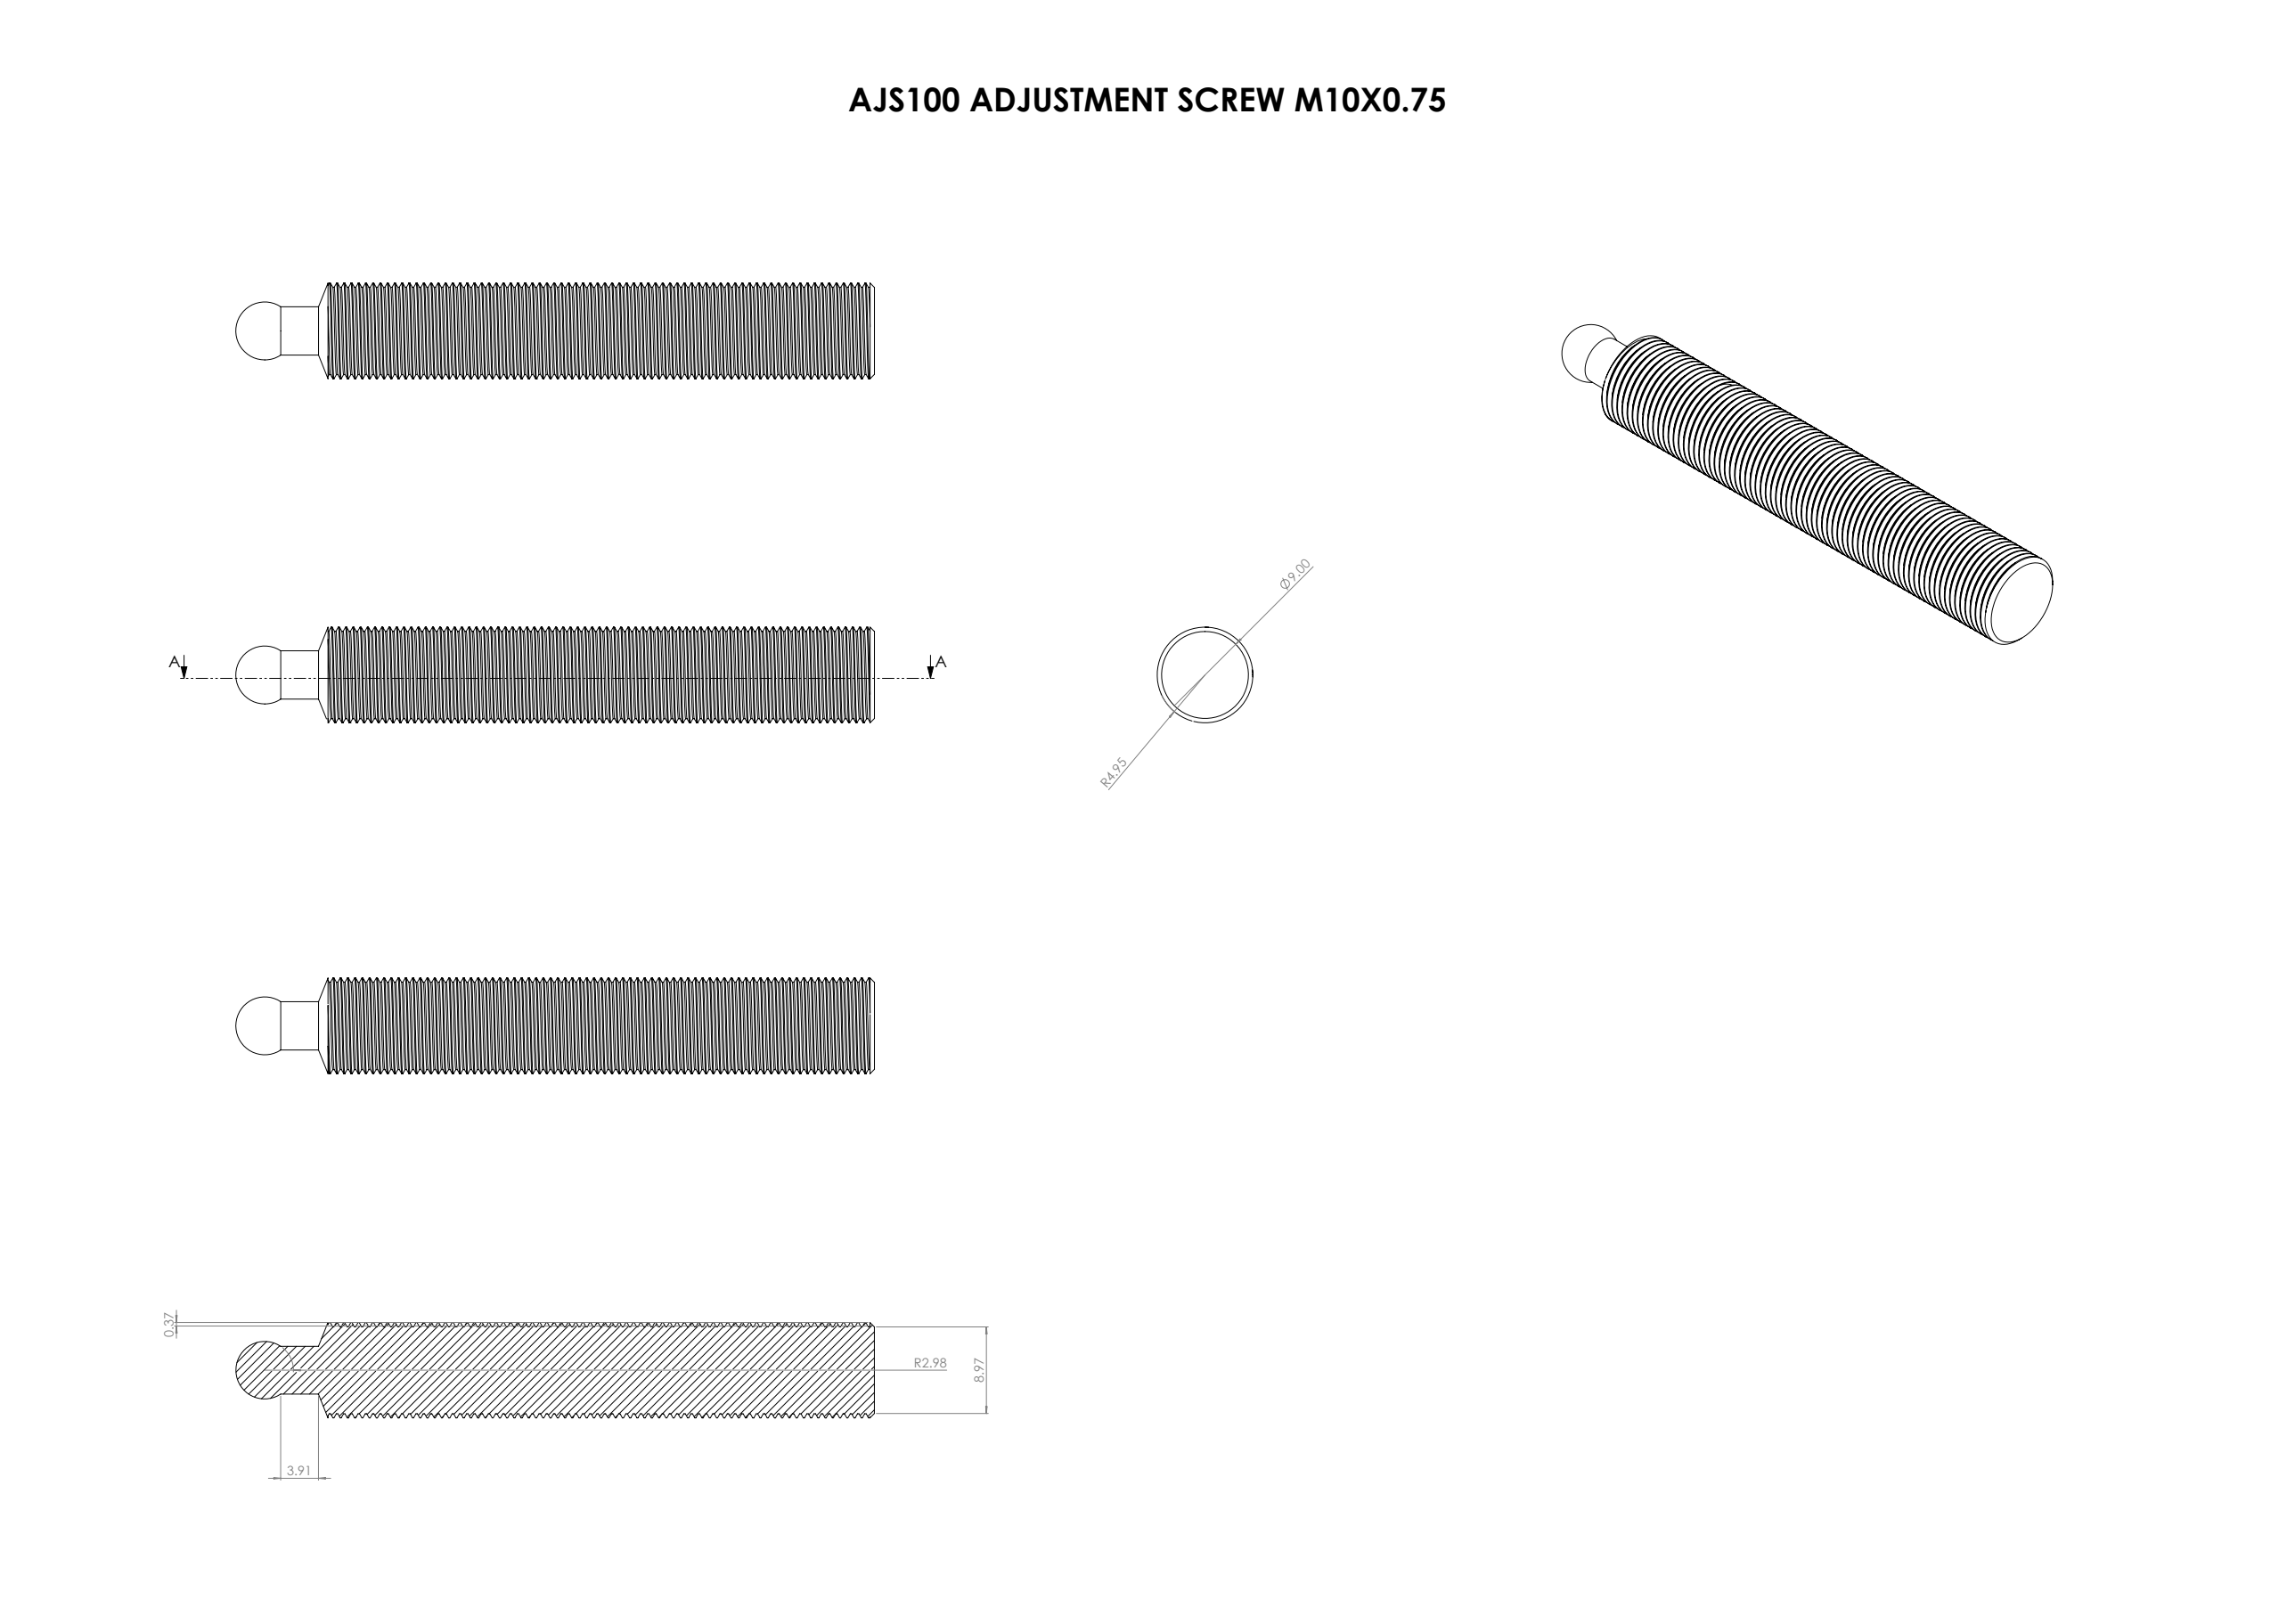
ISO-10303-21;
HEADER;
/* Generated by software containing ST-Developer
 * from STEP Tools, Inc. (www.steptools.com) 
 */

FILE_DESCRIPTION(
/* description */ (''),
/* implementation_level */ '2;1');

FILE_NAME(
/* name */ '05_AJS100_Adjustment_Screw_M10x0.75.step',
/* time_stamp */ '2026-10-21T01:56:51-07:00',
/* author */ (''),
/* organization */ (''),
/* preprocessor_version */ 'ST-DEVELOPER v20.2',
/* originating_system */ 'Autodesk Translation Framework v15.15.0.0',
/* authorisation */ '');

FILE_SCHEMA (('AUTOMOTIVE_DESIGN { 1 0 10303 214 3 1 1 }'));
ENDSEC;

DATA;
#10=MECHANICAL_DESIGN_GEOMETRIC_PRESENTATION_REPRESENTATION('',(#286),#82384);
#156=SPHERICAL_SURFACE('',#33152,3.00000000000001);
#248=SHAPE_REPRESENTATION_RELATIONSHIP('SRR','None',#82482,#267);
#267=ADVANCED_BREP_SHAPE_REPRESENTATION('',(#305),#82381);
#286=STYLED_ITEM('',(#82638),#305);
#305=MANIFOLD_SOLID_BREP('Body1',#30677);
#429=B_SPLINE_SURFACE_WITH_KNOTS('',3,3,((#76147,#76148,#76149,#76150,#76151,
#76152,#76153,#76154,#76155,#76156,#76157,#76158,#76159,#76160,#76161,#76162,
#76163,#76164,#76165,#76166,#76167,#76168,#76169,#76170,#76171,#76172,#76173,
#76174,#76175,#76176,#76177,#76178,#76179,#76180,#76181,#76182,#76183,#76184,
#76185,#76186,#76187,#76188,#76189,#76190,#76191,#76192,#76193,#76194,#76195,
#76196,#76197,#76198,#76199,#76200,#76201,#76202,#76203,#76204,#76205,#76206,
#76207,#76208,#76209,#76210,#76211,#76212,#76213,#76214,#76215,#76216,#76217,
#76218,#76219,#76220,#76221,#76222,#76223,#76224,#76225,#76226,#76227,#76228,
#76229,#76230,#76231,#76232,#76233,#76234,#76235,#76236,#76237,#76238,#76239,
#76240,#76241,#76242,#76243,#76244,#76245,#76246,#76247,#76248,#76249,#76250,
#76251,#76252,#76253,#76254,#76255,#76256,#76257,#76258,#76259,#76260,#76261,
#76262,#76263,#76264,#76265,#76266,#76267,#76268,#76269,#76270,#76271,#76272,
#76273,#76274,#76275,#76276,#76277,#76278,#76279,#76280,#76281,#76282,#76283,
#76284,#76285,#76286,#76287,#76288,#76289,#76290,#76291,#76292,#76293,#76294,
#76295,#76296,#76297,#76298,#76299,#76300,#76301,#76302,#76303,#76304,#76305,
#76306,#76307,#76308,#76309,#76310,#76311,#76312,#76313,#76314,#76315,#76316,
#76317,#76318,#76319,#76320,#76321,#76322,#76323,#76324,#76325,#76326,#76327,
#76328,#76329,#76330,#76331,#76332,#76333,#76334,#76335,#76336,#76337,#76338,
#76339,#76340,#76341,#76342,#76343,#76344,#76345,#76346,#76347,#76348,#76349,
#76350,#76351,#76352,#76353,#76354,#76355,#76356,#76357,#76358,#76359,#76360,
#76361,#76362,#76363,#76364,#76365,#76366,#76367,#76368,#76369,#76370,#76371,
#76372,#76373,#76374,#76375,#76376,#76377,#76378,#76379,#76380,#76381,#76382,
#76383,#76384,#76385,#76386,#76387,#76388,#76389,#76390,#76391,#76392,#76393,
#76394,#76395,#76396,#76397,#76398,#76399,#76400,#76401,#76402,#76403,#76404,
#76405,#76406,#76407,#76408,#76409,#76410,#76411,#76412,#76413,#76414,#76415,
#76416,#76417,#76418,#76419,#76420,#76421,#76422,#76423,#76424,#76425,#76426,
#76427,#76428,#76429,#76430,#76431,#76432,#76433,#76434,#76435,#76436,#76437,
#76438,#76439,#76440,#76441,#76442,#76443,#76444,#76445,#76446,#76447,#76448,
#76449,#76450,#76451,#76452,#76453,#76454,#76455,#76456,#76457,#76458,#76459,
#76460,#76461,#76462,#76463,#76464,#76465,#76466,#76467,#76468,#76469,#76470,
#76471,#76472,#76473,#76474,#76475,#76476,#76477,#76478,#76479,#76480,#76481,
#76482,#76483,#76484,#76485,#76486,#76487,#76488,#76489,#76490,#76491,#76492,
#76493,#76494,#76495,#76496,#76497,#76498,#76499,#76500,#76501,#76502,#76503,
#76504,#76505,#76506,#76507,#76508,#76509,#76510,#76511,#76512,#76513,#76514,
#76515,#76516,#76517,#76518,#76519,#76520,#76521,#76522,#76523,#76524,#76525,
#76526,#76527,#76528,#76529,#76530,#76531,#76532,#76533,#76534,#76535,#76536,
#76537,#76538,#76539,#76540,#76541,#76542,#76543,#76544,#76545,#76546,#76547,
#76548,#76549,#76550,#76551,#76552,#76553,#76554,#76555,#76556,#76557,#76558,
#76559,#76560,#76561,#76562,#76563,#76564,#76565,#76566,#76567,#76568,#76569,
#76570,#76571,#76572,#76573,#76574,#76575,#76576,#76577,#76578,#76579,#76580,
#76581,#76582,#76583,#76584,#76585,#76586,#76587,#76588,#76589,#76590,#76591,
#76592,#76593,#76594,#76595,#76596,#76597,#76598,#76599,#76600,#76601,#76602,
#76603,#76604,#76605,#76606,#76607,#76608,#76609,#76610,#76611,#76612,#76613,
#76614,#76615,#76616,#76617,#76618,#76619,#76620,#76621,#76622,#76623,#76624),
(#76625,#76626,#76627,#76628,#76629,#76630,#76631,#76632,#76633,#76634,
#76635,#76636,#76637,#76638,#76639,#76640,#76641,#76642,#76643,#76644,#76645,
#76646,#76647,#76648,#76649,#76650,#76651,#76652,#76653,#76654,#76655,#76656,
#76657,#76658,#76659,#76660,#76661,#76662,#76663,#76664,#76665,#76666,#76667,
#76668,#76669,#76670,#76671,#76672,#76673,#76674,#76675,#76676,#76677,#76678,
#76679,#76680,#76681,#76682,#76683,#76684,#76685,#76686,#76687,#76688,#76689,
#76690,#76691,#76692,#76693,#76694,#76695,#76696,#76697,#76698,#76699,#76700,
#76701,#76702,#76703,#76704,#76705,#76706,#76707,#76708,#76709,#76710,#76711,
#76712,#76713,#76714,#76715,#76716,#76717,#76718,#76719,#76720,#76721,#76722,
#76723,#76724,#76725,#76726,#76727,#76728,#76729,#76730,#76731,#76732,#76733,
#76734,#76735,#76736,#76737,#76738,#76739,#76740,#76741,#76742,#76743,#76744,
#76745,#76746,#76747,#76748,#76749,#76750,#76751,#76752,#76753,#76754,#76755,
#76756,#76757,#76758,#76759,#76760,#76761,#76762,#76763,#76764,#76765,#76766,
#76767,#76768,#76769,#76770,#76771,#76772,#76773,#76774,#76775,#76776,#76777,
#76778,#76779,#76780,#76781,#76782,#76783,#76784,#76785,#76786,#76787,#76788,
#76789,#76790,#76791,#76792,#76793,#76794,#76795,#76796,#76797,#76798,#76799,
#76800,#76801,#76802,#76803,#76804,#76805,#76806,#76807,#76808,#76809,#76810,
#76811,#76812,#76813,#76814,#76815,#76816,#76817,#76818,#76819,#76820,#76821,
#76822,#76823,#76824,#76825,#76826,#76827,#76828,#76829,#76830,#76831,#76832,
#76833,#76834,#76835,#76836,#76837,#76838,#76839,#76840,#76841,#76842,#76843,
#76844,#76845,#76846,#76847,#76848,#76849,#76850,#76851,#76852,#76853,#76854,
#76855,#76856,#76857,#76858,#76859,#76860,#76861,#76862,#76863,#76864,#76865,
#76866,#76867,#76868,#76869,#76870,#76871,#76872,#76873,#76874,#76875,#76876,
#76877,#76878,#76879,#76880,#76881,#76882,#76883,#76884,#76885,#76886,#76887,
#76888,#76889,#76890,#76891,#76892,#76893,#76894,#76895,#76896,#76897,#76898,
#76899,#76900,#76901,#76902,#76903,#76904,#76905,#76906,#76907,#76908,#76909,
#76910,#76911,#76912,#76913,#76914,#76915,#76916,#76917,#76918,#76919,#76920,
#76921,#76922,#76923,#76924,#76925,#76926,#76927,#76928,#76929,#76930,#76931,
#76932,#76933,#76934,#76935,#76936,#76937,#76938,#76939,#76940,#76941,#76942,
#76943,#76944,#76945,#76946,#76947,#76948,#76949,#76950,#76951,#76952,#76953,
#76954,#76955,#76956,#76957,#76958,#76959,#76960,#76961,#76962,#76963,#76964,
#76965,#76966,#76967,#76968,#76969,#76970,#76971,#76972,#76973,#76974,#76975,
#76976,#76977,#76978,#76979,#76980,#76981,#76982,#76983,#76984,#76985,#76986,
#76987,#76988,#76989,#76990,#76991,#76992,#76993,#76994,#76995,#76996,#76997,
#76998,#76999,#77000,#77001,#77002,#77003,#77004,#77005,#77006,#77007,#77008,
#77009,#77010,#77011,#77012,#77013,#77014,#77015,#77016,#77017,#77018,#77019,
#77020,#77021,#77022,#77023,#77024,#77025,#77026,#77027,#77028,#77029,#77030,
#77031,#77032,#77033,#77034,#77035,#77036,#77037,#77038,#77039,#77040,#77041,
#77042,#77043,#77044,#77045,#77046,#77047,#77048,#77049,#77050,#77051,#77052,
#77053,#77054,#77055,#77056,#77057,#77058,#77059,#77060,#77061,#77062,#77063,
#77064,#77065,#77066,#77067,#77068,#77069,#77070,#77071,#77072,#77073,#77074,
#77075,#77076,#77077,#77078,#77079,#77080,#77081,#77082,#77083,#77084,#77085,
#77086,#77087,#77088,#77089,#77090,#77091,#77092,#77093,#77094,#77095,#77096,
#77097,#77098,#77099,#77100,#77101,#77102),(#77103,#77104,#77105,#77106,
#77107,#77108,#77109,#77110,#77111,#77112,#77113,#77114,#77115,#77116,#77117,
#77118,#77119,#77120,#77121,#77122,#77123,#77124,#77125,#77126,#77127,#77128,
#77129,#77130,#77131,#77132,#77133,#77134,#77135,#77136,#77137,#77138,#77139,
#77140,#77141,#77142,#77143,#77144,#77145,#77146,#77147,#77148,#77149,#77150,
#77151,#77152,#77153,#77154,#77155,#77156,#77157,#77158,#77159,#77160,#77161,
#77162,#77163,#77164,#77165,#77166,#77167,#77168,#77169,#77170,#77171,#77172,
#77173,#77174,#77175,#77176,#77177,#77178,#77179,#77180,#77181,#77182,#77183,
#77184,#77185,#77186,#77187,#77188,#77189,#77190,#77191,#77192,#77193,#77194,
#77195,#77196,#77197,#77198,#77199,#77200,#77201,#77202,#77203,#77204,#77205,
#77206,#77207,#77208,#77209,#77210,#77211,#77212,#77213,#77214,#77215,#77216,
#77217,#77218,#77219,#77220,#77221,#77222,#77223,#77224,#77225,#77226,#77227,
#77228,#77229,#77230,#77231,#77232,#77233,#77234,#77235,#77236,#77237,#77238,
#77239,#77240,#77241,#77242,#77243,#77244,#77245,#77246,#77247,#77248,#77249,
#77250,#77251,#77252,#77253,#77254,#77255,#77256,#77257,#77258,#77259,#77260,
#77261,#77262,#77263,#77264,#77265,#77266,#77267,#77268,#77269,#77270,#77271,
#77272,#77273,#77274,#77275,#77276,#77277,#77278,#77279,#77280,#77281,#77282,
#77283,#77284,#77285,#77286,#77287,#77288,#77289,#77290,#77291,#77292,#77293,
#77294,#77295,#77296,#77297,#77298,#77299,#77300,#77301,#77302,#77303,#77304,
#77305,#77306,#77307,#77308,#77309,#77310,#77311,#77312,#77313,#77314,#77315,
#77316,#77317,#77318,#77319,#77320,#77321,#77322,#77323,#77324,#77325,#77326,
#77327,#77328,#77329,#77330,#77331,#77332,#77333,#77334,#77335,#77336,#77337,
#77338,#77339,#77340,#77341,#77342,#77343,#77344,#77345,#77346,#77347,#77348,
#77349,#77350,#77351,#77352,#77353,#77354,#77355,#77356,#77357,#77358,#77359,
#77360,#77361,#77362,#77363,#77364,#77365,#77366,#77367,#77368,#77369,#77370,
#77371,#77372,#77373,#77374,#77375,#77376,#77377,#77378,#77379,#77380,#77381,
#77382,#77383,#77384,#77385,#77386,#77387,#77388,#77389,#77390,#77391,#77392,
#77393,#77394,#77395,#77396,#77397,#77398,#77399,#77400,#77401,#77402,#77403,
#77404,#77405,#77406,#77407,#77408,#77409,#77410,#77411,#77412,#77413,#77414,
#77415,#77416,#77417,#77418,#77419,#77420,#77421,#77422,#77423,#77424,#77425,
#77426,#77427,#77428,#77429,#77430,#77431,#77432,#77433,#77434,#77435,#77436,
#77437,#77438,#77439,#77440,#77441,#77442,#77443,#77444,#77445,#77446,#77447,
#77448,#77449,#77450,#77451,#77452,#77453,#77454,#77455,#77456,#77457,#77458,
#77459,#77460,#77461,#77462,#77463,#77464,#77465,#77466,#77467,#77468,#77469,
#77470,#77471,#77472,#77473,#77474,#77475,#77476,#77477,#77478,#77479,#77480,
#77481,#77482,#77483,#77484,#77485,#77486,#77487,#77488,#77489,#77490,#77491,
#77492,#77493,#77494,#77495,#77496,#77497,#77498,#77499,#77500,#77501,#77502,
#77503,#77504,#77505,#77506,#77507,#77508,#77509,#77510,#77511,#77512,#77513,
#77514,#77515,#77516,#77517,#77518,#77519,#77520,#77521,#77522,#77523,#77524,
#77525,#77526,#77527,#77528,#77529,#77530,#77531,#77532,#77533,#77534,#77535,
#77536,#77537,#77538,#77539,#77540,#77541,#77542,#77543,#77544,#77545,#77546,
#77547,#77548,#77549,#77550,#77551,#77552,#77553,#77554,#77555,#77556,#77557,
#77558,#77559,#77560,#77561,#77562,#77563,#77564,#77565,#77566,#77567,#77568,
#77569,#77570,#77571,#77572,#77573,#77574,#77575,#77576,#77577,#77578,#77579,
#77580),(#77581,#77582,#77583,#77584,#77585,#77586,#77587,#77588,#77589,
#77590,#77591,#77592,#77593,#77594,#77595,#77596,#77597,#77598,#77599,#77600,
#77601,#77602,#77603,#77604,#77605,#77606,#77607,#77608,#77609,#77610,#77611,
#77612,#77613,#77614,#77615,#77616,#77617,#77618,#77619,#77620,#77621,#77622,
#77623,#77624,#77625,#77626,#77627,#77628,#77629,#77630,#77631,#77632,#77633,
#77634,#77635,#77636,#77637,#77638,#77639,#77640,#77641,#77642,#77643,#77644,
#77645,#77646,#77647,#77648,#77649,#77650,#77651,#77652,#77653,#77654,#77655,
#77656,#77657,#77658,#77659,#77660,#77661,#77662,#77663,#77664,#77665,#77666,
#77667,#77668,#77669,#77670,#77671,#77672,#77673,#77674,#77675,#77676,#77677,
#77678,#77679,#77680,#77681,#77682,#77683,#77684,#77685,#77686,#77687,#77688,
#77689,#77690,#77691,#77692,#77693,#77694,#77695,#77696,#77697,#77698,#77699,
#77700,#77701,#77702,#77703,#77704,#77705,#77706,#77707,#77708,#77709,#77710,
#77711,#77712,#77713,#77714,#77715,#77716,#77717,#77718,#77719,#77720,#77721,
#77722,#77723,#77724,#77725,#77726,#77727,#77728,#77729,#77730,#77731,#77732,
#77733,#77734,#77735,#77736,#77737,#77738,#77739,#77740,#77741,#77742,#77743,
#77744,#77745,#77746,#77747,#77748,#77749,#77750,#77751,#77752,#77753,#77754,
#77755,#77756,#77757,#77758,#77759,#77760,#77761,#77762,#77763,#77764,#77765,
#77766,#77767,#77768,#77769,#77770,#77771,#77772,#77773,#77774,#77775,#77776,
#77777,#77778,#77779,#77780,#77781,#77782,#77783,#77784,#77785,#77786,#77787,
#77788,#77789,#77790,#77791,#77792,#77793,#77794,#77795,#77796,#77797,#77798,
#77799,#77800,#77801,#77802,#77803,#77804,#77805,#77806,#77807,#77808,#77809,
#77810,#77811,#77812,#77813,#77814,#77815,#77816,#77817,#77818,#77819,#77820,
#77821,#77822,#77823,#77824,#77825,#77826,#77827,#77828,#77829,#77830,#77831,
#77832,#77833,#77834,#77835,#77836,#77837,#77838,#77839,#77840,#77841,#77842,
#77843,#77844,#77845,#77846,#77847,#77848,#77849,#77850,#77851,#77852,#77853,
#77854,#77855,#77856,#77857,#77858,#77859,#77860,#77861,#77862,#77863,#77864,
#77865,#77866,#77867,#77868,#77869,#77870,#77871,#77872,#77873,#77874,#77875,
#77876,#77877,#77878,#77879,#77880,#77881,#77882,#77883,#77884,#77885,#77886,
#77887,#77888,#77889,#77890,#77891,#77892,#77893,#77894,#77895,#77896,#77897,
#77898,#77899,#77900,#77901,#77902,#77903,#77904,#77905,#77906,#77907,#77908,
#77909,#77910,#77911,#77912,#77913,#77914,#77915,#77916,#77917,#77918,#77919,
#77920,#77921,#77922,#77923,#77924,#77925,#77926,#77927,#77928,#77929,#77930,
#77931,#77932,#77933,#77934,#77935,#77936,#77937,#77938,#77939,#77940,#77941,
#77942,#77943,#77944,#77945,#77946,#77947,#77948,#77949,#77950,#77951,#77952,
#77953,#77954,#77955,#77956,#77957,#77958,#77959,#77960,#77961,#77962,#77963,
#77964,#77965,#77966,#77967,#77968,#77969,#77970,#77971,#77972,#77973,#77974,
#77975,#77976,#77977,#77978,#77979,#77980,#77981,#77982,#77983,#77984,#77985,
#77986,#77987,#77988,#77989,#77990,#77991,#77992,#77993,#77994,#77995,#77996,
#77997,#77998,#77999,#78000,#78001,#78002,#78003,#78004,#78005,#78006,#78007,
#78008,#78009,#78010,#78011,#78012,#78013,#78014,#78015,#78016,#78017,#78018,
#78019,#78020,#78021,#78022,#78023,#78024,#78025,#78026,#78027,#78028,#78029,
#78030,#78031,#78032,#78033,#78034,#78035,#78036,#78037,#78038,#78039,#78040,
#78041,#78042,#78043,#78044,#78045,#78046,#78047,#78048,#78049,#78050,#78051,
#78052,#78053,#78054,#78055,#78056,#78057,#78058)),.UNSPECIFIED.,.F.,.F.,
 .F.,(4,4),(4,1,1,1,1,1,1,1,1,1,1,1,1,1,1,1,1,1,1,1,1,1,1,1,1,1,1,1,1,1,
1,1,1,1,1,1,1,1,1,1,1,1,1,1,1,1,1,1,1,1,1,1,1,1,1,1,1,1,1,1,1,1,1,1,1,1,
1,1,1,1,1,1,1,1,1,1,1,1,1,1,1,1,1,1,1,1,1,1,1,1,1,1,1,1,1,1,1,1,1,1,1,1,
1,1,1,1,1,1,1,1,1,1,1,1,1,1,1,1,1,1,1,1,1,1,1,1,1,1,1,1,1,1,1,1,1,1,1,1,
1,1,1,1,1,1,1,1,1,1,1,1,1,1,1,1,1,1,1,1,1,1,1,1,1,1,1,1,1,1,1,1,1,1,1,1,
1,1,1,1,1,1,1,1,1,1,1,1,1,1,1,1,1,1,1,1,1,1,1,1,1,1,1,1,1,1,1,1,1,1,1,1,
1,1,1,1,1,1,1,1,1,1,1,1,1,1,1,1,1,1,1,1,1,1,1,1,1,1,1,1,1,1,1,1,1,1,1,1,
1,1,1,1,1,1,1,1,1,1,1,1,1,1,1,1,1,1,1,1,1,1,1,1,1,1,1,1,1,1,1,1,1,1,1,1,
1,1,1,1,1,1,1,1,1,1,1,1,1,1,1,1,1,1,1,1,1,1,1,1,1,1,1,1,1,1,1,1,1,1,1,1,
1,1,1,1,1,1,1,1,1,1,1,1,1,1,1,1,1,1,1,1,1,1,1,1,1,1,1,1,1,1,1,1,1,1,1,1,
1,1,1,1,1,1,1,1,1,1,1,1,1,1,1,1,1,1,1,1,1,1,1,1,1,1,1,1,1,1,1,1,1,1,1,1,
1,1,1,1,1,1,1,1,1,1,1,1,1,1,1,1,1,1,1,1,1,1,1,1,1,1,1,1,1,1,1,1,1,1,1,1,
1,1,1,1,1,1,1,1,1,1,1,1,1,1,1,1,1,1,1,1,1,1,1,1,1,1,1,1,1,1,1,1,1,1,1,1,
1,1,1,1,1,1,1,1,1,1,1,1,1,4),(0.,0.0496809906637672),(8.29538555664048,
8.79496569366582,9.29454583069116,10.2937061047418,11.2928663787925,12.2920266528432,
13.2911869268939,14.2903472009446,15.2895074749953,16.288667749046,17.2878280230966,
18.2869882971473,19.286148571198,20.2853088452487,21.2844691192994,22.2836293933501,
23.2827896674008,24.2819499414514,25.2811102155021,26.2802704895528,27.2794307636035,
28.2785910376542,29.2777513117049,30.2769115857556,31.2760718598062,32.2752321338569,
33.2743924079076,34.2735526819583,35.272712956009,36.2718732300597,37.2710335041103,
38.270193778161,39.2693540522117,40.2685143262624,41.2676746003131,42.2668348743638,
43.2659951484145,44.2651554224651,45.2643156965158,46.2634759705665,47.2626362446172,
48.2617965186679,49.2609567927186,50.2601170667693,51.2592773408199,52.2584376148706,
53.2575978889213,54.256758162972,55.2559184370227,56.2550787110734,57.2542389851241,
58.2533992591747,59.2525595332254,60.2517198072761,61.2508800813268,62.2500403553775,
63.2492006294282,64.2483609034789,65.2475211775295,66.2466814515802,67.2458417256309,
68.2450019996816,69.2441622737323,70.243322547783,71.2424828218336,72.2416430958843,
73.240803369935,74.2399636439857,75.2391239180364,76.2382841920871,77.2374444661378,
78.2366047401885,79.2357650142391,80.2349252882898,81.2340855623405,82.2332458363912,
83.2324061104419,84.2315663844926,85.2307266585432,86.2298869325939,87.2290472066446,
88.2282074806953,89.227367754746,90.2265280287967,91.2256883028474,92.2248485768981,
93.2240088509487,94.2231691249994,95.2223293990501,96.2214896731008,97.2206499471515,
98.2198102212022,99.2189704952528,100.218130769304,101.217291043354,102.216451317405,
103.215611591456,104.214771865506,105.213932139557,106.213092413608,107.212252687658,
108.211412961709,109.21057323576,110.20973350981,111.208893783861,112.208054057912,
113.207214331962,114.206374606013,115.205534880064,116.204695154114,117.203855428165,
118.203015702216,119.202175976267,120.201336250317,121.200496524368,122.199656798419,
123.198817072469,124.19797734652,125.197137620571,126.196297894621,127.195458168672,
128.194618442723,129.193778716773,130.192938990824,131.192099264875,132.191259538925,
133.190419812976,134.189580087027,135.188740361078,136.187900635128,137.187060909179,
138.18622118323,139.18538145728,140.184541731331,141.183702005382,142.182862279432,
143.182022553483,144.181182827534,145.180343101584,146.179503375635,147.178663649686,
148.177823923736,149.176984197787,150.176144471838,151.175304745888,152.174465019939,
153.17362529399,154.172785568041,155.171945842091,156.171106116142,157.170266390193,
158.169426664243,159.168586938294,160.167747212345,161.166907486395,162.166067760446,
163.165228034497,164.164388308547,165.163548582598,166.162708856649,167.161869130699,
168.16102940475,169.160189678801,170.159349952851,171.158510226902,172.157670500953,
173.156830775004,174.155991049054,175.155151323105,176.154311597156,177.153471871206,
178.152632145257,179.151792419308,180.150952693358,181.150112967409,182.14927324146,
183.14843351551,184.147593789561,185.146754063612,186.145914337662,187.145074611713,
188.144234885764,189.143395159815,190.142555433865,191.141715707916,192.140875981967,
193.140036256017,194.139196530068,195.138356804119,196.137517078169,197.13667735222,
198.135837626271,199.134997900321,200.134158174372,201.133318448423,202.132478722473,
203.131638996524,204.130799270575,205.129959544625,206.129119818676,207.128280092727,
208.127440366778,209.126600640828,210.125760914879,211.12492118893,212.12408146298,
213.123241737031,214.122402011082,215.121562285132,216.120722559183,217.119882833234,
218.119043107284,219.118203381335,220.117363655386,221.116523929436,222.115684203487,
223.114844477538,224.114004751588,225.113165025639,226.11232529969,227.111485573741,
228.110645847791,229.109806121842,230.108966395893,231.108126669943,232.107286943994,
233.106447218045,234.105607492095,235.104767766146,236.103928040197,237.103088314247,
238.102248588298,239.101408862349,240.100569136399,241.09972941045,242.098889684501,
243.098049958552,244.097210232602,245.096370506653,246.095530780704,247.094691054754,
248.093851328805,249.093011602856,250.092171876906,251.091332150957,252.090492425008,
253.089652699058,254.088812973109,255.08797324716,256.08713352121,257.086293795261,
258.085454069312,259.084614343362,260.083774617413,261.082934891464,262.082095165515,
263.081255439565,264.080415713616,265.079575987667,266.078736261717,267.077896535768,
268.077056809819,269.076217083869,270.07537735792,271.074537631971,272.073697906021,
273.072858180072,274.072018454123,275.071178728173,276.070339002224,277.069499276275,
278.068659550326,279.067819824376,280.066980098427,281.066140372478,282.065300646528,
283.064460920579,284.06362119463,285.06278146868,286.061941742731,287.061102016782,
288.060262290832,289.059422564883,290.058582838934,291.057743112984,292.056903387035,
293.056063661086,294.055223935136,295.054384209187,296.053544483238,297.052704757289,
298.051865031339,299.05102530539,300.050185579441,301.049345853491,302.048506127542,
303.047666401593,304.046826675643,305.045986949694,306.045147223745,307.044307497795,
308.043467771846,309.042628045897,310.041788319947,311.040948593998,312.040108868049,
313.039269142099,314.03842941615,315.037589690201,316.036749964252,317.035910238302,
318.035070512353,319.034230786404,320.033391060454,321.032551334505,322.031711608556,
323.030871882606,324.030032156657,325.029192430708,326.028352704758,327.027512978809,
328.02667325286,329.025833526911,330.024993800961,331.024154075012,332.023314349063,
333.022474623113,334.021634897164,335.020795171215,336.019955445265,337.019115719316,
338.018275993367,339.017436267417,340.016596541468,341.015756815519,342.014917089569,
343.01407736362,344.013237637671,345.012397911721,346.011558185772,347.010718459823,
348.009878733874,349.009039007924,350.008199281975,351.007359556026,352.006519830076,
353.005680104127,354.004840378178,355.004000652228,356.003160926279,357.00232120033,
358.00148147438,359.000641748431,359.999802022482,360.998962296532,361.998122570583,
362.997282844634,363.996443118684,364.995603392735,365.994763666786,366.993923940837,
367.993084214887,368.992244488938,369.991404762989,370.990565037039,371.98972531109,
372.988885585141,373.988045859191,374.987206133242,375.986366407293,376.985526681343,
377.984686955394,378.983847229445,379.983007503495,380.982167777546,381.981328051597,
382.980488325648,383.979648599698,384.978808873749,385.9779691478,386.97712942185,
387.976289695901,388.975449969952,389.974610244002,390.973770518053,391.972930792104,
392.972091066154,393.971251340205,394.970411614256,395.969571888306,396.968732162357,
397.967892436408,398.967052710458,399.966212984509,400.96537325856,401.964533532611,
402.963693806661,403.962854080712,404.962014354763,405.961174628813,406.960334902864,
407.959495176915,408.958655450965,409.957815725016,410.956975999067,411.956136273117,
412.955296547168,413.954456821219,414.953617095269,415.95277736932,416.951937643371,
417.951097917421,418.950258191472,419.949418465523,420.948578739574,421.947739013624,
422.946899287675,423.946059561726,424.945219835776,425.944380109827,426.943540383878,
427.942700657928,428.941860931979,429.94102120603,430.94018148008,431.939341754131,
432.938502028182,433.937662302232,434.936822576283,435.935982850334,436.935143124384,
437.934303398435,438.933463672486,439.932623946537,440.931784220587,441.930944494638,
442.930104768689,443.929265042739,444.92842531679,445.927585590841,446.926745864891,
447.925906138942,448.925066412993,449.924226687043,450.923386961094,451.922547235145,
452.921707509195,453.920867783246,454.920028057297,455.919188331348,456.918348605398,
457.917508879449,458.9166691535,459.91582942755,460.914989701601,461.914149975652,
462.913310249702,463.912470523753,464.911630797804,465.910791071854,466.909951345905,
467.909111619956,468.908271894006,469.907432168057,470.906592442108,471.905752716158,
472.904912990209,473.90407326426,474.903233538311,475.902393812361,476.901554086412,
477.900714360463,478.899874634513,479.899034908564,480.398615045589,480.898195182615),
 .UNSPECIFIED.);
#430=B_SPLINE_SURFACE_WITH_KNOTS('',3,3,((#78316,#78317,#78318,#78319,#78320,
#78321,#78322,#78323,#78324,#78325,#78326,#78327,#78328,#78329,#78330,#78331,
#78332,#78333,#78334,#78335,#78336,#78337,#78338,#78339,#78340,#78341,#78342,
#78343,#78344,#78345,#78346,#78347,#78348,#78349,#78350,#78351,#78352,#78353,
#78354,#78355,#78356,#78357,#78358,#78359,#78360,#78361,#78362,#78363,#78364,
#78365,#78366,#78367,#78368,#78369,#78370,#78371,#78372,#78373,#78374,#78375,
#78376,#78377,#78378,#78379,#78380,#78381,#78382,#78383,#78384,#78385,#78386,
#78387,#78388,#78389,#78390,#78391,#78392,#78393,#78394,#78395,#78396,#78397,
#78398,#78399,#78400,#78401,#78402,#78403,#78404,#78405,#78406,#78407,#78408,
#78409,#78410,#78411,#78412,#78413,#78414,#78415,#78416,#78417,#78418,#78419,
#78420,#78421,#78422,#78423,#78424,#78425,#78426,#78427,#78428,#78429,#78430,
#78431,#78432,#78433,#78434,#78435,#78436,#78437,#78438,#78439,#78440,#78441,
#78442,#78443,#78444,#78445,#78446,#78447,#78448,#78449,#78450,#78451,#78452,
#78453,#78454,#78455,#78456,#78457,#78458,#78459,#78460,#78461,#78462,#78463,
#78464,#78465,#78466,#78467,#78468,#78469,#78470,#78471,#78472,#78473,#78474,
#78475,#78476,#78477,#78478,#78479,#78480,#78481,#78482,#78483,#78484,#78485,
#78486,#78487,#78488,#78489,#78490,#78491,#78492,#78493,#78494,#78495,#78496,
#78497,#78498,#78499,#78500,#78501,#78502,#78503,#78504,#78505,#78506,#78507,
#78508,#78509,#78510,#78511,#78512,#78513,#78514,#78515,#78516,#78517,#78518,
#78519,#78520,#78521,#78522,#78523,#78524,#78525,#78526,#78527,#78528,#78529,
#78530,#78531,#78532,#78533,#78534,#78535,#78536,#78537,#78538,#78539,#78540,
#78541,#78542,#78543,#78544,#78545,#78546,#78547,#78548,#78549,#78550,#78551,
#78552,#78553,#78554,#78555,#78556,#78557,#78558,#78559,#78560,#78561,#78562,
#78563,#78564,#78565,#78566,#78567,#78568,#78569,#78570,#78571,#78572,#78573,
#78574,#78575,#78576,#78577,#78578,#78579,#78580,#78581,#78582,#78583,#78584,
#78585,#78586,#78587,#78588,#78589,#78590,#78591,#78592,#78593,#78594,#78595,
#78596,#78597,#78598,#78599,#78600,#78601,#78602,#78603,#78604,#78605,#78606,
#78607,#78608,#78609,#78610,#78611,#78612,#78613,#78614,#78615,#78616,#78617,
#78618,#78619,#78620,#78621,#78622,#78623,#78624,#78625,#78626,#78627,#78628,
#78629,#78630,#78631,#78632,#78633,#78634,#78635,#78636,#78637,#78638,#78639,
#78640,#78641,#78642,#78643,#78644,#78645,#78646,#78647,#78648,#78649,#78650,
#78651,#78652,#78653,#78654,#78655,#78656,#78657,#78658,#78659,#78660,#78661,
#78662,#78663,#78664,#78665,#78666,#78667,#78668,#78669,#78670,#78671,#78672,
#78673,#78674,#78675,#78676,#78677,#78678,#78679,#78680,#78681,#78682,#78683,
#78684,#78685,#78686,#78687,#78688,#78689,#78690,#78691,#78692,#78693,#78694,
#78695,#78696,#78697,#78698,#78699,#78700,#78701,#78702,#78703,#78704,#78705,
#78706,#78707,#78708,#78709,#78710,#78711,#78712,#78713,#78714,#78715,#78716,
#78717,#78718,#78719,#78720,#78721,#78722,#78723,#78724,#78725,#78726,#78727,
#78728,#78729,#78730,#78731,#78732,#78733,#78734,#78735,#78736,#78737,#78738,
#78739,#78740,#78741,#78742,#78743,#78744,#78745,#78746,#78747,#78748,#78749,
#78750,#78751,#78752,#78753,#78754,#78755,#78756,#78757,#78758,#78759,#78760,
#78761,#78762,#78763,#78764,#78765,#78766,#78767,#78768,#78769,#78770,#78771,
#78772,#78773,#78774,#78775,#78776,#78777,#78778,#78779,#78780,#78781,#78782,
#78783,#78784,#78785,#78786,#78787,#78788,#78789,#78790,#78791,#78792,#78793),
(#78794,#78795,#78796,#78797,#78798,#78799,#78800,#78801,#78802,#78803,
#78804,#78805,#78806,#78807,#78808,#78809,#78810,#78811,#78812,#78813,#78814,
#78815,#78816,#78817,#78818,#78819,#78820,#78821,#78822,#78823,#78824,#78825,
#78826,#78827,#78828,#78829,#78830,#78831,#78832,#78833,#78834,#78835,#78836,
#78837,#78838,#78839,#78840,#78841,#78842,#78843,#78844,#78845,#78846,#78847,
#78848,#78849,#78850,#78851,#78852,#78853,#78854,#78855,#78856,#78857,#78858,
#78859,#78860,#78861,#78862,#78863,#78864,#78865,#78866,#78867,#78868,#78869,
#78870,#78871,#78872,#78873,#78874,#78875,#78876,#78877,#78878,#78879,#78880,
#78881,#78882,#78883,#78884,#78885,#78886,#78887,#78888,#78889,#78890,#78891,
#78892,#78893,#78894,#78895,#78896,#78897,#78898,#78899,#78900,#78901,#78902,
#78903,#78904,#78905,#78906,#78907,#78908,#78909,#78910,#78911,#78912,#78913,
#78914,#78915,#78916,#78917,#78918,#78919,#78920,#78921,#78922,#78923,#78924,
#78925,#78926,#78927,#78928,#78929,#78930,#78931,#78932,#78933,#78934,#78935,
#78936,#78937,#78938,#78939,#78940,#78941,#78942,#78943,#78944,#78945,#78946,
#78947,#78948,#78949,#78950,#78951,#78952,#78953,#78954,#78955,#78956,#78957,
#78958,#78959,#78960,#78961,#78962,#78963,#78964,#78965,#78966,#78967,#78968,
#78969,#78970,#78971,#78972,#78973,#78974,#78975,#78976,#78977,#78978,#78979,
#78980,#78981,#78982,#78983,#78984,#78985,#78986,#78987,#78988,#78989,#78990,
#78991,#78992,#78993,#78994,#78995,#78996,#78997,#78998,#78999,#79000,#79001,
#79002,#79003,#79004,#79005,#79006,#79007,#79008,#79009,#79010,#79011,#79012,
#79013,#79014,#79015,#79016,#79017,#79018,#79019,#79020,#79021,#79022,#79023,
#79024,#79025,#79026,#79027,#79028,#79029,#79030,#79031,#79032,#79033,#79034,
#79035,#79036,#79037,#79038,#79039,#79040,#79041,#79042,#79043,#79044,#79045,
#79046,#79047,#79048,#79049,#79050,#79051,#79052,#79053,#79054,#79055,#79056,
#79057,#79058,#79059,#79060,#79061,#79062,#79063,#79064,#79065,#79066,#79067,
#79068,#79069,#79070,#79071,#79072,#79073,#79074,#79075,#79076,#79077,#79078,
#79079,#79080,#79081,#79082,#79083,#79084,#79085,#79086,#79087,#79088,#79089,
#79090,#79091,#79092,#79093,#79094,#79095,#79096,#79097,#79098,#79099,#79100,
#79101,#79102,#79103,#79104,#79105,#79106,#79107,#79108,#79109,#79110,#79111,
#79112,#79113,#79114,#79115,#79116,#79117,#79118,#79119,#79120,#79121,#79122,
#79123,#79124,#79125,#79126,#79127,#79128,#79129,#79130,#79131,#79132,#79133,
#79134,#79135,#79136,#79137,#79138,#79139,#79140,#79141,#79142,#79143,#79144,
#79145,#79146,#79147,#79148,#79149,#79150,#79151,#79152,#79153,#79154,#79155,
#79156,#79157,#79158,#79159,#79160,#79161,#79162,#79163,#79164,#79165,#79166,
#79167,#79168,#79169,#79170,#79171,#79172,#79173,#79174,#79175,#79176,#79177,
#79178,#79179,#79180,#79181,#79182,#79183,#79184,#79185,#79186,#79187,#79188,
#79189,#79190,#79191,#79192,#79193,#79194,#79195,#79196,#79197,#79198,#79199,
#79200,#79201,#79202,#79203,#79204,#79205,#79206,#79207,#79208,#79209,#79210,
#79211,#79212,#79213,#79214,#79215,#79216,#79217,#79218,#79219,#79220,#79221,
#79222,#79223,#79224,#79225,#79226,#79227,#79228,#79229,#79230,#79231,#79232,
#79233,#79234,#79235,#79236,#79237,#79238,#79239,#79240,#79241,#79242,#79243,
#79244,#79245,#79246,#79247,#79248,#79249,#79250,#79251,#79252,#79253,#79254,
#79255,#79256,#79257,#79258,#79259,#79260,#79261,#79262,#79263,#79264,#79265,
#79266,#79267,#79268,#79269,#79270,#79271),(#79272,#79273,#79274,#79275,
#79276,#79277,#79278,#79279,#79280,#79281,#79282,#79283,#79284,#79285,#79286,
#79287,#79288,#79289,#79290,#79291,#79292,#79293,#79294,#79295,#79296,#79297,
#79298,#79299,#79300,#79301,#79302,#79303,#79304,#79305,#79306,#79307,#79308,
#79309,#79310,#79311,#79312,#79313,#79314,#79315,#79316,#79317,#79318,#79319,
#79320,#79321,#79322,#79323,#79324,#79325,#79326,#79327,#79328,#79329,#79330,
#79331,#79332,#79333,#79334,#79335,#79336,#79337,#79338,#79339,#79340,#79341,
#79342,#79343,#79344,#79345,#79346,#79347,#79348,#79349,#79350,#79351,#79352,
#79353,#79354,#79355,#79356,#79357,#79358,#79359,#79360,#79361,#79362,#79363,
#79364,#79365,#79366,#79367,#79368,#79369,#79370,#79371,#79372,#79373,#79374,
#79375,#79376,#79377,#79378,#79379,#79380,#79381,#79382,#79383,#79384,#79385,
#79386,#79387,#79388,#79389,#79390,#79391,#79392,#79393,#79394,#79395,#79396,
#79397,#79398,#79399,#79400,#79401,#79402,#79403,#79404,#79405,#79406,#79407,
#79408,#79409,#79410,#79411,#79412,#79413,#79414,#79415,#79416,#79417,#79418,
#79419,#79420,#79421,#79422,#79423,#79424,#79425,#79426,#79427,#79428,#79429,
#79430,#79431,#79432,#79433,#79434,#79435,#79436,#79437,#79438,#79439,#79440,
#79441,#79442,#79443,#79444,#79445,#79446,#79447,#79448,#79449,#79450,#79451,
#79452,#79453,#79454,#79455,#79456,#79457,#79458,#79459,#79460,#79461,#79462,
#79463,#79464,#79465,#79466,#79467,#79468,#79469,#79470,#79471,#79472,#79473,
#79474,#79475,#79476,#79477,#79478,#79479,#79480,#79481,#79482,#79483,#79484,
#79485,#79486,#79487,#79488,#79489,#79490,#79491,#79492,#79493,#79494,#79495,
#79496,#79497,#79498,#79499,#79500,#79501,#79502,#79503,#79504,#79505,#79506,
#79507,#79508,#79509,#79510,#79511,#79512,#79513,#79514,#79515,#79516,#79517,
#79518,#79519,#79520,#79521,#79522,#79523,#79524,#79525,#79526,#79527,#79528,
#79529,#79530,#79531,#79532,#79533,#79534,#79535,#79536,#79537,#79538,#79539,
#79540,#79541,#79542,#79543,#79544,#79545,#79546,#79547,#79548,#79549,#79550,
#79551,#79552,#79553,#79554,#79555,#79556,#79557,#79558,#79559,#79560,#79561,
#79562,#79563,#79564,#79565,#79566,#79567,#79568,#79569,#79570,#79571,#79572,
#79573,#79574,#79575,#79576,#79577,#79578,#79579,#79580,#79581,#79582,#79583,
#79584,#79585,#79586,#79587,#79588,#79589,#79590,#79591,#79592,#79593,#79594,
#79595,#79596,#79597,#79598,#79599,#79600,#79601,#79602,#79603,#79604,#79605,
#79606,#79607,#79608,#79609,#79610,#79611,#79612,#79613,#79614,#79615,#79616,
#79617,#79618,#79619,#79620,#79621,#79622,#79623,#79624,#79625,#79626,#79627,
#79628,#79629,#79630,#79631,#79632,#79633,#79634,#79635,#79636,#79637,#79638,
#79639,#79640,#79641,#79642,#79643,#79644,#79645,#79646,#79647,#79648,#79649,
#79650,#79651,#79652,#79653,#79654,#79655,#79656,#79657,#79658,#79659,#79660,
#79661,#79662,#79663,#79664,#79665,#79666,#79667,#79668,#79669,#79670,#79671,
#79672,#79673,#79674,#79675,#79676,#79677,#79678,#79679,#79680,#79681,#79682,
#79683,#79684,#79685,#79686,#79687,#79688,#79689,#79690,#79691,#79692,#79693,
#79694,#79695,#79696,#79697,#79698,#79699,#79700,#79701,#79702,#79703,#79704,
#79705,#79706,#79707,#79708,#79709,#79710,#79711,#79712,#79713,#79714,#79715,
#79716,#79717,#79718,#79719,#79720,#79721,#79722,#79723,#79724,#79725,#79726,
#79727,#79728,#79729,#79730,#79731,#79732,#79733,#79734,#79735,#79736,#79737,
#79738,#79739,#79740,#79741,#79742,#79743,#79744,#79745,#79746,#79747,#79748,
#79749),(#79750,#79751,#79752,#79753,#79754,#79755,#79756,#79757,#79758,
#79759,#79760,#79761,#79762,#79763,#79764,#79765,#79766,#79767,#79768,#79769,
#79770,#79771,#79772,#79773,#79774,#79775,#79776,#79777,#79778,#79779,#79780,
#79781,#79782,#79783,#79784,#79785,#79786,#79787,#79788,#79789,#79790,#79791,
#79792,#79793,#79794,#79795,#79796,#79797,#79798,#79799,#79800,#79801,#79802,
#79803,#79804,#79805,#79806,#79807,#79808,#79809,#79810,#79811,#79812,#79813,
#79814,#79815,#79816,#79817,#79818,#79819,#79820,#79821,#79822,#79823,#79824,
#79825,#79826,#79827,#79828,#79829,#79830,#79831,#79832,#79833,#79834,#79835,
#79836,#79837,#79838,#79839,#79840,#79841,#79842,#79843,#79844,#79845,#79846,
#79847,#79848,#79849,#79850,#79851,#79852,#79853,#79854,#79855,#79856,#79857,
#79858,#79859,#79860,#79861,#79862,#79863,#79864,#79865,#79866,#79867,#79868,
#79869,#79870,#79871,#79872,#79873,#79874,#79875,#79876,#79877,#79878,#79879,
#79880,#79881,#79882,#79883,#79884,#79885,#79886,#79887,#79888,#79889,#79890,
#79891,#79892,#79893,#79894,#79895,#79896,#79897,#79898,#79899,#79900,#79901,
#79902,#79903,#79904,#79905,#79906,#79907,#79908,#79909,#79910,#79911,#79912,
#79913,#79914,#79915,#79916,#79917,#79918,#79919,#79920,#79921,#79922,#79923,
#79924,#79925,#79926,#79927,#79928,#79929,#79930,#79931,#79932,#79933,#79934,
#79935,#79936,#79937,#79938,#79939,#79940,#79941,#79942,#79943,#79944,#79945,
#79946,#79947,#79948,#79949,#79950,#79951,#79952,#79953,#79954,#79955,#79956,
#79957,#79958,#79959,#79960,#79961,#79962,#79963,#79964,#79965,#79966,#79967,
#79968,#79969,#79970,#79971,#79972,#79973,#79974,#79975,#79976,#79977,#79978,
#79979,#79980,#79981,#79982,#79983,#79984,#79985,#79986,#79987,#79988,#79989,
#79990,#79991,#79992,#79993,#79994,#79995,#79996,#79997,#79998,#79999,#80000,
#80001,#80002,#80003,#80004,#80005,#80006,#80007,#80008,#80009,#80010,#80011,
#80012,#80013,#80014,#80015,#80016,#80017,#80018,#80019,#80020,#80021,#80022,
#80023,#80024,#80025,#80026,#80027,#80028,#80029,#80030,#80031,#80032,#80033,
#80034,#80035,#80036,#80037,#80038,#80039,#80040,#80041,#80042,#80043,#80044,
#80045,#80046,#80047,#80048,#80049,#80050,#80051,#80052,#80053,#80054,#80055,
#80056,#80057,#80058,#80059,#80060,#80061,#80062,#80063,#80064,#80065,#80066,
#80067,#80068,#80069,#80070,#80071,#80072,#80073,#80074,#80075,#80076,#80077,
#80078,#80079,#80080,#80081,#80082,#80083,#80084,#80085,#80086,#80087,#80088,
#80089,#80090,#80091,#80092,#80093,#80094,#80095,#80096,#80097,#80098,#80099,
#80100,#80101,#80102,#80103,#80104,#80105,#80106,#80107,#80108,#80109,#80110,
#80111,#80112,#80113,#80114,#80115,#80116,#80117,#80118,#80119,#80120,#80121,
#80122,#80123,#80124,#80125,#80126,#80127,#80128,#80129,#80130,#80131,#80132,
#80133,#80134,#80135,#80136,#80137,#80138,#80139,#80140,#80141,#80142,#80143,
#80144,#80145,#80146,#80147,#80148,#80149,#80150,#80151,#80152,#80153,#80154,
#80155,#80156,#80157,#80158,#80159,#80160,#80161,#80162,#80163,#80164,#80165,
#80166,#80167,#80168,#80169,#80170,#80171,#80172,#80173,#80174,#80175,#80176,
#80177,#80178,#80179,#80180,#80181,#80182,#80183,#80184,#80185,#80186,#80187,
#80188,#80189,#80190,#80191,#80192,#80193,#80194,#80195,#80196,#80197,#80198,
#80199,#80200,#80201,#80202,#80203,#80204,#80205,#80206,#80207,#80208,#80209,
#80210,#80211,#80212,#80213,#80214,#80215,#80216,#80217,#80218,#80219,#80220,
#80221,#80222,#80223,#80224,#80225,#80226,#80227)),.UNSPECIFIED.,.F.,.F.,
 .F.,(4,4),(4,1,1,1,1,1,1,1,1,1,1,1,1,1,1,1,1,1,1,1,1,1,1,1,1,1,1,1,1,1,
1,1,1,1,1,1,1,1,1,1,1,1,1,1,1,1,1,1,1,1,1,1,1,1,1,1,1,1,1,1,1,1,1,1,1,1,
1,1,1,1,1,1,1,1,1,1,1,1,1,1,1,1,1,1,1,1,1,1,1,1,1,1,1,1,1,1,1,1,1,1,1,1,
1,1,1,1,1,1,1,1,1,1,1,1,1,1,1,1,1,1,1,1,1,1,1,1,1,1,1,1,1,1,1,1,1,1,1,1,
1,1,1,1,1,1,1,1,1,1,1,1,1,1,1,1,1,1,1,1,1,1,1,1,1,1,1,1,1,1,1,1,1,1,1,1,
1,1,1,1,1,1,1,1,1,1,1,1,1,1,1,1,1,1,1,1,1,1,1,1,1,1,1,1,1,1,1,1,1,1,1,1,
1,1,1,1,1,1,1,1,1,1,1,1,1,1,1,1,1,1,1,1,1,1,1,1,1,1,1,1,1,1,1,1,1,1,1,1,
1,1,1,1,1,1,1,1,1,1,1,1,1,1,1,1,1,1,1,1,1,1,1,1,1,1,1,1,1,1,1,1,1,1,1,1,
1,1,1,1,1,1,1,1,1,1,1,1,1,1,1,1,1,1,1,1,1,1,1,1,1,1,1,1,1,1,1,1,1,1,1,1,
1,1,1,1,1,1,1,1,1,1,1,1,1,1,1,1,1,1,1,1,1,1,1,1,1,1,1,1,1,1,1,1,1,1,1,1,
1,1,1,1,1,1,1,1,1,1,1,1,1,1,1,1,1,1,1,1,1,1,1,1,1,1,1,1,1,1,1,1,1,1,1,1,
1,1,1,1,1,1,1,1,1,1,1,1,1,1,1,1,1,1,1,1,1,1,1,1,1,1,1,1,1,1,1,1,1,1,1,1,
1,1,1,1,1,1,1,1,1,1,1,1,1,1,1,1,1,1,1,1,1,1,1,1,1,1,1,1,1,1,1,1,1,1,1,1,
1,1,1,1,1,1,1,1,1,1,1,1,1,4),(0.,0.0496809906637672),(11.6147305479253,
12.1143106849507,12.613890821976,13.6130510960267,14.6122113700774,15.6113716441281,
16.6105319181787,17.6096921922294,18.6088524662801,19.6080127403308,20.6071730143815,
21.6063332884322,22.6054935624829,23.6046538365335,24.6038141105842,25.6029743846349,
26.6021346586856,27.6012949327363,28.600455206787,29.5996154808376,30.5987757548883,
31.597936028939,32.5970963029897,33.5962565770404,34.5954168510911,35.5945771251418,
36.5937373991924,37.5928976732431,38.5920579472938,39.5912182213445,40.5903784953952,
41.5895387694459,42.5886990434966,43.5878593175472,44.5870195915979,45.5861798656486,
46.5853401396993,47.58450041375,48.5836606878007,49.5828209618514,50.581981235902,
51.5811415099527,52.5803017840034,53.5794620580541,54.5786223321048,55.5777826061555,
56.5769428802061,57.5761031542568,58.5752634283075,59.5744237023582,60.5735839764089,
61.5727442504596,62.5719045245103,63.5710647985609,64.5702250726116,65.5693853466623,
66.568545620713,67.5677058947637,68.5668661688144,69.5660264428651,70.5651867169157,
71.5643469909664,72.5635072650171,73.5626675390678,74.5618278131185,75.5609880871692,
76.5601483612199,77.5593086352705,78.5584689093212,79.5576291833719,80.5567894574226,
81.5559497314733,82.555110005524,83.5542702795747,84.5534305536253,85.552590827676,
86.5517511017267,87.5509113757774,88.5500716498281,89.5492319238788,90.5483921979294,
91.5475524719801,92.5467127460308,93.5458730200815,94.5450332941322,95.5441935681829,
96.5433538422336,97.5425141162843,98.5416743903349,99.5408346643856,100.539994938436,
101.539155212487,102.538315486538,103.537475760588,104.536636034639,105.53579630869,
106.53495658274,107.534116856791,108.533277130842,109.532437404892,110.531597678943,
111.530757952994,112.529918227045,113.529078501095,114.528238775146,115.527399049197,
116.526559323247,117.525719597298,118.524879871349,119.524040145399,120.52320041945,
121.522360693501,122.521520967551,123.520681241602,124.519841515653,125.519001789703,
126.518162063754,127.517322337805,128.516482611855,129.515642885906,130.514803159957,
131.513963434008,132.513123708058,133.512283982109,134.51144425616,135.51060453021,
136.509764804261,137.508925078312,138.508085352362,139.507245626413,140.506405900464,
141.505566174514,142.504726448565,143.503886722616,144.503046996666,145.502207270717,
146.501367544768,147.500527818819,148.499688092869,149.49884836692,150.498008640971,
151.497168915021,152.496329189072,153.495489463123,154.494649737173,155.493810011224,
156.492970285275,157.492130559325,158.491290833376,159.490451107427,160.489611381477,
161.488771655528,162.487931929579,163.487092203629,164.48625247768,165.485412751731,
166.484573025782,167.483733299832,168.482893573883,169.482053847934,170.481214121984,
171.480374396035,172.479534670086,173.478694944136,174.477855218187,175.477015492238,
176.476175766288,177.475336040339,178.47449631439,179.47365658844,180.472816862491,
181.471977136542,182.471137410592,183.470297684643,184.469457958694,185.468618232745,
186.467778506795,187.466938780846,188.466099054897,189.465259328947,190.464419602998,
191.463579877049,192.462740151099,193.46190042515,194.461060699201,195.460220973251,
196.459381247302,197.458541521353,198.457701795403,199.456862069454,200.456022343505,
201.455182617555,202.454342891606,203.453503165657,204.452663439708,205.451823713758,
206.450983987809,207.45014426186,208.44930453591,209.448464809961,210.447625084012,
211.446785358062,212.445945632113,213.445105906164,214.444266180214,215.443426454265,
216.442586728316,217.441747002366,218.440907276417,219.440067550468,220.439227824519,
221.438388098569,222.43754837262,223.436708646671,224.435868920721,225.435029194772,
226.434189468823,227.433349742873,228.432510016924,229.431670290975,230.430830565025,
231.429990839076,232.429151113127,233.428311387177,234.427471661228,235.426631935279,
236.42579220933,237.42495248338,238.424112757431,239.423273031482,240.422433305532,
241.421593579583,242.420753853634,243.419914127684,244.419074401735,245.418234675786,
246.417394949836,247.416555223887,248.415715497938,249.414875771988,250.414036046039,
251.41319632009,252.41235659414,253.411516868191,254.410677142242,255.409837416293,
256.408997690343,257.408157964394,258.407318238445,259.406478512495,260.405638786546,
261.404799060597,262.403959334647,263.403119608698,264.402279882749,265.401440156799,
266.40060043085,267.399760704901,268.398920978951,269.398081253002,270.397241527053,
271.396401801103,272.395562075154,273.394722349205,274.393882623256,275.393042897306,
276.392203171357,277.391363445408,278.390523719458,279.389683993509,280.38884426756,
281.38800454161,282.387164815661,283.386325089712,284.385485363762,285.384645637813,
286.383805911864,287.382966185914,288.382126459965,289.381286734016,290.380447008066,
291.379607282117,292.378767556168,293.377927830219,294.377088104269,295.37624837832,
296.375408652371,297.374568926421,298.373729200472,299.372889474523,300.372049748573,
301.371210022624,302.370370296675,303.369530570725,304.368690844776,305.367851118827,
306.367011392877,307.366171666928,308.365331940979,309.364492215029,310.36365248908,
311.362812763131,312.361973037182,313.361133311232,314.360293585283,315.359453859334,
316.358614133384,317.357774407435,318.356934681486,319.356094955536,320.355255229587,
321.354415503638,322.353575777688,323.352736051739,324.35189632579,325.35105659984,
326.350216873891,327.349377147942,328.348537421993,329.347697696043,330.346857970094,
331.346018244145,332.345178518195,333.344338792246,334.343499066297,335.342659340347,
336.341819614398,337.340979888449,338.340140162499,339.33930043655,340.338460710601,
341.337620984651,342.336781258702,343.335941532753,344.335101806803,345.334262080854,
346.333422354905,347.332582628956,348.331742903006,349.330903177057,350.330063451108,
351.329223725158,352.328383999209,353.32754427326,354.32670454731,355.325864821361,
356.325025095412,357.324185369462,358.323345643513,359.322505917564,360.321666191614,
361.320826465665,362.319986739716,363.319147013766,364.318307287817,365.317467561868,
366.316627835919,367.315788109969,368.31494838402,369.314108658071,370.313268932121,
371.312429206172,372.311589480223,373.310749754273,374.309910028324,375.309070302375,
376.308230576425,377.307390850476,378.306551124527,379.305711398577,380.304871672628,
381.304031946679,382.303192220729,383.30235249478,384.301512768831,385.300673042882,
386.299833316932,387.298993590983,388.298153865034,389.297314139084,390.296474413135,
391.295634687186,392.294794961236,393.293955235287,394.293115509338,395.292275783388,
396.291436057439,397.29059633149,398.289756605541,399.288916879591,400.288077153642,
401.287237427693,402.286397701743,403.285557975794,404.284718249845,405.283878523895,
406.283038797946,407.282199071997,408.281359346047,409.280519620098,410.279679894149,
411.278840168199,412.27800044225,413.277160716301,414.276320990351,415.275481264402,
416.274641538453,417.273801812504,418.272962086554,419.272122360605,420.271282634656,
421.270442908706,422.269603182757,423.268763456808,424.267923730858,425.267084004909,
426.26624427896,427.26540455301,428.264564827061,429.263725101112,430.262885375162,
431.262045649213,432.261205923264,433.260366197314,434.259526471365,435.258686745416,
436.257847019467,437.257007293517,438.256167567568,439.255327841619,440.254488115669,
441.25364838972,442.252808663771,443.251968937821,444.251129211872,445.250289485923,
446.249449759973,447.248610034024,448.247770308075,449.246930582125,450.246090856176,
451.245251130227,452.244411404278,453.243571678328,454.242731952379,455.24189222643,
456.24105250048,457.240212774531,458.239373048582,459.238533322632,460.237693596683,
461.236853870734,462.236014144784,463.235174418835,464.234334692886,465.233494966936,
466.232655240987,467.231815515038,468.230975789088,469.230136063139,470.22929633719,
471.228456611241,472.227616885291,473.226777159342,474.225937433393,475.225097707443,
476.224257981494,477.223418255545,478.222578529595,479.221738803646,480.220899077697,
481.220059351747,482.219219625798,483.218379899849,483.717960036874,484.217540173899),
 .UNSPECIFIED.);
#850=CYLINDRICAL_SURFACE('',#32983,4.954);
#851=CYLINDRICAL_SURFACE('',#32985,4.954);
#852=CYLINDRICAL_SURFACE('',#32986,4.954);
#853=CYLINDRICAL_SURFACE('',#32987,4.954);
#854=CYLINDRICAL_SURFACE('',#32988,4.954);
#855=CYLINDRICAL_SURFACE('',#32989,4.954);
#856=CYLINDRICAL_SURFACE('',#32990,4.954);
#857=CYLINDRICAL_SURFACE('',#32991,4.954);
#858=CYLINDRICAL_SURFACE('',#32992,4.954);
#859=CYLINDRICAL_SURFACE('',#32993,4.954);
#860=CYLINDRICAL_SURFACE('',#32994,4.954);
#861=CYLINDRICAL_SURFACE('',#32995,4.954);
#862=CYLINDRICAL_SURFACE('',#32996,4.954);
#863=CYLINDRICAL_SURFACE('',#32997,4.954);
#864=CYLINDRICAL_SURFACE('',#32998,4.954);
#865=CYLINDRICAL_SURFACE('',#32999,4.954);
#866=CYLINDRICAL_SURFACE('',#33000,4.954);
#867=CYLINDRICAL_SURFACE('',#33001,4.954);
#868=CYLINDRICAL_SURFACE('',#33002,4.954);
#869=CYLINDRICAL_SURFACE('',#33003,4.954);
#870=CYLINDRICAL_SURFACE('',#33004,4.954);
#871=CYLINDRICAL_SURFACE('',#33005,4.954);
#872=CYLINDRICAL_SURFACE('',#33006,4.954);
#873=CYLINDRICAL_SURFACE('',#33007,4.954);
#874=CYLINDRICAL_SURFACE('',#33008,4.954);
#875=CYLINDRICAL_SURFACE('',#33009,4.954);
#876=CYLINDRICAL_SURFACE('',#33010,4.954);
#877=CYLINDRICAL_SURFACE('',#33011,4.954);
#878=CYLINDRICAL_SURFACE('',#33012,4.954);
#879=CYLINDRICAL_SURFACE('',#33013,4.954);
#880=CYLINDRICAL_SURFACE('',#33014,4.954);
#881=CYLINDRICAL_SURFACE('',#33015,4.954);
#882=CYLINDRICAL_SURFACE('',#33016,4.954);
#883=CYLINDRICAL_SURFACE('',#33017,4.954);
#884=CYLINDRICAL_SURFACE('',#33018,4.954);
#885=CYLINDRICAL_SURFACE('',#33019,4.954);
#886=CYLINDRICAL_SURFACE('',#33020,4.954);
#887=CYLINDRICAL_SURFACE('',#33021,4.954);
#888=CYLINDRICAL_SURFACE('',#33022,4.954);
#889=CYLINDRICAL_SURFACE('',#33023,4.954);
#890=CYLINDRICAL_SURFACE('',#33024,4.954);
#891=CYLINDRICAL_SURFACE('',#33025,4.954);
#892=CYLINDRICAL_SURFACE('',#33026,4.954);
#893=CYLINDRICAL_SURFACE('',#33027,4.954);
#894=CYLINDRICAL_SURFACE('',#33028,4.954);
#895=CYLINDRICAL_SURFACE('',#33029,4.954);
#896=CYLINDRICAL_SURFACE('',#33030,4.954);
#897=CYLINDRICAL_SURFACE('',#33031,4.954);
#898=CYLINDRICAL_SURFACE('',#33032,4.954);
#899=CYLINDRICAL_SURFACE('',#33033,4.954);
#900=CYLINDRICAL_SURFACE('',#33034,4.954);
#901=CYLINDRICAL_SURFACE('',#33035,4.954);
#902=CYLINDRICAL_SURFACE('',#33036,4.954);
#903=CYLINDRICAL_SURFACE('',#33037,4.954);
#904=CYLINDRICAL_SURFACE('',#33038,4.954);
#905=CYLINDRICAL_SURFACE('',#33039,4.954);
#906=CYLINDRICAL_SURFACE('',#33040,4.954);
#907=CYLINDRICAL_SURFACE('',#33041,4.954);
#908=CYLINDRICAL_SURFACE('',#33042,4.954);
#909=CYLINDRICAL_SURFACE('',#33043,4.954);
#910=CYLINDRICAL_SURFACE('',#33044,4.954);
#911=CYLINDRICAL_SURFACE('',#33045,4.954);
#912=CYLINDRICAL_SURFACE('',#33046,4.954);
#913=CYLINDRICAL_SURFACE('',#33047,4.954);
#914=CYLINDRICAL_SURFACE('',#33048,4.954);
#915=CYLINDRICAL_SURFACE('',#33049,4.954);
#916=CYLINDRICAL_SURFACE('',#33050,4.954);
#917=CYLINDRICAL_SURFACE('',#33051,4.954);
#918=CYLINDRICAL_SURFACE('',#33052,4.954);
#919=CYLINDRICAL_SURFACE('',#33053,4.954);
#920=CYLINDRICAL_SURFACE('',#33054,4.954);
#921=CYLINDRICAL_SURFACE('',#33055,4.954);
#922=CYLINDRICAL_SURFACE('',#33056,4.954);
#923=CYLINDRICAL_SURFACE('',#33057,4.954);
#924=CYLINDRICAL_SURFACE('',#33058,4.954);
#925=CYLINDRICAL_SURFACE('',#33059,4.52375);
#926=CYLINDRICAL_SURFACE('',#33061,4.52375);
#927=CYLINDRICAL_SURFACE('',#33062,4.52375);
#928=CYLINDRICAL_SURFACE('',#33063,4.52375);
#929=CYLINDRICAL_SURFACE('',#33064,4.52375);
#930=CYLINDRICAL_SURFACE('',#33065,4.52375);
#931=CYLINDRICAL_SURFACE('',#33066,4.52375);
#932=CYLINDRICAL_SURFACE('',#33067,4.52375);
#933=CYLINDRICAL_SURFACE('',#33068,4.52375);
#934=CYLINDRICAL_SURFACE('',#33069,4.52375);
#935=CYLINDRICAL_SURFACE('',#33070,4.52375);
#936=CYLINDRICAL_SURFACE('',#33071,4.52375);
#937=CYLINDRICAL_SURFACE('',#33072,4.52375);
#938=CYLINDRICAL_SURFACE('',#33073,4.52375);
#939=CYLINDRICAL_SURFACE('',#33074,4.52375);
#940=CYLINDRICAL_SURFACE('',#33075,4.52375);
#941=CYLINDRICAL_SURFACE('',#33076,4.52375);
#942=CYLINDRICAL_SURFACE('',#33077,4.52375);
#943=CYLINDRICAL_SURFACE('',#33078,4.52375);
#944=CYLINDRICAL_SURFACE('',#33079,4.52375);
#945=CYLINDRICAL_SURFACE('',#33080,4.52375);
#946=CYLINDRICAL_SURFACE('',#33081,4.52375);
#947=CYLINDRICAL_SURFACE('',#33082,4.52375);
#948=CYLINDRICAL_SURFACE('',#33083,4.52375);
#949=CYLINDRICAL_SURFACE('',#33084,4.52375);
#950=CYLINDRICAL_SURFACE('',#33085,4.52375);
#951=CYLINDRICAL_SURFACE('',#33086,4.52375);
#952=CYLINDRICAL_SURFACE('',#33087,4.52375);
#953=CYLINDRICAL_SURFACE('',#33088,4.52375);
#954=CYLINDRICAL_SURFACE('',#33089,4.52375);
#955=CYLINDRICAL_SURFACE('',#33090,4.52375);
#956=CYLINDRICAL_SURFACE('',#33091,4.52375);
#957=CYLINDRICAL_SURFACE('',#33092,4.52375);
#958=CYLINDRICAL_SURFACE('',#33093,4.52375);
#959=CYLINDRICAL_SURFACE('',#33094,4.52375);
#960=CYLINDRICAL_SURFACE('',#33095,4.52375);
#961=CYLINDRICAL_SURFACE('',#33096,4.52375);
#962=CYLINDRICAL_SURFACE('',#33097,4.52375);
#963=CYLINDRICAL_SURFACE('',#33098,4.52375);
#964=CYLINDRICAL_SURFACE('',#33099,4.52375);
#965=CYLINDRICAL_SURFACE('',#33100,4.52375);
#966=CYLINDRICAL_SURFACE('',#33101,4.52375);
#967=CYLINDRICAL_SURFACE('',#33102,4.52375);
#968=CYLINDRICAL_SURFACE('',#33103,4.52375);
#969=CYLINDRICAL_SURFACE('',#33104,4.52375);
#970=CYLINDRICAL_SURFACE('',#33105,4.52375);
#971=CYLINDRICAL_SURFACE('',#33106,4.52375);
#972=CYLINDRICAL_SURFACE('',#33107,4.52375);
#973=CYLINDRICAL_SURFACE('',#33108,4.52375);
#974=CYLINDRICAL_SURFACE('',#33109,4.52375);
#975=CYLINDRICAL_SURFACE('',#33110,4.52375);
#976=CYLINDRICAL_SURFACE('',#33111,4.52375);
#977=CYLINDRICAL_SURFACE('',#33112,4.52375);
#978=CYLINDRICAL_SURFACE('',#33113,4.52375);
#979=CYLINDRICAL_SURFACE('',#33114,4.52375);
#980=CYLINDRICAL_SURFACE('',#33115,4.52375);
#981=CYLINDRICAL_SURFACE('',#33116,4.52375);
#982=CYLINDRICAL_SURFACE('',#33117,4.52375);
#983=CYLINDRICAL_SURFACE('',#33118,4.52375);
#984=CYLINDRICAL_SURFACE('',#33119,4.52375);
#985=CYLINDRICAL_SURFACE('',#33120,4.52375);
#986=CYLINDRICAL_SURFACE('',#33121,4.52375);
#987=CYLINDRICAL_SURFACE('',#33122,4.52375);
#988=CYLINDRICAL_SURFACE('',#33123,4.52375);
#989=CYLINDRICAL_SURFACE('',#33124,4.52375);
#990=CYLINDRICAL_SURFACE('',#33125,4.52375);
#991=CYLINDRICAL_SURFACE('',#33126,4.52375);
#992=CYLINDRICAL_SURFACE('',#33127,4.52375);
#993=CYLINDRICAL_SURFACE('',#33128,4.52375);
#994=CYLINDRICAL_SURFACE('',#33129,4.52375);
#995=CYLINDRICAL_SURFACE('',#33130,4.52375);
#996=CYLINDRICAL_SURFACE('',#33131,4.52375);
#997=CYLINDRICAL_SURFACE('',#33132,4.52375);
#998=CYLINDRICAL_SURFACE('',#33133,4.52375);
#999=CYLINDRICAL_SURFACE('',#33134,4.52375);
#1000=CYLINDRICAL_SURFACE('',#33142,4.52375);
#1001=CYLINDRICAL_SURFACE('',#33143,2.5);
#1002=CYLINDRICAL_SURFACE('',#33147,4.954);
#1765=CIRCLE('',#32984,4.954);
#1766=CIRCLE('',#33060,4.52375);
#1767=CIRCLE('',#33136,4.954);
#1768=CIRCLE('',#33137,4.954);
#1769=CIRCLE('',#33139,4.954);
#1770=CIRCLE('',#33140,4.954);
#1771=CIRCLE('',#33141,4.52375);
#1772=CIRCLE('',#33144,2.5);
#1773=CIRCLE('',#33145,2.5);
#1774=CIRCLE('',#33148,4.954);
#1775=CIRCLE('',#33150,4.5);
#1776=CIRCLE('',#33153,3.00000000000001);
#2061=CONICAL_SURFACE('',#33146,3.75,1.19028994968253);
#2062=CONICAL_SURFACE('',#33149,4.75,0.78539816339745);
#2912=B_SPLINE_CURVE_WITH_KNOTS('',3,(#70397,#70398,#70399,#70400,#70401,
#70402,#70403,#70404,#70405,#70406),.UNSPECIFIED.,.F.,.F.,(4,3,3,4),(-4.09323272002468,
-3.99664109620274,-2.99748082215206,-2.08103247056466),.UNSPECIFIED.);
#2913=B_SPLINE_CURVE_WITH_KNOTS('',3,(#70409,#70410,#70411,#70412,#70413,
#70414,#70415,#70416,#70417,#70418),.UNSPECIFIED.,.F.,.F.,(4,3,3,4),(0.,
0.499580137025342,0.999160274050685,1.12939240413109),.UNSPECIFIED.);
#2914=B_SPLINE_CURVE_WITH_KNOTS('',3,(#70423,#70424,#70425,#70426,#70427,
#70428,#70429,#70430,#70431,#70432,#70433,#70434,#70435,#70436,#70437,#70438,
#70439,#70440,#70441,#70442,#70443,#70444),.UNSPECIFIED.,.F.,.F.,(4,3,3,
3,3,3,3,4),(-10.3764180272043,-9.99160274050685,-8.99244246645616,-7.99328219240548,
-6.9941219183548,-5.99496164430411,-4.99580137025343,-4.09323272002468),
 .UNSPECIFIED.);
#2915=B_SPLINE_CURVE_WITH_KNOTS('',3,(#70445,#70446,#70447,#70448,#70449,
#70450,#70451,#70452,#70453,#70454,#70455,#70456,#70457,#70458,#70459,#70460,
#70461,#70462,#70463,#70464,#70465,#70466),.UNSPECIFIED.,.F.,.F.,(4,3,3,
3,3,3,3,4),(1.12939240413109,1.99832054810137,2.99748082215204,3.99664109620273,
4.9958013702534,5.99496164430408,6.99412191835476,7.41257771131067),
 .UNSPECIFIED.);
#2916=B_SPLINE_CURVE_WITH_KNOTS('',3,(#70471,#70472,#70473,#70474,#70475,
#70476,#70477,#70478,#70479,#70480,#70481,#70482,#70483,#70484,#70485,#70486,
#70487,#70488,#70489,#70490,#70491,#70492),.UNSPECIFIED.,.F.,.F.,(4,3,3,
3,3,3,3,4),(-16.6596033343839,-15.986564384811,-14.9874041107603,-13.9882438367096,
-12.9890835626589,-11.9899232886082,-10.9907630145575,-10.3764180272043),
 .UNSPECIFIED.);
#2917=B_SPLINE_CURVE_WITH_KNOTS('',3,(#70493,#70494,#70495,#70496,#70497,
#70498,#70499,#70500,#70501,#70502,#70503,#70504,#70505,#70506,#70507,#70508,
#70509,#70510,#70511,#70512,#70513,#70514),.UNSPECIFIED.,.F.,.F.,(4,3,3,
3,3,3,3,4),(7.41257771131067,7.99328219240545,8.99244246645615,9.99160274050685,
10.9907630145575,11.9899232886082,12.9890835626589,13.6957630184903),
 .UNSPECIFIED.);
#2918=B_SPLINE_CURVE_WITH_KNOTS('',3,(#70519,#70520,#70521,#70522,#70523,
#70524,#70525,#70526,#70527,#70528,#70529,#70530,#70531,#70532,#70533,#70534,
#70535,#70536,#70537,#70538,#70539,#70540),.UNSPECIFIED.,.F.,.F.,(4,3,3,
3,3,3,3,4),(-22.9427886415634,-21.9815260291151,-20.9823657550644,-19.9832054810137,
-18.984045206963,-17.9848849329123,-16.9857246588616,-16.6596033343839),
 .UNSPECIFIED.);
#2919=B_SPLINE_CURVE_WITH_KNOTS('',3,(#70541,#70542,#70543,#70544,#70545,
#70546,#70547,#70548,#70549,#70550,#70551,#70552,#70553,#70554,#70555,#70556,
#70557,#70558,#70559,#70560,#70561,#70562),.UNSPECIFIED.,.F.,.F.,(4,3,3,
3,3,3,3,4),(13.6957630184903,13.9882438367096,14.9874041107603,15.986564384811,
16.9857246588617,17.9848849329123,18.984045206963,19.9789483256699),
 .UNSPECIFIED.);
#2920=B_SPLINE_CURVE_WITH_KNOTS('',3,(#70567,#70568,#70569,#70570,#70571,
#70572,#70573,#70574,#70575,#70576,#70577,#70578,#70579,#70580,#70581,#70582,
#70583,#70584,#70585,#70586,#70587,#70588,#70589,#70590,#70591),
 .UNSPECIFIED.,.F.,.F.,(4,3,3,3,3,3,3,3,4),(-29.225973948743,-28.9756479474699,
-27.9764876734192,-26.9773273993685,-25.9781671253178,-24.9790068512671,
-23.9798465772164,-22.9806863031658,-22.9427886415634),.UNSPECIFIED.);
#2921=B_SPLINE_CURVE_WITH_KNOTS('',3,(#70592,#70593,#70594,#70595,#70596,
#70597,#70598,#70599,#70600,#70601,#70602,#70603,#70604,#70605,#70606,#70607,
#70608,#70609,#70610,#70611,#70612,#70613,#70614,#70615,#70616),
 .UNSPECIFIED.,.F.,.F.,(4,3,3,3,3,3,3,3,4),(19.9789483256699,19.9832054810137,
20.9823657550644,21.9815260291151,22.9806863031658,23.9798465772165,24.9790068512671,
25.9781671253178,26.2621336328494),.UNSPECIFIED.);
#2922=B_SPLINE_CURVE_WITH_KNOTS('',3,(#70621,#70622,#70623,#70624,#70625,
#70626,#70627,#70628,#70629,#70630,#70631,#70632,#70633,#70634,#70635,#70636,
#70637,#70638,#70639,#70640,#70641,#70642),.UNSPECIFIED.,.F.,.F.,(4,3,3,
3,3,3,3,4),(-35.5091592559226,-34.970609591774,-33.9714493177233,-32.9722890436726,
-31.9731287696219,-30.9739684955712,-29.9748082215206,-29.225973948743),
 .UNSPECIFIED.);
#2923=B_SPLINE_CURVE_WITH_KNOTS('',3,(#70643,#70644,#70645,#70646,#70647,
#70648,#70649,#70650,#70651,#70652,#70653,#70654,#70655,#70656,#70657,#70658,
#70659,#70660,#70661,#70662,#70663,#70664),.UNSPECIFIED.,.F.,.F.,(4,3,3,
3,3,3,3,4),(26.2621336328494,26.9773273993685,27.9764876734192,28.9756479474699,
29.9748082215206,30.9739684955713,31.9731287696219,32.545318940029),
 .UNSPECIFIED.);
#2924=B_SPLINE_CURVE_WITH_KNOTS('',3,(#70669,#70670,#70671,#70672,#70673,
#70674,#70675,#70676,#70677,#70678,#70679,#70680,#70681,#70682,#70683,#70684,
#70685,#70686,#70687,#70688,#70689,#70690),.UNSPECIFIED.,.F.,.F.,(4,3,3,
3,3,3,3,4),(-41.7923445631022,-40.9655712360781,-39.9664109620274,-38.9672506879767,
-37.968090413926,-36.9689301398754,-35.9697698658247,-35.5091592559226),
 .UNSPECIFIED.);
#2925=B_SPLINE_CURVE_WITH_KNOTS('',3,(#70691,#70692,#70693,#70694,#70695,
#70696,#70697,#70698,#70699,#70700,#70701,#70702,#70703,#70704,#70705,#70706,
#70707,#70708,#70709,#70710,#70711,#70712),.UNSPECIFIED.,.F.,.F.,(4,3,3,
3,3,3,3,4),(32.545318940029,32.9722890436726,33.9714493177233,34.970609591774,
35.9697698658247,36.9689301398753,37.968090413926,38.8285042472086),
 .UNSPECIFIED.);
#2926=B_SPLINE_CURVE_WITH_KNOTS('',3,(#70717,#70718,#70719,#70720,#70721,
#70722,#70723,#70724,#70725,#70726,#70727,#70728,#70729,#70730,#70731,#70732,
#70733,#70734,#70735,#70736,#70737,#70738,#70739,#70740,#70741),
 .UNSPECIFIED.,.F.,.F.,(4,3,3,3,3,3,3,3,4),(-48.0755298702818,-47.9596931544329,
-46.9605328803822,-45.9613726063315,-44.9622123322808,-43.9630520582302,
-42.9638917841795,-41.9647315101288,-41.7923445631022),.UNSPECIFIED.);
#2927=B_SPLINE_CURVE_WITH_KNOTS('',3,(#70742,#70743,#70744,#70745,#70746,
#70747,#70748,#70749,#70750,#70751,#70752,#70753,#70754,#70755,#70756,#70757,
#70758,#70759,#70760,#70761,#70762,#70763,#70764,#70765,#70766),
 .UNSPECIFIED.,.F.,.F.,(4,3,3,3,3,3,3,3,4),(38.8285042472086,38.9672506879767,
39.9664109620274,40.9655712360781,41.9647315101288,42.9638917841795,43.9630520582302,
44.9622123322809,45.1116895543882),.UNSPECIFIED.);
#2928=B_SPLINE_CURVE_WITH_KNOTS('',3,(#70771,#70772,#70773,#70774,#70775,
#70776,#70777,#70778,#70779,#70780,#70781,#70782,#70783,#70784,#70785,#70786,
#70787,#70788,#70789,#70790,#70791,#70792),.UNSPECIFIED.,.F.,.F.,(4,3,3,
3,3,3,3,4),(-54.3587151774614,-53.954654798737,-52.9554945246863,-51.9563342506356,
-50.9571739765849,-49.9580137025343,-48.9588534284836,-48.0755298702818),
 .UNSPECIFIED.);
#2929=B_SPLINE_CURVE_WITH_KNOTS('',3,(#70793,#70794,#70795,#70796,#70797,
#70798,#70799,#70800,#70801,#70802,#70803,#70804,#70805,#70806,#70807,#70808,
#70809,#70810,#70811,#70812,#70813,#70814),.UNSPECIFIED.,.F.,.F.,(4,3,3,
3,3,3,3,4),(45.1116895543882,45.9613726063316,46.9605328803822,47.9596931544329,
48.9588534284836,49.9580137025343,50.9571739765849,51.3948748615678),
 .UNSPECIFIED.);
#2930=B_SPLINE_CURVE_WITH_KNOTS('',3,(#70819,#70820,#70821,#70822,#70823,
#70824,#70825,#70826,#70827,#70828,#70829,#70830,#70831,#70832,#70833,#70834,
#70835,#70836,#70837,#70838,#70839,#70840),.UNSPECIFIED.,.F.,.F.,(4,3,3,
3,3,3,3,4),(-60.641900484641,-59.9496164430411,-58.9504561689904,-57.9512958949397,
-56.9521356208891,-55.9529753468384,-54.9538150727877,-54.3587151774614),
 .UNSPECIFIED.);
#2931=B_SPLINE_CURVE_WITH_KNOTS('',3,(#70841,#70842,#70843,#70844,#70845,
#70846,#70847,#70848,#70849,#70850,#70851,#70852,#70853,#70854,#70855,#70856,
#70857,#70858,#70859,#70860,#70861,#70862),.UNSPECIFIED.,.F.,.F.,(4,3,3,
3,3,3,3,4),(51.3948748615678,51.9563342506356,52.9554945246863,53.954654798737,
54.9538150727877,55.9529753468384,56.9521356208891,57.6780601687474),
 .UNSPECIFIED.);
#2932=B_SPLINE_CURVE_WITH_KNOTS('',3,(#70867,#70868,#70869,#70870,#70871,
#70872,#70873,#70874,#70875,#70876,#70877,#70878,#70879,#70880,#70881,#70882,
#70883,#70884,#70885,#70886,#70887,#70888),.UNSPECIFIED.,.F.,.F.,(4,3,3,
3,3,3,3,4),(-66.9250857918206,-65.9445780873452,-64.9454178132945,-63.9462575392438,
-62.9470972651932,-61.9479369911425,-60.9487767170918,-60.641900484641),
 .UNSPECIFIED.);
#2933=B_SPLINE_CURVE_WITH_KNOTS('',3,(#70889,#70890,#70891,#70892,#70893,
#70894,#70895,#70896,#70897,#70898,#70899,#70900,#70901,#70902,#70903,#70904,
#70905,#70906,#70907,#70908,#70909,#70910,#70911,#70912,#70913),
 .UNSPECIFIED.,.F.,.F.,(4,3,3,3,3,3,3,3,4),(57.6780601687474,57.9512958949398,
58.9504561689905,59.9496164430411,60.9487767170918,61.9479369911425,62.9470972651932,
63.9462575392438,63.961245475927),.UNSPECIFIED.);
#2934=B_SPLINE_CURVE_WITH_KNOTS('',3,(#70918,#70919,#70920,#70921,#70922,
#70923,#70924,#70925,#70926,#70927,#70928,#70929,#70930,#70931,#70932,#70933,
#70934,#70935,#70936,#70937,#70938,#70939,#70940,#70941,#70942),
 .UNSPECIFIED.,.F.,.F.,(4,3,3,3,3,3,3,3,4),(-73.2082710990002,-72.9387000057,
-71.9395397316493,-70.9403794575987,-69.941219183548,-68.9420589094973,
-67.9428986354466,-66.9437383613959,-66.9250857918206),.UNSPECIFIED.);
#2935=B_SPLINE_CURVE_WITH_KNOTS('',3,(#70943,#70944,#70945,#70946,#70947,
#70948,#70949,#70950,#70951,#70952,#70953,#70954,#70955,#70956,#70957,#70958,
#70959,#70960,#70961,#70962,#70963,#70964),.UNSPECIFIED.,.F.,.F.,(4,3,3,
3,3,3,3,4),(63.961245475927,64.9454178132945,65.9445780873452,66.9437383613959,
67.9428986354466,68.9420589094973,69.941219183548,70.2444307831066),
 .UNSPECIFIED.);
#2936=B_SPLINE_CURVE_WITH_KNOTS('',3,(#70969,#70970,#70971,#70972,#70973,
#70974,#70975,#70976,#70977,#70978,#70979,#70980,#70981,#70982,#70983,#70984,
#70985,#70986,#70987,#70988,#70989,#70990),.UNSPECIFIED.,.F.,.F.,(4,3,3,
3,3,3,3,4),(-79.4914564061798,-78.9336616500041,-77.9345013759535,-76.9353411019028,
-75.9361808278521,-74.9370205538014,-73.9378602797507,-73.2082710990002),
 .UNSPECIFIED.);
#2937=B_SPLINE_CURVE_WITH_KNOTS('',3,(#70991,#70992,#70993,#70994,#70995,
#70996,#70997,#70998,#70999,#71000,#71001,#71002,#71003,#71004,#71005,#71006,
#71007,#71008,#71009,#71010,#71011,#71012),.UNSPECIFIED.,.F.,.F.,(4,3,3,
3,3,3,3,4),(70.2444307831066,70.9403794575987,71.9395397316494,72.9387000057001,
73.9378602797507,74.9370205538014,75.9361808278521,76.5276160902862),
 .UNSPECIFIED.);
#2938=B_SPLINE_CURVE_WITH_KNOTS('',3,(#71017,#71018,#71019,#71020,#71021,
#71022,#71023,#71024,#71025,#71026,#71027,#71028,#71029,#71030,#71031,#71032,
#71033,#71034,#71035,#71036,#71037,#71038),.UNSPECIFIED.,.F.,.F.,(4,3,3,
3,3,3,3,4),(-85.7746417133594,-84.9286232943083,-83.9294630202576,-82.9303027462069,
-81.9311424721562,-80.9319821981055,-79.9328219240548,-79.4914564061798),
 .UNSPECIFIED.);
#2939=B_SPLINE_CURVE_WITH_KNOTS('',3,(#71039,#71040,#71041,#71042,#71043,
#71044,#71045,#71046,#71047,#71048,#71049,#71050,#71051,#71052,#71053,#71054,
#71055,#71056,#71057,#71058,#71059,#71060),.UNSPECIFIED.,.F.,.F.,(4,3,3,
3,3,3,3,4),(76.5276160902862,76.9353411019028,77.9345013759535,78.9336616500042,
79.9328219240548,80.9319821981055,81.9311424721562,82.8108013974658),
 .UNSPECIFIED.);
#2940=B_SPLINE_CURVE_WITH_KNOTS('',3,(#71065,#71066,#71067,#71068,#71069,
#71070,#71071,#71072,#71073,#71074,#71075,#71076,#71077,#71078,#71079,#71080,
#71081,#71082,#71083,#71084,#71085,#71086,#71087,#71088,#71089),
 .UNSPECIFIED.,.F.,.F.,(4,3,3,3,3,3,3,3,4),(-92.057827020539,-91.922745212663,
-90.9235849386124,-89.9244246645617,-88.925264390511,-87.9261041164603,
-86.9269438424096,-85.9277835683589,-85.7746417133594),.UNSPECIFIED.);
#2941=B_SPLINE_CURVE_WITH_KNOTS('',3,(#71090,#71091,#71092,#71093,#71094,
#71095,#71096,#71097,#71098,#71099,#71100,#71101,#71102,#71103,#71104,#71105,
#71106,#71107,#71108,#71109,#71110,#71111,#71112,#71113,#71114),
 .UNSPECIFIED.,.F.,.F.,(4,3,3,3,3,3,3,3,4),(82.8108013974658,82.9303027462069,
83.9294630202576,84.9286232943083,85.9277835683589,86.9269438424096,87.9261041164603,
88.925264390511,89.0939867046454),.UNSPECIFIED.);
#2942=B_SPLINE_CURVE_WITH_KNOTS('',3,(#71119,#71120,#71121,#71122,#71123,
#71124,#71125,#71126,#71127,#71128,#71129,#71130,#71131,#71132,#71133,#71134,
#71135,#71136,#71137,#71138,#71139,#71140),.UNSPECIFIED.,.F.,.F.,(4,3,3,
3,3,3,3,4),(-98.3410123277185,-97.9177068569672,-96.9185465829165,-95.9193863088658,
-94.9202260348151,-93.9210657607644,-92.9219054867137,-92.057827020539),
 .UNSPECIFIED.);
#2943=B_SPLINE_CURVE_WITH_KNOTS('',3,(#71141,#71142,#71143,#71144,#71145,
#71146,#71147,#71148,#71149,#71150,#71151,#71152,#71153,#71154,#71155,#71156,
#71157,#71158,#71159,#71160,#71161,#71162),.UNSPECIFIED.,.F.,.F.,(4,3,3,
3,3,3,3,4),(89.0939867046454,89.9244246645617,90.9235849386124,91.922745212663,
92.9219054867137,93.9210657607644,94.9202260348151,95.377172011825),
 .UNSPECIFIED.);
#2944=B_SPLINE_CURVE_WITH_KNOTS('',3,(#71167,#71168,#71169,#71170,#71171,
#71172,#71173,#71174,#71175,#71176,#71177,#71178,#71179,#71180,#71181,#71182,
#71183,#71184,#71185,#71186,#71187,#71188),.UNSPECIFIED.,.F.,.F.,(4,3,3,
3,3,3,3,4),(-104.624197634898,-103.912668501271,-102.913508227221,-101.91434795317,
-100.915187679119,-99.9160274050685,-98.9168671310179,-98.3410123277185),
 .UNSPECIFIED.);
#2945=B_SPLINE_CURVE_WITH_KNOTS('',3,(#71189,#71190,#71191,#71192,#71193,
#71194,#71195,#71196,#71197,#71198,#71199,#71200,#71201,#71202,#71203,#71204,
#71205,#71206,#71207,#71208,#71209,#71210),.UNSPECIFIED.,.F.,.F.,(4,3,3,
3,3,3,3,4),(95.377172011825,95.9193863088658,96.9185465829165,97.9177068569672,
98.9168671310178,99.9160274050685,100.915187679119,101.660357319005),
 .UNSPECIFIED.);
#2946=B_SPLINE_CURVE_WITH_KNOTS('',3,(#71215,#71216,#71217,#71218,#71219,
#71220,#71221,#71222,#71223,#71224,#71225,#71226,#71227,#71228,#71229,#71230,
#71231,#71232,#71233,#71234,#71235,#71236),.UNSPECIFIED.,.F.,.F.,(4,3,3,
3,3,3,3,4),(-110.907382942078,-109.907630145575,-108.908469871525,-107.909309597474,
-106.910149323423,-105.910989049373,-104.911828775322,-104.624197634898),
 .UNSPECIFIED.);
#2947=B_SPLINE_CURVE_WITH_KNOTS('',3,(#71237,#71238,#71239,#71240,#71241,
#71242,#71243,#71244,#71245,#71246,#71247,#71248,#71249,#71250,#71251,#71252,
#71253,#71254,#71255,#71256,#71257,#71258,#71259,#71260,#71261),
 .UNSPECIFIED.,.F.,.F.,(4,3,3,3,3,3,3,3,4),(101.660357319005,101.91434795317,
102.913508227221,103.912668501271,104.911828775322,105.910989049373,106.910149323423,
107.909309597474,107.943542626184),.UNSPECIFIED.);
#2948=B_SPLINE_CURVE_WITH_KNOTS('',3,(#71266,#71267,#71268,#71269,#71270,
#71271,#71272,#71273,#71274,#71275,#71276,#71277,#71278,#71279,#71280,#71281,
#71282,#71283,#71284,#71285,#71286,#71287),.UNSPECIFIED.,.F.,.F.,(4,3,3,
3,3,3,3,4),(-117.190568249257,-116.90175206393,-115.902591789879,-114.903431515829,
-113.904271241778,-112.905110967727,-111.905950693677,-110.907382942078),
 .UNSPECIFIED.);
#2949=B_SPLINE_CURVE_WITH_KNOTS('',3,(#71288,#71289,#71290,#71291,#71292,
#71293,#71294,#71295,#71296,#71297,#71298,#71299,#71300,#71301,#71302,#71303,
#71304,#71305,#71306,#71307,#71308,#71309),.UNSPECIFIED.,.F.,.F.,(4,3,3,
3,3,3,3,4),(107.943542626184,108.908469871525,109.907630145575,110.906790419626,
111.905950693677,112.905110967727,113.904271241778,114.226727933364),
 .UNSPECIFIED.);
#2950=B_SPLINE_CURVE_WITH_KNOTS('',3,(#71314,#71315,#71316,#71317,#71318,
#71319,#71320,#71321,#71322,#71323,#71324,#71325,#71326,#71327,#71328,#71329,
#71330,#71331,#71332,#71333,#71334,#71335),.UNSPECIFIED.,.F.,.F.,(4,3,3,
3,3,3,3,4),(-123.473753556437,-122.896713708234,-121.897553434184,-120.898393160133,
-119.899232886082,-118.900072612032,-117.900912337981,-117.190568249257),
 .UNSPECIFIED.);
#2951=B_SPLINE_CURVE_WITH_KNOTS('',3,(#71336,#71337,#71338,#71339,#71340,
#71341,#71342,#71343,#71344,#71345,#71346,#71347,#71348,#71349,#71350,#71351,
#71352,#71353,#71354,#71355,#71356,#71357),.UNSPECIFIED.,.F.,.F.,(4,3,3,
3,3,3,3,4),(114.226727933364,114.903431515829,115.90259178988,116.90175206393,
117.900912337981,118.900072612032,119.899232886082,120.509913240543),
 .UNSPECIFIED.);
#2952=B_SPLINE_CURVE_WITH_KNOTS('',3,(#71362,#71363,#71364,#71365,#71366,
#71367,#71368,#71369,#71370,#71371,#71372,#71373,#71374,#71375,#71376,#71377,
#71378,#71379,#71380,#71381,#71382,#71383),.UNSPECIFIED.,.F.,.F.,(4,3,3,
3,3,3,3,4),(-129.756938863617,-128.891675352538,-127.892515078488,-126.893354804437,
-125.894194530386,-124.895034256336,-123.895873982285,-123.473753556437),
 .UNSPECIFIED.);
#2953=B_SPLINE_CURVE_WITH_KNOTS('',3,(#71384,#71385,#71386,#71387,#71388,
#71389,#71390,#71391,#71392,#71393,#71394,#71395,#71396,#71397,#71398,#71399,
#71400,#71401,#71402,#71403,#71404,#71405),.UNSPECIFIED.,.F.,.F.,(4,3,3,
3,3,3,3,4),(120.509913240543,120.898393160133,121.897553434184,122.896713708234,
123.895873982285,124.895034256336,125.894194530386,126.793098547723),
 .UNSPECIFIED.);
#2954=B_SPLINE_CURVE_WITH_KNOTS('',3,(#71410,#71411,#71412,#71413,#71414,
#71415,#71416,#71417,#71418,#71419,#71420,#71421,#71422,#71423,#71424,#71425,
#71426,#71427,#71428,#71429,#71430,#71431,#71432,#71433,#71434),
 .UNSPECIFIED.,.F.,.F.,(4,3,3,3,3,3,3,3,4),(-136.040124170796,-135.885797270893,
-134.886636996842,-133.887476722792,-132.888316448741,-131.88915617469,
-130.88999590064,-129.890835626589,-129.756938863617),.UNSPECIFIED.);
#2955=B_SPLINE_CURVE_WITH_KNOTS('',3,(#71435,#71436,#71437,#71438,#71439,
#71440,#71441,#71442,#71443,#71444,#71445,#71446,#71447,#71448,#71449,#71450,
#71451,#71452,#71453,#71454,#71455,#71456,#71457,#71458,#71459),
 .UNSPECIFIED.,.F.,.F.,(4,3,3,3,3,3,3,3,4),(126.793098547723,126.893354804437,
127.892515078488,128.891675352538,129.890835626589,130.88999590064,131.88915617469,
132.888316448741,133.076283854902),.UNSPECIFIED.);
#2956=B_SPLINE_CURVE_WITH_KNOTS('',3,(#71464,#71465,#71466,#71467,#71468,
#71469,#71470,#71471,#71472,#71473,#71474,#71475,#71476,#71477,#71478,#71479,
#71480,#71481,#71482,#71483,#71484,#71485),.UNSPECIFIED.,.F.,.F.,(4,3,3,
3,3,3,3,4),(-142.323309477976,-141.880758915197,-140.881598641147,-139.882438367096,
-138.883278093045,-137.884117818995,-136.884957544944,-136.040124170796),
 .UNSPECIFIED.);
#2957=B_SPLINE_CURVE_WITH_KNOTS('',3,(#71486,#71487,#71488,#71489,#71490,
#71491,#71492,#71493,#71494,#71495,#71496,#71497,#71498,#71499,#71500,#71501,
#71502,#71503,#71504,#71505,#71506,#71507),.UNSPECIFIED.,.F.,.F.,(4,3,3,
3,3,3,3,4),(133.076283854902,133.887476722792,134.886636996843,135.885797270893,
136.884957544944,137.884117818995,138.883278093045,139.359469162082),
 .UNSPECIFIED.);
#2958=B_SPLINE_CURVE_WITH_KNOTS('',3,(#71512,#71513,#71514,#71515,#71516,
#71517,#71518,#71519,#71520,#71521,#71522,#71523,#71524,#71525,#71526,#71527,
#71528,#71529,#71530,#71531,#71532,#71533),.UNSPECIFIED.,.F.,.F.,(4,3,3,
3,3,3,3,4),(-148.606494785155,-147.875720559501,-146.876560285451,-145.8774000114,
-144.878239737349,-143.879079463299,-142.879919189248,-142.323309477976),
 .UNSPECIFIED.);
#2959=B_SPLINE_CURVE_WITH_KNOTS('',3,(#71534,#71535,#71536,#71537,#71538,
#71539,#71540,#71541,#71542,#71543,#71544,#71545,#71546,#71547,#71548,#71549,
#71550,#71551,#71552,#71553,#71554,#71555),.UNSPECIFIED.,.F.,.F.,(4,3,3,
3,3,3,3,4),(139.359469162082,139.882438367096,140.881598641147,141.880758915197,
142.879919189248,143.879079463299,144.878239737349,145.642654469262),
 .UNSPECIFIED.);
#2960=B_SPLINE_CURVE_WITH_KNOTS('',3,(#71560,#71561,#71562,#71563,#71564,
#71565,#71566,#71567,#71568,#71569,#71570,#71571,#71572,#71573,#71574,#71575,
#71576,#71577,#71578,#71579,#71580,#71581,#71582,#71583,#71584),
 .UNSPECIFIED.,.F.,.F.,(4,3,3,3,3,3,3,3,4),(-154.889680092335,-154.869842477856,
-153.870682203806,-152.871521929755,-151.872361655704,-150.873201381653,
-149.874041107603,-148.874880833552,-148.606494785155),.UNSPECIFIED.);
#2961=B_SPLINE_CURVE_WITH_KNOTS('',3,(#71585,#71586,#71587,#71588,#71589,
#71590,#71591,#71592,#71593,#71594,#71595,#71596,#71597,#71598,#71599,#71600,
#71601,#71602,#71603,#71604,#71605,#71606,#71607,#71608,#71609),
 .UNSPECIFIED.,.F.,.F.,(4,3,3,3,3,3,3,3,4),(145.642654469262,145.8774000114,
146.876560285451,147.875720559501,148.874880833552,149.874041107603,150.873201381653,
151.872361655704,151.925839776441),.UNSPECIFIED.);
#2962=B_SPLINE_CURVE_WITH_KNOTS('',3,(#71614,#71615,#71616,#71617,#71618,
#71619,#71620,#71621,#71622,#71623,#71624,#71625,#71626,#71627,#71628,#71629,
#71630,#71631,#71632,#71633,#71634,#71635),.UNSPECIFIED.,.F.,.F.,(4,3,3,
3,3,3,3,4),(-161.172865399514,-160.86480412216,-159.86564384811,-158.866483574059,
-157.867323300008,-156.868163025958,-155.869002751907,-154.889680092335),
 .UNSPECIFIED.);
#2963=B_SPLINE_CURVE_WITH_KNOTS('',3,(#71636,#71637,#71638,#71639,#71640,
#71641,#71642,#71643,#71644,#71645,#71646,#71647,#71648,#71649,#71650,#71651,
#71652,#71653,#71654,#71655,#71656,#71657),.UNSPECIFIED.,.F.,.F.,(4,3,3,
3,3,3,3,4),(151.925839776441,152.871521929755,153.870682203806,154.869842477856,
155.869002751907,156.868163025958,157.867323300008,158.209025083621),
 .UNSPECIFIED.);
#2964=B_SPLINE_CURVE_WITH_KNOTS('',3,(#71662,#71663,#71664,#71665,#71666,
#71667,#71668,#71669,#71670,#71671,#71672,#71673,#71674,#71675,#71676,#71677,
#71678,#71679,#71680,#71681,#71682,#71683),.UNSPECIFIED.,.F.,.F.,(4,3,3,
3,3,3,3,4),(-167.456050706694,-166.859765766464,-165.860605492414,-164.861445218363,
-163.862284944312,-162.863124670262,-161.863964396211,-161.172865399514),
 .UNSPECIFIED.);
#2965=B_SPLINE_CURVE_WITH_KNOTS('',3,(#71684,#71685,#71686,#71687,#71688,
#71689,#71690,#71691,#71692,#71693,#71694,#71695,#71696,#71697,#71698,#71699,
#71700,#71701,#71702,#71703,#71704,#71705),.UNSPECIFIED.,.F.,.F.,(4,3,3,
3,3,3,3,4),(158.209025083621,158.866483574059,159.86564384811,160.86480412216,
161.863964396211,162.863124670262,163.862284944312,164.4922103908),
 .UNSPECIFIED.);
#2966=B_SPLINE_CURVE_WITH_KNOTS('',3,(#71710,#71711,#71712,#71713,#71714,
#71715,#71716,#71717,#71718,#71719,#71720,#71721,#71722,#71723,#71724,#71725,
#71726,#71727,#71728,#71729,#71730,#71731),.UNSPECIFIED.,.F.,.F.,(4,3,3,
3,3,3,3,4),(-173.739236013873,-172.854727410769,-171.855567136718,-170.856406862667,
-169.857246588616,-168.858086314566,-167.858926040515,-167.456050706694),
 .UNSPECIFIED.);
#2967=B_SPLINE_CURVE_WITH_KNOTS('',3,(#71732,#71733,#71734,#71735,#71736,
#71737,#71738,#71739,#71740,#71741,#71742,#71743,#71744,#71745,#71746,#71747,
#71748,#71749,#71750,#71751,#71752,#71753),.UNSPECIFIED.,.F.,.F.,(4,3,3,
3,3,3,3,4),(164.4922103908,164.861445218363,165.860605492414,166.859765766465,
167.858926040515,168.858086314566,169.857246588617,170.77539569798),
 .UNSPECIFIED.);
#2968=B_SPLINE_CURVE_WITH_KNOTS('',3,(#71758,#71759,#71760,#71761,#71762,
#71763,#71764,#71765,#71766,#71767,#71768,#71769,#71770,#71771,#71772,#71773,
#71774,#71775,#71776,#71777,#71778,#71779,#71780,#71781,#71782),
 .UNSPECIFIED.,.F.,.F.,(4,3,3,3,3,3,3,3,4),(-180.022421321053,-179.848849329123,
-178.849689055073,-177.850528781022,-176.851368506971,-175.852208232921,
-174.85304795887,-173.853887684819,-173.739236013873),.UNSPECIFIED.);
#2969=B_SPLINE_CURVE_WITH_KNOTS('',3,(#71783,#71784,#71785,#71786,#71787,
#71788,#71789,#71790,#71791,#71792,#71793,#71794,#71795,#71796,#71797,#71798,
#71799,#71800,#71801,#71802,#71803,#71804,#71805,#71806,#71807),
 .UNSPECIFIED.,.F.,.F.,(4,3,3,3,3,3,3,3,4),(170.77539569798,170.856406862667,
171.855567136718,172.854727410769,173.853887684819,174.85304795887,175.852208232921,
176.851368506971,177.058581005159),.UNSPECIFIED.);
#2970=B_SPLINE_CURVE_WITH_KNOTS('',3,(#71812,#71813,#71814,#71815,#71816,
#71817,#71818,#71819,#71820,#71821,#71822,#71823,#71824,#71825,#71826,#71827,
#71828,#71829,#71830,#71831,#71832,#71833),.UNSPECIFIED.,.F.,.F.,(4,3,3,
3,3,3,3,4),(-186.305606628233,-185.843810973427,-184.844650699377,-183.845490425326,
-182.846330151275,-181.847169877225,-180.848009603174,-180.022421321053),
 .UNSPECIFIED.);
#2971=B_SPLINE_CURVE_WITH_KNOTS('',3,(#71834,#71835,#71836,#71837,#71838,
#71839,#71840,#71841,#71842,#71843,#71844,#71845,#71846,#71847,#71848,#71849,
#71850,#71851,#71852,#71853,#71854,#71855),.UNSPECIFIED.,.F.,.F.,(4,3,3,
3,3,3,3,4),(177.058581005159,177.850528781022,178.849689055073,179.848849329123,
180.848009603174,181.847169877225,182.846330151275,183.341766312339),
 .UNSPECIFIED.);
#2972=B_SPLINE_CURVE_WITH_KNOTS('',3,(#71860,#71861,#71862,#71863,#71864,
#71865,#71866,#71867,#71868,#71869,#71870,#71871,#71872,#71873,#71874,#71875,
#71876,#71877,#71878,#71879,#71880,#71881),.UNSPECIFIED.,.F.,.F.,(4,3,3,
3,3,3,3,4),(-192.588791935412,-191.838772617732,-190.839612343681,-189.84045206963,
-188.841291795579,-187.842131521529,-186.842971247478,-186.305606628233),
 .UNSPECIFIED.);
#2973=B_SPLINE_CURVE_WITH_KNOTS('',3,(#71882,#71883,#71884,#71885,#71886,
#71887,#71888,#71889,#71890,#71891,#71892,#71893,#71894,#71895,#71896,#71897,
#71898,#71899,#71900,#71901,#71902,#71903),.UNSPECIFIED.,.F.,.F.,(4,3,3,
3,3,3,3,4),(183.341766312339,183.845490425326,184.844650699377,185.843810973427,
186.842971247478,187.842131521529,188.84129179558,189.624951619519),
 .UNSPECIFIED.);
#2974=B_SPLINE_CURVE_WITH_KNOTS('',3,(#71908,#71909,#71910,#71911,#71912,
#71913,#71914,#71915,#71916,#71917,#71918,#71919,#71920,#71921,#71922,#71923,
#71924,#71925,#71926,#71927,#71928,#71929,#71930,#71931,#71932),
 .UNSPECIFIED.,.F.,.F.,(4,3,3,3,3,3,3,3,4),(-198.871977242592,-198.832894536086,
-197.833734262036,-196.834573987985,-195.835413713934,-194.836253439884,
-193.837093165833,-192.837932891782,-192.588791935412),.UNSPECIFIED.);
#2975=B_SPLINE_CURVE_WITH_KNOTS('',3,(#71933,#71934,#71935,#71936,#71937,
#71938,#71939,#71940,#71941,#71942,#71943,#71944,#71945,#71946,#71947,#71948,
#71949,#71950,#71951,#71952,#71953,#71954,#71955,#71956,#71957),
 .UNSPECIFIED.,.F.,.F.,(4,3,3,3,3,3,3,3,4),(189.624951619519,189.84045206963,
190.839612343681,191.838772617732,192.837932891782,193.837093165833,194.836253439884,
195.835413713934,195.908136926698),.UNSPECIFIED.);
#2976=B_SPLINE_CURVE_WITH_KNOTS('',3,(#71962,#71963,#71964,#71965,#71966,
#71967,#71968,#71969,#71970,#71971,#71972,#71973,#71974,#71975,#71976,#71977,
#71978,#71979,#71980,#71981,#71982,#71983),.UNSPECIFIED.,.F.,.F.,(4,3,3,
3,3,3,3,4),(-205.155162549771,-204.82785618039,-203.82869590634,-202.829535632289,
-201.830375358238,-200.831215084188,-199.832054810137,-198.871977242592),
 .UNSPECIFIED.);
#2977=B_SPLINE_CURVE_WITH_KNOTS('',3,(#71984,#71985,#71986,#71987,#71988,
#71989,#71990,#71991,#71992,#71993,#71994,#71995,#71996,#71997,#71998,#71999,
#72000,#72001,#72002,#72003,#72004,#72005),.UNSPECIFIED.,.F.,.F.,(4,3,3,
3,3,3,3,4),(195.908136926698,196.834573987985,197.833734262036,198.832894536086,
199.832054810137,200.831215084188,201.830375358238,202.191322233878),
 .UNSPECIFIED.);
#2978=B_SPLINE_CURVE_WITH_KNOTS('',3,(#72010,#72011,#72012,#72013,#72014,
#72015,#72016,#72017,#72018,#72019,#72020,#72021,#72022,#72023,#72024,#72025,
#72026,#72027,#72028,#72029,#72030,#72031),.UNSPECIFIED.,.F.,.F.,(4,3,3,
3,3,3,3,4),(-211.438347856951,-210.822817824695,-209.823657550644,-208.824497276593,
-207.825337002543,-206.826176728492,-205.827016454441,-205.155162549771),
 .UNSPECIFIED.);
#2979=B_SPLINE_CURVE_WITH_KNOTS('',3,(#72032,#72033,#72034,#72035,#72036,
#72037,#72038,#72039,#72040,#72041,#72042,#72043,#72044,#72045,#72046,#72047,
#72048,#72049,#72050,#72051,#72052,#72053),.UNSPECIFIED.,.F.,.F.,(4,3,3,
3,3,3,3,4),(202.191322233878,202.829535632289,203.82869590634,204.82785618039,
205.827016454441,206.826176728492,207.825337002543,208.474507541057),
 .UNSPECIFIED.);
#2980=B_SPLINE_CURVE_WITH_KNOTS('',3,(#72058,#72059,#72060,#72061,#72062,
#72063,#72064,#72065,#72066,#72067,#72068,#72069,#72070,#72071,#72072,#72073,
#72074,#72075,#72076,#72077,#72078,#72079),.UNSPECIFIED.,.F.,.F.,(4,3,3,
3,3,3,3,4),(-217.72153316413,-216.817779468999,-215.818619194948,-214.819458920897,
-213.820298646847,-212.821138372796,-211.821978098745,-211.438347856951),
 .UNSPECIFIED.);
#2981=B_SPLINE_CURVE_WITH_KNOTS('',3,(#72080,#72081,#72082,#72083,#72084,
#72085,#72086,#72087,#72088,#72089,#72090,#72091,#72092,#72093,#72094,#72095,
#72096,#72097,#72098,#72099,#72100,#72101),.UNSPECIFIED.,.F.,.F.,(4,3,3,
3,3,3,3,4),(208.474507541057,208.824497276593,209.823657550644,210.822817824695,
211.821978098745,212.821138372796,213.820298646847,214.757692848237),
 .UNSPECIFIED.);
#2982=B_SPLINE_CURVE_WITH_KNOTS('',3,(#72106,#72107,#72108,#72109,#72110,
#72111,#72112,#72113,#72114,#72115,#72116,#72117,#72118,#72119,#72120,#72121,
#72122,#72123,#72124,#72125,#72126,#72127,#72128,#72129,#72130),
 .UNSPECIFIED.,.F.,.F.,(4,3,3,3,3,3,3,3,4),(-224.00471847131,-223.811901387354,
-222.812741113303,-221.813580839252,-220.814420565201,-219.815260291151,
-218.8161000171,-217.816939743049,-217.72153316413),.UNSPECIFIED.);
#2983=B_SPLINE_CURVE_WITH_KNOTS('',3,(#72131,#72132,#72133,#72134,#72135,
#72136,#72137,#72138,#72139,#72140,#72141,#72142,#72143,#72144,#72145,#72146,
#72147,#72148,#72149,#72150,#72151,#72152,#72153,#72154,#72155),
 .UNSPECIFIED.,.F.,.F.,(4,3,3,3,3,3,3,3,4),(214.757692848237,214.819458920897,
215.818619194948,216.817779468999,217.816939743049,218.8161000171,219.815260291151,
220.814420565201,221.040878155416),.UNSPECIFIED.);
#2984=B_SPLINE_CURVE_WITH_KNOTS('',3,(#72160,#72161,#72162,#72163,#72164,
#72165,#72166,#72167,#72168,#72169,#72170,#72171,#72172,#72173,#72174,#72175,
#72176,#72177,#72178,#72179,#72180,#72181),.UNSPECIFIED.,.F.,.F.,(4,3,3,
3,3,3,3,4),(-230.287903778489,-229.806863031658,-228.807702757607,-227.808542483556,
-226.809382209506,-225.810221935455,-224.811061661404,-224.00471847131),
 .UNSPECIFIED.);
#2985=B_SPLINE_CURVE_WITH_KNOTS('',3,(#72182,#72183,#72184,#72185,#72186,
#72187,#72188,#72189,#72190,#72191,#72192,#72193,#72194,#72195,#72196,#72197,
#72198,#72199,#72200,#72201,#72202,#72203),.UNSPECIFIED.,.F.,.F.,(4,3,3,
3,3,3,3,4),(221.040878155416,221.813580839252,222.812741113303,223.811901387354,
224.811061661404,225.810221935455,226.809382209506,227.324063462596),
 .UNSPECIFIED.);
#2986=B_SPLINE_CURVE_WITH_KNOTS('',3,(#72208,#72209,#72210,#72211,#72212,
#72213,#72214,#72215,#72216,#72217,#72218,#72219,#72220,#72221,#72222,#72223,
#72224,#72225,#72226,#72227,#72228,#72229),.UNSPECIFIED.,.F.,.F.,(4,3,3,
3,3,3,3,4),(-236.571089085669,-235.801824675962,-234.802664401911,-233.80350412786,
-232.80434385381,-231.805183579759,-230.806023305708,-230.287903778489),
 .UNSPECIFIED.);
#2987=B_SPLINE_CURVE_WITH_KNOTS('',3,(#72230,#72231,#72232,#72233,#72234,
#72235,#72236,#72237,#72238,#72239,#72240,#72241,#72242,#72243,#72244,#72245,
#72246,#72247,#72248,#72249,#72250,#72251),.UNSPECIFIED.,.F.,.F.,(4,3,3,
3,3,3,3,4),(227.324063462596,227.808542483556,228.807702757607,229.806863031658,
230.806023305708,231.805183579759,232.80434385381,233.607248769776),
 .UNSPECIFIED.);
#2988=B_SPLINE_CURVE_WITH_KNOTS('',3,(#72256,#72257,#72258,#72259,#72260,
#72261,#72262,#72263,#72264,#72265,#72266,#72267,#72268,#72269,#72270,#72271,
#72272,#72273,#72274,#72275,#72276,#72277,#72278,#72279,#72280),
 .UNSPECIFIED.,.F.,.F.,(4,3,3,3,3,3,3,3,4),(-242.854274392849,-242.795946594317,
-241.796786320266,-240.797626046215,-239.798465772164,-238.799305498114,
-237.800145224063,-236.800984950012,-236.571089085669),.UNSPECIFIED.);
#2989=B_SPLINE_CURVE_WITH_KNOTS('',3,(#72281,#72282,#72283,#72284,#72285,
#72286,#72287,#72288,#72289,#72290,#72291,#72292,#72293,#72294,#72295,#72296,
#72297,#72298,#72299,#72300,#72301,#72302,#72303,#72304,#72305),
 .UNSPECIFIED.,.F.,.F.,(4,3,3,3,3,3,3,3,4),(233.607248769776,233.80350412786,
234.802664401911,235.801824675962,236.800984950012,237.800145224063,238.799305498114,
239.798465772164,239.890434076955),.UNSPECIFIED.);
#2990=B_SPLINE_CURVE_WITH_KNOTS('',3,(#72310,#72311,#72312,#72313,#72314,
#72315,#72316,#72317,#72318,#72319,#72320,#72321,#72322,#72323,#72324,#72325,
#72326,#72327,#72328,#72329,#72330,#72331),.UNSPECIFIED.,.F.,.F.,(4,3,3,
3,3,3,3,4),(-249.137459700028,-248.790908238621,-247.79174796457,-246.792587690519,
-245.793427416469,-244.794267142418,-243.795106868367,-242.854274392849),
 .UNSPECIFIED.);
#2991=B_SPLINE_CURVE_WITH_KNOTS('',3,(#72332,#72333,#72334,#72335,#72336,
#72337,#72338,#72339,#72340,#72341,#72342,#72343,#72344,#72345,#72346,#72347,
#72348,#72349,#72350,#72351,#72352,#72353),.UNSPECIFIED.,.F.,.F.,(4,3,3,
3,3,3,3,4),(239.890434076955,240.797626046215,241.796786320266,242.795946594317,
243.795106868367,244.794267142418,245.793427416469,246.173619384135),
 .UNSPECIFIED.);
#2992=B_SPLINE_CURVE_WITH_KNOTS('',3,(#72358,#72359,#72360,#72361,#72362,
#72363,#72364,#72365,#72366,#72367,#72368,#72369,#72370,#72371,#72372,#72373,
#72374,#72375,#72376,#72377,#72378,#72379),.UNSPECIFIED.,.F.,.F.,(4,3,3,
3,3,3,3,4),(-255.420645007208,-254.785869882925,-253.786709608874,-252.787549334823,
-251.788389060773,-250.789228786722,-249.790068512671,-249.137459700028),
 .UNSPECIFIED.);
#2993=B_SPLINE_CURVE_WITH_KNOTS('',3,(#72380,#72381,#72382,#72383,#72384,
#72385,#72386,#72387,#72388,#72389,#72390,#72391,#72392,#72393,#72394,#72395,
#72396,#72397,#72398,#72399,#72400,#72401),.UNSPECIFIED.,.F.,.F.,(4,3,3,
3,3,3,3,4),(246.173619384135,246.792587690519,247.79174796457,248.790908238621,
249.790068512671,250.789228786722,251.788389060773,252.456804691314),
 .UNSPECIFIED.);
#2994=B_SPLINE_CURVE_WITH_KNOTS('',3,(#72406,#72407,#72408,#72409,#72410,
#72411,#72412,#72413,#72414,#72415,#72416,#72417,#72418,#72419,#72420,#72421,
#72422,#72423,#72424,#72425,#72426,#72427),.UNSPECIFIED.,.F.,.F.,(4,3,3,
3,3,3,3,4),(-261.703830314387,-260.780831527229,-259.781671253178,-258.782510979127,
-257.783350705077,-256.784190431026,-255.785030156975,-255.420645007208),
 .UNSPECIFIED.);
#2995=B_SPLINE_CURVE_WITH_KNOTS('',3,(#72428,#72429,#72430,#72431,#72432,
#72433,#72434,#72435,#72436,#72437,#72438,#72439,#72440,#72441,#72442,#72443,
#72444,#72445,#72446,#72447,#72448,#72449),.UNSPECIFIED.,.F.,.F.,(4,3,3,
3,3,3,3,4),(252.456804691314,252.787549334823,253.786709608874,254.785869882925,
255.785030156975,256.784190431026,257.783350705077,258.739989998494),
 .UNSPECIFIED.);
#2996=B_SPLINE_CURVE_WITH_KNOTS('',3,(#72454,#72455,#72456,#72457,#72458,
#72459,#72460,#72461,#72462,#72463,#72464,#72465,#72466,#72467,#72468,#72469,
#72470,#72471,#72472,#72473,#72474,#72475,#72476,#72477,#72478),
 .UNSPECIFIED.,.F.,.F.,(4,3,3,3,3,3,3,3,4),(-267.987015621567,-267.774953445584,
-266.775793171533,-265.776632897482,-264.777472623432,-263.778312349381,
-262.77915207533,-261.77999180128,-261.703830314387),.UNSPECIFIED.);
#2997=B_SPLINE_CURVE_WITH_KNOTS('',3,(#72479,#72480,#72481,#72482,#72483,
#72484,#72485,#72486,#72487,#72488,#72489,#72490,#72491,#72492,#72493,#72494,
#72495,#72496,#72497,#72498,#72499,#72500,#72501,#72502,#72503),
 .UNSPECIFIED.,.F.,.F.,(4,3,3,3,3,3,3,3,4),(258.739989998494,258.782510979128,
259.781671253178,260.780831527229,261.77999180128,262.77915207533,263.778312349381,
264.777472623432,265.023175305673),.UNSPECIFIED.);
#2998=B_SPLINE_CURVE_WITH_KNOTS('',3,(#72508,#72509,#72510,#72511,#72512,
#72513,#72514,#72515,#72516,#72517,#72518,#72519,#72520,#72521,#72522,#72523,
#72524,#72525,#72526,#72527,#72528,#72529),.UNSPECIFIED.,.F.,.F.,(4,3,3,
3,3,3,3,4),(-274.270200928747,-273.769915089888,-272.770754815837,-271.771594541786,
-270.772434267736,-269.773273993685,-268.774113719634,-267.987015621567),
 .UNSPECIFIED.);
#2999=B_SPLINE_CURVE_WITH_KNOTS('',3,(#72530,#72531,#72532,#72533,#72534,
#72535,#72536,#72537,#72538,#72539,#72540,#72541,#72542,#72543,#72544,#72545,
#72546,#72547,#72548,#72549,#72550,#72551),.UNSPECIFIED.,.F.,.F.,(4,3,3,
3,3,3,3,4),(265.023175305673,265.776632897482,266.775793171533,267.774953445584,
268.774113719634,269.773273993685,270.772434267736,271.306360612853),
 .UNSPECIFIED.);
#3000=B_SPLINE_CURVE_WITH_KNOTS('',3,(#72556,#72557,#72558,#72559,#72560,
#72561,#72562,#72563,#72564,#72565,#72566,#72567,#72568,#72569,#72570,#72571,
#72572,#72573,#72574,#72575,#72576,#72577),.UNSPECIFIED.,.F.,.F.,(4,3,3,
3,3,3,3,4),(-280.553386235926,-279.764876734192,-278.765716460141,-277.76655618609,
-276.76739591204,-275.768235637989,-274.769075363938,-274.270200928747),
 .UNSPECIFIED.);
#3001=B_SPLINE_CURVE_WITH_KNOTS('',3,(#72578,#72579,#72580,#72581,#72582,
#72583,#72584,#72585,#72586,#72587,#72588,#72589,#72590,#72591,#72592,#72593,
#72594,#72595,#72596,#72597,#72598,#72599),.UNSPECIFIED.,.F.,.F.,(4,3,3,
3,3,3,3,4),(271.306360612853,271.771594541786,272.770754815837,273.769915089888,
274.769075363938,275.768235637989,276.76739591204,277.589545920032),
 .UNSPECIFIED.);
#3002=B_SPLINE_CURVE_WITH_KNOTS('',3,(#72604,#72605,#72606,#72607,#72608,
#72609,#72610,#72611,#72612,#72613,#72614,#72615,#72616,#72617,#72618,#72619,
#72620,#72621,#72622,#72623,#72624,#72625,#72626,#72627,#72628),
 .UNSPECIFIED.,.F.,.F.,(4,3,3,3,3,3,3,3,4),(-286.836571543106,-286.758998652547,
-285.759838378496,-284.760678104445,-283.761517830395,-282.762357556344,
-281.763197282293,-280.764037008243,-280.553386235926),.UNSPECIFIED.);
#3003=B_SPLINE_CURVE_WITH_KNOTS('',3,(#72629,#72630,#72631,#72632,#72633,
#72634,#72635,#72636,#72637,#72638,#72639,#72640,#72641,#72642,#72643,#72644,
#72645,#72646,#72647,#72648,#72649,#72650,#72651,#72652,#72653),
 .UNSPECIFIED.,.F.,.F.,(4,3,3,3,3,3,3,3,4),(277.589545920032,277.766556186091,
278.765716460141,279.764876734192,280.764037008243,281.763197282293,282.762357556344,
283.761517830395,283.872731227212),.UNSPECIFIED.);
#3004=B_SPLINE_CURVE_WITH_KNOTS('',3,(#72658,#72659,#72660,#72661,#72662,
#72663,#72664,#72665,#72666,#72667,#72668,#72669,#72670,#72671,#72672,#72673,
#72674,#72675,#72676,#72677,#72678,#72679),.UNSPECIFIED.,.F.,.F.,(4,3,3,
3,3,3,3,4),(-293.119756850285,-292.753960296851,-291.7548000228,-290.755639748749,
-289.756479474699,-288.757319200648,-287.758158926597,-286.836571543106),
 .UNSPECIFIED.);
#3005=B_SPLINE_CURVE_WITH_KNOTS('',3,(#72680,#72681,#72682,#72683,#72684,
#72685,#72686,#72687,#72688,#72689,#72690,#72691,#72692,#72693,#72694,#72695,
#72696,#72697,#72698,#72699,#72700,#72701),.UNSPECIFIED.,.F.,.F.,(4,3,3,
3,3,3,3,4),(283.872731227212,284.760678104445,285.759838378496,286.758998652547,
287.758158926597,288.757319200648,289.756479474699,290.155916534392),
 .UNSPECIFIED.);
#3006=B_SPLINE_CURVE_WITH_KNOTS('',3,(#72706,#72707,#72708,#72709,#72710,
#72711,#72712,#72713,#72714,#72715,#72716,#72717,#72718,#72719,#72720,#72721,
#72722,#72723,#72724,#72725,#72726,#72727),.UNSPECIFIED.,.F.,.F.,(4,3,3,
3,3,3,3,4),(-299.402942157465,-298.748921941155,-297.749761667104,-296.750601393054,
-295.751441119003,-294.752280844952,-293.753120570902,-293.119756850285),
 .UNSPECIFIED.);
#3007=B_SPLINE_CURVE_WITH_KNOTS('',3,(#72728,#72729,#72730,#72731,#72732,
#72733,#72734,#72735,#72736,#72737,#72738,#72739,#72740,#72741,#72742,#72743,
#72744,#72745,#72746,#72747,#72748,#72749),.UNSPECIFIED.,.F.,.F.,(4,3,3,
3,3,3,3,4),(290.155916534392,290.755639748749,291.7548000228,292.753960296851,
293.753120570902,294.752280844952,295.751441119003,296.439101841571),
 .UNSPECIFIED.);
#3008=B_SPLINE_CURVE_WITH_KNOTS('',3,(#72754,#72755,#72756,#72757,#72758,
#72759,#72760,#72761,#72762,#72763,#72764,#72765,#72766,#72767,#72768,#72769,
#72770,#72771,#72772,#72773,#72774,#72775),.UNSPECIFIED.,.F.,.F.,(4,3,3,
3,3,3,3,4),(-305.686127464644,-304.743883585459,-303.744723311408,-302.745563037358,
-301.746402763307,-300.747242489256,-299.748082215206,-299.402942157465),
 .UNSPECIFIED.);
#3009=B_SPLINE_CURVE_WITH_KNOTS('',3,(#72776,#72777,#72778,#72779,#72780,
#72781,#72782,#72783,#72784,#72785,#72786,#72787,#72788,#72789,#72790,#72791,
#72792,#72793,#72794,#72795,#72796,#72797),.UNSPECIFIED.,.F.,.F.,(4,3,3,
3,3,3,3,4),(296.439101841571,296.750601393054,297.749761667104,298.748921941155,
299.748082215206,300.747242489256,301.746402763307,302.722287148751),
 .UNSPECIFIED.);
#3010=B_SPLINE_CURVE_WITH_KNOTS('',3,(#72802,#72803,#72804,#72805,#72806,
#72807,#72808,#72809,#72810,#72811,#72812,#72813,#72814,#72815,#72816,#72817,
#72818,#72819,#72820,#72821,#72822,#72823,#72824,#72825,#72826),
 .UNSPECIFIED.,.F.,.F.,(4,3,3,3,3,3,3,3,4),(-311.969312771824,-311.738005503814,
-310.738845229763,-309.739684955712,-308.740524681662,-307.741364407611,
-306.74220413356,-305.74304385951,-305.686127464644),.UNSPECIFIED.);
#3011=B_SPLINE_CURVE_WITH_KNOTS('',3,(#72827,#72828,#72829,#72830,#72831,
#72832,#72833,#72834,#72835,#72836,#72837,#72838,#72839,#72840,#72841,#72842,
#72843,#72844,#72845,#72846,#72847,#72848,#72849,#72850,#72851),
 .UNSPECIFIED.,.F.,.F.,(4,3,3,3,3,3,3,3,4),(302.722287148751,302.745563037358,
303.744723311408,304.743883585459,305.74304385951,306.74220413356,307.741364407611,
308.740524681662,309.00547245593),.UNSPECIFIED.);
#3012=B_SPLINE_CURVE_WITH_KNOTS('',3,(#72856,#72857,#72858,#72859,#72860,
#72861,#72862,#72863,#72864,#72865,#72866,#72867,#72868,#72869,#72870,#72871,
#72872,#72873,#72874,#72875,#72876,#72877),.UNSPECIFIED.,.F.,.F.,(4,3,3,
3,3,3,3,4),(-318.252498079003,-317.732967148118,-316.733806874067,-315.734646600017,
-314.735486325966,-313.736326051915,-312.737165777864,-311.969312771824),
 .UNSPECIFIED.);
#3013=B_SPLINE_CURVE_WITH_KNOTS('',3,(#72878,#72879,#72880,#72881,#72882,
#72883,#72884,#72885,#72886,#72887,#72888,#72889,#72890,#72891,#72892,#72893,
#72894,#72895,#72896,#72897,#72898,#72899),.UNSPECIFIED.,.F.,.F.,(4,3,3,
3,3,3,3,4),(309.00547245593,309.739684955712,310.738845229763,311.738005503814,
312.737165777865,313.736326051915,314.735486325966,315.28865776311),
 .UNSPECIFIED.);
#3014=B_SPLINE_CURVE_WITH_KNOTS('',3,(#72904,#72905,#72906,#72907,#72908,
#72909,#72910,#72911,#72912,#72913,#72914,#72915,#72916,#72917,#72918,#72919,
#72920,#72921,#72922,#72923,#72924,#72925),.UNSPECIFIED.,.F.,.F.,(4,3,3,
3,3,3,3,4),(-324.535683386183,-323.727928792422,-322.728768518371,-321.729608244321,
-320.73044797027,-319.731287696219,-318.732127422169,-318.252498079003),
 .UNSPECIFIED.);
#3015=B_SPLINE_CURVE_WITH_KNOTS('',3,(#72926,#72927,#72928,#72929,#72930,
#72931,#72932,#72933,#72934,#72935,#72936,#72937,#72938,#72939,#72940,#72941,
#72942,#72943,#72944,#72945,#72946,#72947),.UNSPECIFIED.,.F.,.F.,(4,3,3,
3,3,3,3,4),(315.28865776311,315.734646600017,316.733806874067,317.732967148118,
318.732127422169,319.731287696219,320.73044797027,321.571843070289),
 .UNSPECIFIED.);
#3016=B_SPLINE_CURVE_WITH_KNOTS('',3,(#72952,#72953,#72954,#72955,#72956,
#72957,#72958,#72959,#72960,#72961,#72962,#72963,#72964,#72965,#72966,#72967,
#72968,#72969,#72970,#72971,#72972,#72973,#72974,#72975,#72976),
 .UNSPECIFIED.,.F.,.F.,(4,3,3,3,3,3,3,3,4),(-330.818868693363,-330.722050710777,
-329.722890436726,-328.723730162676,-327.724569888625,-326.725409614574,
-325.726249340523,-324.727089066473,-324.535683386183),.UNSPECIFIED.);
#3017=B_SPLINE_CURVE_WITH_KNOTS('',3,(#72977,#72978,#72979,#72980,#72981,
#72982,#72983,#72984,#72985,#72986,#72987,#72988,#72989,#72990,#72991,#72992,
#72993,#72994,#72995,#72996,#72997,#72998,#72999,#73000,#73001),
 .UNSPECIFIED.,.F.,.F.,(4,3,3,3,3,3,3,3,4),(321.571843070289,321.729608244321,
322.728768518371,323.727928792422,324.727089066473,325.726249340523,326.725409614574,
327.724569888625,327.855028377469),.UNSPECIFIED.);
#3018=B_SPLINE_CURVE_WITH_KNOTS('',3,(#73006,#73007,#73008,#73009,#73010,
#73011,#73012,#73013,#73014,#73015,#73016,#73017,#73018,#73019,#73020,#73021,
#73022,#73023,#73024,#73025,#73026,#73027),.UNSPECIFIED.,.F.,.F.,(4,3,3,
3,3,3,3,4),(-337.102054000542,-336.717012355081,-335.71785208103,-334.71869180698,
-333.719531532929,-332.720371258878,-331.721210984828,-330.818868693363),
 .UNSPECIFIED.);
#3019=B_SPLINE_CURVE_WITH_KNOTS('',3,(#73028,#73029,#73030,#73031,#73032,
#73033,#73034,#73035,#73036,#73037,#73038,#73039,#73040,#73041,#73042,#73043,
#73044,#73045,#73046,#73047,#73048,#73049),.UNSPECIFIED.,.F.,.F.,(4,3,3,
3,3,3,3,4),(327.855028377469,328.723730162675,329.722890436726,330.722050710777,
331.721210984828,332.720371258878,333.719531532929,334.138213684649),
 .UNSPECIFIED.);
#3020=B_SPLINE_CURVE_WITH_KNOTS('',3,(#73054,#73055,#73056,#73057,#73058,
#73059,#73060,#73061,#73062,#73063,#73064,#73065,#73066,#73067,#73068,#73069,
#73070,#73071,#73072,#73073,#73074,#73075),.UNSPECIFIED.,.F.,.F.,(4,3,3,
3,3,3,3,4),(-343.385239307722,-342.711973999385,-341.712813725334,-340.713653451284,
-339.714493177233,-338.715332903182,-337.716172629132,-337.102054000542),
 .UNSPECIFIED.);
#3021=B_SPLINE_CURVE_WITH_KNOTS('',3,(#73076,#73077,#73078,#73079,#73080,
#73081,#73082,#73083,#73084,#73085,#73086,#73087,#73088,#73089,#73090,#73091,
#73092,#73093,#73094,#73095,#73096,#73097),.UNSPECIFIED.,.F.,.F.,(4,3,3,
3,3,3,3,4),(334.138213684649,334.71869180698,335.71785208103,336.717012355081,
337.716172629132,338.715332903182,339.714493177233,340.421398991828),
 .UNSPECIFIED.);
#3022=B_SPLINE_CURVE_WITH_KNOTS('',3,(#73102,#73103,#73104,#73105,#73106,
#73107,#73108,#73109,#73110,#73111,#73112,#73113,#73114,#73115,#73116,#73117,
#73118,#73119,#73120,#73121,#73122,#73123),.UNSPECIFIED.,.F.,.F.,(4,3,3,
3,3,3,3,4),(-349.668424614901,-348.706935643689,-347.707775369639,-346.708615095588,
-345.709454821537,-344.710294547486,-343.711134273436,-343.385239307722),
 .UNSPECIFIED.);
#3023=B_SPLINE_CURVE_WITH_KNOTS('',3,(#73124,#73125,#73126,#73127,#73128,
#73129,#73130,#73131,#73132,#73133,#73134,#73135,#73136,#73137,#73138,#73139,
#73140,#73141,#73142,#73143,#73144,#73145),.UNSPECIFIED.,.F.,.F.,(4,3,3,
3,3,3,3,4),(340.421398991828,340.713653451284,341.712813725334,342.711973999385,
343.711134273436,344.710294547487,345.709454821537,346.704584299008),
 .UNSPECIFIED.);
#3024=B_SPLINE_CURVE_WITH_KNOTS('',3,(#73150,#73151,#73152,#73153,#73154,
#73155,#73156,#73157,#73158,#73159,#73160,#73161,#73162,#73163,#73164,#73165,
#73166,#73167,#73168,#73169,#73170,#73171,#73172,#73173,#73174),
 .UNSPECIFIED.,.F.,.F.,(4,3,3,3,3,3,3,3,4),(-355.951609922081,-355.701057562044,
-354.701897287993,-353.702737013943,-352.703576739892,-351.704416465841,
-350.705256191791,-349.70609591774,-349.668424614901),.UNSPECIFIED.);
#3025=B_SPLINE_CURVE_WITH_KNOTS('',3,(#73175,#73176,#73177,#73178,#73179,
#73180,#73181,#73182,#73183,#73184,#73185,#73186,#73187,#73188,#73189,#73190,
#73191,#73192,#73193,#73194,#73195,#73196,#73197,#73198,#73199),
 .UNSPECIFIED.,.F.,.F.,(4,3,3,3,3,3,3,3,4),(346.704584299008,346.708615095588,
347.707775369639,348.706935643689,349.70609591774,350.705256191791,351.704416465841,
352.703576739892,352.987769606187),.UNSPECIFIED.);
#3026=B_SPLINE_CURVE_WITH_KNOTS('',3,(#73204,#73205,#73206,#73207,#73208,
#73209,#73210,#73211,#73212,#73213,#73214,#73215,#73216,#73217,#73218,#73219,
#73220,#73221,#73222,#73223,#73224,#73225),.UNSPECIFIED.,.F.,.F.,(4,3,3,
3,3,3,3,4),(-362.23479522926,-361.696019206348,-360.696858932297,-359.697698658247,
-358.698538384196,-357.699378110145,-356.700217836095,-355.951609922081),
 .UNSPECIFIED.);
#3027=B_SPLINE_CURVE_WITH_KNOTS('',3,(#73226,#73227,#73228,#73229,#73230,
#73231,#73232,#73233,#73234,#73235,#73236,#73237,#73238,#73239,#73240,#73241,
#73242,#73243,#73244,#73245,#73246,#73247),.UNSPECIFIED.,.F.,.F.,(4,3,3,
3,3,3,3,4),(352.987769606187,353.702737013943,354.701897287993,355.701057562044,
356.700217836095,357.699378110145,358.698538384196,359.270954913367),
 .UNSPECIFIED.);
#3028=B_SPLINE_CURVE_WITH_KNOTS('',3,(#73252,#73253,#73254,#73255,#73256,
#73257,#73258,#73259,#73260,#73261,#73262,#73263,#73264,#73265,#73266,#73267,
#73268,#73269,#73270,#73271,#73272,#73273),.UNSPECIFIED.,.F.,.F.,(4,3,3,
3,3,3,3,4),(-368.51798053644,-367.690980850652,-366.691820576602,-365.692660302551,
-364.6935000285,-363.694339754449,-362.695179480399,-362.23479522926),
 .UNSPECIFIED.);
#3029=B_SPLINE_CURVE_WITH_KNOTS('',3,(#73274,#73275,#73276,#73277,#73278,
#73279,#73280,#73281,#73282,#73283,#73284,#73285,#73286,#73287,#73288,#73289,
#73290,#73291,#73292,#73293,#73294,#73295),.UNSPECIFIED.,.F.,.F.,(4,3,3,
3,3,3,3,4),(359.270954913367,359.697698658247,360.696858932297,361.696019206348,
362.695179480399,363.69433975445,364.6935000285,365.554140220546),
 .UNSPECIFIED.);
#3030=B_SPLINE_CURVE_WITH_KNOTS('',3,(#73300,#73301,#73302,#73303,#73304,
#73305,#73306,#73307,#73308,#73309,#73310,#73311,#73312,#73313,#73314,#73315,
#73316,#73317,#73318,#73319,#73320,#73321,#73322,#73323,#73324),
 .UNSPECIFIED.,.F.,.F.,(4,3,3,3,3,3,3,3,4),(-374.80116584362,-374.685102769007,
-373.685942494956,-372.686782220906,-371.687621946855,-370.688461672804,
-369.689301398754,-368.690141124703,-368.51798053644),.UNSPECIFIED.);
#3031=B_SPLINE_CURVE_WITH_KNOTS('',3,(#73325,#73326,#73327,#73328,#73329,
#73330,#73331,#73332,#73333,#73334,#73335,#73336,#73337,#73338,#73339,#73340,
#73341,#73342,#73343,#73344,#73345,#73346,#73347,#73348,#73349),
 .UNSPECIFIED.,.F.,.F.,(4,3,3,3,3,3,3,3,4),(365.554140220546,365.692660302551,
366.691820576602,367.690980850652,368.690141124703,369.689301398754,370.688461672804,
371.687621946855,371.837325527726),.UNSPECIFIED.);
#3032=B_SPLINE_CURVE_WITH_KNOTS('',3,(#73354,#73355,#73356,#73357,#73358,
#73359,#73360,#73361,#73362,#73363,#73364,#73365,#73366,#73367,#73368,#73369,
#73370,#73371,#73372,#73373,#73374,#73375),.UNSPECIFIED.,.F.,.F.,(4,3,3,
3,3,3,3,4),(-381.084351150799,-380.680064413311,-379.68090413926,-378.68174386521,
-377.682583591159,-376.683423317108,-375.684263043058,-374.80116584362),
 .UNSPECIFIED.);
#3033=B_SPLINE_CURVE_WITH_KNOTS('',3,(#73376,#73377,#73378,#73379,#73380,
#73381,#73382,#73383,#73384,#73385,#73386,#73387,#73388,#73389,#73390,#73391,
#73392,#73393,#73394,#73395,#73396,#73397),.UNSPECIFIED.,.F.,.F.,(4,3,3,
3,3,3,3,4),(371.837325527726,372.686782220906,373.685942494956,374.685102769007,
375.684263043058,376.683423317108,377.682583591159,378.120510834905),
 .UNSPECIFIED.);
#3034=B_SPLINE_CURVE_WITH_KNOTS('',3,(#73402,#73403,#73404,#73405,#73406,
#73407,#73408,#73409,#73410,#73411,#73412,#73413,#73414,#73415,#73416,#73417,
#73418,#73419,#73420,#73421,#73422,#73423),.UNSPECIFIED.,.F.,.F.,(4,3,3,
3,3,3,3,4),(-387.367536457979,-386.675026057615,-385.675865783564,-384.676705509514,
-383.677545235463,-382.678384961412,-381.679224687362,-381.084351150799),
 .UNSPECIFIED.);
#3035=B_SPLINE_CURVE_WITH_KNOTS('',3,(#73424,#73425,#73426,#73427,#73428,
#73429,#73430,#73431,#73432,#73433,#73434,#73435,#73436,#73437,#73438,#73439,
#73440,#73441,#73442,#73443,#73444,#73445),.UNSPECIFIED.,.F.,.F.,(4,3,3,
3,3,3,3,4),(378.120510834905,378.68174386521,379.68090413926,380.680064413311,
381.679224687362,382.678384961412,383.677545235463,384.403696142085),
 .UNSPECIFIED.);
#3036=B_SPLINE_CURVE_WITH_KNOTS('',3,(#73450,#73451,#73452,#73453,#73454,
#73455,#73456,#73457,#73458,#73459,#73460,#73461,#73462,#73463,#73464,#73465,
#73466,#73467,#73468,#73469,#73470,#73471),.UNSPECIFIED.,.F.,.F.,(4,3,3,
3,3,3,3,4),(-393.650721765158,-392.669987701919,-391.670827427869,-390.671667153818,
-389.672506879767,-388.673346605717,-387.674186331666,-387.367536457979),
 .UNSPECIFIED.);
#3037=B_SPLINE_CURVE_WITH_KNOTS('',3,(#73472,#73473,#73474,#73475,#73476,
#73477,#73478,#73479,#73480,#73481,#73482,#73483,#73484,#73485,#73486,#73487,
#73488,#73489,#73490,#73491,#73492,#73493,#73494,#73495,#73496),
 .UNSPECIFIED.,.F.,.F.,(4,3,3,3,3,3,3,3,4),(384.403696142085,384.676705509514,
385.675865783564,386.675026057615,387.674186331666,388.673346605717,389.672506879767,
390.671667153818,390.686881449265),.UNSPECIFIED.);
#3038=B_SPLINE_CURVE_WITH_KNOTS('',3,(#73501,#73502,#73503,#73504,#73505,
#73506,#73507,#73508,#73509,#73510,#73511,#73512,#73513,#73514,#73515,#73516,
#73517,#73518,#73519,#73520,#73521,#73522,#73523,#73524,#73525),
 .UNSPECIFIED.,.F.,.F.,(4,3,3,3,3,3,3,3,4),(-399.933907072338,-399.664109620274,
-398.664949346223,-397.665789072173,-396.666628798122,-395.667468524071,
-394.668308250021,-393.66914797597,-393.650721765158),.UNSPECIFIED.);
#3039=B_SPLINE_CURVE_WITH_KNOTS('',3,(#73526,#73527,#73528,#73529,#73530,
#73531,#73532,#73533,#73534,#73535,#73536,#73537,#73538,#73539,#73540,#73541,
#73542,#73543,#73544,#73545,#73546,#73547),.UNSPECIFIED.,.F.,.F.,(4,3,3,
3,3,3,3,4),(390.686881449265,391.670827427869,392.669987701919,393.66914797597,
394.668308250021,395.667468524071,396.666628798122,396.970066756444),
 .UNSPECIFIED.);
#3040=B_SPLINE_CURVE_WITH_KNOTS('',3,(#73552,#73553,#73554,#73555,#73556,
#73557,#73558,#73559,#73560,#73561,#73562,#73563,#73564,#73565,#73566,#73567,
#73568,#73569,#73570,#73571,#73572,#73573),.UNSPECIFIED.,.F.,.F.,(4,3,3,
3,3,3,3,4),(-406.217092379517,-405.659071264578,-404.659910990528,-403.660750716477,
-402.661590442426,-401.662430168375,-400.663269894325,-399.933907072338),
 .UNSPECIFIED.);
#3041=B_SPLINE_CURVE_WITH_KNOTS('',3,(#73574,#73575,#73576,#73577,#73578,
#73579,#73580,#73581,#73582,#73583,#73584,#73585,#73586,#73587,#73588,#73589,
#73590,#73591,#73592,#73593,#73594,#73595),.UNSPECIFIED.,.F.,.F.,(4,3,3,
3,3,3,3,4),(396.970066756444,397.665789072173,398.664949346223,399.664109620274,
400.663269894325,401.662430168376,402.661590442426,403.253252063624),
 .UNSPECIFIED.);
#3042=B_SPLINE_CURVE_WITH_KNOTS('',3,(#73600,#73601,#73602,#73603,#73604,
#73605,#73606,#73607,#73608,#73609,#73610,#73611,#73612,#73613,#73614,#73615,
#73616,#73617,#73618,#73619,#73620,#73621),.UNSPECIFIED.,.F.,.F.,(4,3,3,
3,3,3,3,4),(-412.500277686697,-411.654032908882,-410.654872634832,-409.655712360781,
-408.65655208673,-407.65739181268,-406.658231538629,-406.217092379517),
 .UNSPECIFIED.);
#3043=B_SPLINE_CURVE_WITH_KNOTS('',3,(#73622,#73623,#73624,#73625,#73626,
#73627,#73628,#73629,#73630,#73631,#73632,#73633,#73634,#73635,#73636,#73637,
#73638,#73639,#73640,#73641,#73642,#73643),.UNSPECIFIED.,.F.,.F.,(4,3,3,
3,3,3,3,4),(403.253252063624,403.660750716477,404.659910990528,405.659071264578,
406.658231538629,407.65739181268,408.65655208673,409.536437370803),
 .UNSPECIFIED.);
#3044=B_SPLINE_CURVE_WITH_KNOTS('',3,(#73648,#73649,#73650,#73651,#73652,
#73653,#73654,#73655,#73656,#73657,#73658,#73659,#73660,#73661,#73662,#73663,
#73664,#73665,#73666,#73667,#73668,#73669,#73670,#73671,#73672),
 .UNSPECIFIED.,.F.,.F.,(4,3,3,3,3,3,3,3,4),(-418.783462993876,-418.648154827237,
-417.648994553186,-416.649834279136,-415.650674005085,-414.651513731034,
-413.652353456984,-412.653193182933,-412.500277686697),.UNSPECIFIED.);
#3045=B_SPLINE_CURVE_WITH_KNOTS('',3,(#73673,#73674,#73675,#73676,#73677,
#73678,#73679,#73680,#73681,#73682,#73683,#73684,#73685,#73686,#73687,#73688,
#73689,#73690,#73691,#73692,#73693,#73694,#73695,#73696,#73697),
 .UNSPECIFIED.,.F.,.F.,(4,3,3,3,3,3,3,3,4),(409.536437370803,409.655712360781,
410.654872634832,411.654032908882,412.653193182933,413.652353456984,414.651513731034,
415.650674005085,415.819622677983),.UNSPECIFIED.);
#3046=B_SPLINE_CURVE_WITH_KNOTS('',3,(#73702,#73703,#73704,#73705,#73706,
#73707,#73708,#73709,#73710,#73711,#73712,#73713,#73714,#73715,#73716,#73717,
#73718,#73719,#73720,#73721,#73722,#73723),.UNSPECIFIED.,.F.,.F.,(4,3,3,
3,3,3,3,4),(-425.066648301056,-424.643116471541,-423.643956197491,-422.64479592344,
-421.645635649389,-420.646475375338,-419.647315101288,-418.783462993876),
 .UNSPECIFIED.);
#3047=B_SPLINE_CURVE_WITH_KNOTS('',3,(#73724,#73725,#73726,#73727,#73728,
#73729,#73730,#73731,#73732,#73733,#73734,#73735,#73736,#73737,#73738,#73739,
#73740,#73741,#73742,#73743,#73744,#73745),.UNSPECIFIED.,.F.,.F.,(4,3,3,
3,3,3,3,4),(415.819622677983,416.649834279136,417.648994553187,418.648154827237,
419.647315101288,420.646475375339,421.645635649389,422.102807985162),
 .UNSPECIFIED.);
#3048=B_SPLINE_CURVE_WITH_KNOTS('',3,(#73750,#73751,#73752,#73753,#73754,
#73755,#73756,#73757,#73758,#73759,#73760,#73761,#73762,#73763,#73764,#73765,
#73766,#73767,#73768,#73769,#73770,#73771),.UNSPECIFIED.,.F.,.F.,(4,3,3,
3,3,3,3,4),(-431.349833608236,-430.638078115845,-429.638917841795,-428.639757567744,
-427.640597293693,-426.641437019643,-425.642276745592,-425.066648301056),
 .UNSPECIFIED.);
#3049=B_SPLINE_CURVE_WITH_KNOTS('',3,(#73772,#73773,#73774,#73775,#73776,
#73777,#73778,#73779,#73780,#73781,#73782,#73783,#73784,#73785,#73786,#73787,
#73788,#73789,#73790,#73791,#73792,#73793),.UNSPECIFIED.,.F.,.F.,(4,3,3,
3,3,3,3,4),(422.102807985162,422.64479592344,423.643956197491,424.643116471541,
425.642276745592,426.641437019643,427.640597293693,428.385993292342),
 .UNSPECIFIED.);
#3050=B_SPLINE_CURVE_WITH_KNOTS('',3,(#73798,#73799,#73800,#73801,#73802,
#73803,#73804,#73805,#73806,#73807,#73808,#73809,#73810,#73811,#73812,#73813,
#73814,#73815,#73816,#73817,#73818,#73819),.UNSPECIFIED.,.F.,.F.,(4,3,3,
3,3,3,3,4),(-437.633018915415,-436.633039760149,-435.633879486099,-434.634719212048,
-433.635558937997,-432.636398663947,-431.637238389896,-431.349833608236),
 .UNSPECIFIED.);
#3051=B_SPLINE_CURVE_WITH_KNOTS('',3,(#73820,#73821,#73822,#73823,#73824,
#73825,#73826,#73827,#73828,#73829,#73830,#73831,#73832,#73833,#73834,#73835,
#73836,#73837,#73838,#73839,#73840,#73841,#73842,#73843,#73844),
 .UNSPECIFIED.,.F.,.F.,(4,3,3,3,3,3,3,3,4),(428.385993292342,428.639757567744,
429.638917841795,430.638078115845,431.637238389896,432.636398663947,433.635558937997,
434.634719212048,434.669178599522),.UNSPECIFIED.);
#3052=B_SPLINE_CURVE_WITH_KNOTS('',3,(#73849,#73850,#73851,#73852,#73853,
#73854,#73855,#73856,#73857,#73858,#73859,#73860,#73861,#73862,#73863,#73864,
#73865,#73866,#73867,#73868,#73869,#73870),.UNSPECIFIED.,.F.,.F.,(4,3,3,
3,3,3,3,4),(-443.916204222595,-443.627161678504,-442.628001404454,-441.628841130403,
-440.629680856352,-439.630520582302,-438.631360308251,-437.633018915415),
 .UNSPECIFIED.);
#3053=B_SPLINE_CURVE_WITH_KNOTS('',3,(#73871,#73872,#73873,#73874,#73875,
#73876,#73877,#73878,#73879,#73880,#73881,#73882,#73883,#73884,#73885,#73886,
#73887,#73888,#73889,#73890,#73891,#73892),.UNSPECIFIED.,.F.,.F.,(4,3,3,
3,3,3,3,4),(434.669178599522,435.633879486099,436.633039760149,437.6322000342,
438.631360308251,439.630520582302,440.629680856352,440.952363906701),
 .UNSPECIFIED.);
#3054=B_SPLINE_CURVE_WITH_KNOTS('',3,(#73897,#73898,#73899,#73900,#73901,
#73902,#73903,#73904,#73905,#73906,#73907,#73908,#73909,#73910,#73911,#73912,
#73913,#73914,#73915,#73916,#73917,#73918),.UNSPECIFIED.,.F.,.F.,(4,3,3,
3,3,3,3,4),(-450.199389529774,-449.622123322808,-448.622963048758,-447.623802774707,
-446.624642500656,-445.625482226606,-444.626321952555,-443.916204222595),
 .UNSPECIFIED.);
#3055=B_SPLINE_CURVE_WITH_KNOTS('',3,(#73919,#73920,#73921,#73922,#73923,
#73924,#73925,#73926,#73927,#73928,#73929,#73930,#73931,#73932,#73933,#73934,
#73935,#73936,#73937,#73938,#73939,#73940),.UNSPECIFIED.,.F.,.F.,(4,3,3,
3,3,3,3,4),(440.952363906701,441.628841130403,442.628001404454,443.627161678504,
444.626321952555,445.625482226606,446.624642500656,447.235549213881),
 .UNSPECIFIED.);
#3056=B_SPLINE_CURVE_WITH_KNOTS('',3,(#73945,#73946,#73947,#73948,#73949,
#73950,#73951,#73952,#73953,#73954,#73955,#73956,#73957,#73958,#73959,#73960,
#73961,#73962,#73963,#73964,#73965,#73966),.UNSPECIFIED.,.F.,.F.,(4,3,3,
3,3,3,3,4),(-456.482574836954,-455.617084967113,-454.617924693062,-453.618764419011,
-452.61960414496,-451.62044387091,-450.621283596859,-450.199389529774),
 .UNSPECIFIED.);
#3057=B_SPLINE_CURVE_WITH_KNOTS('',3,(#73967,#73968,#73969,#73970,#73971,
#73972,#73973,#73974,#73975,#73976,#73977,#73978,#73979,#73980,#73981,#73982,
#73983,#73984,#73985,#73986,#73987,#73988),.UNSPECIFIED.,.F.,.F.,(4,3,3,
3,3,3,3,4),(447.235549213881,447.623802774707,448.622963048758,449.622123322808,
450.621283596859,451.62044387091,452.61960414496,453.51873452106),
 .UNSPECIFIED.);
#3058=B_SPLINE_CURVE_WITH_KNOTS('',3,(#73993,#73994,#73995,#73996,#73997,
#73998,#73999,#74000,#74001,#74002,#74003,#74004,#74005,#74006,#74007,#74008,
#74009,#74010,#74011,#74012,#74013,#74014,#74015,#74016,#74017),
 .UNSPECIFIED.,.F.,.F.,(4,3,3,3,3,3,3,3,4),(-462.765760144133,-462.611206885467,
-461.612046611417,-460.612886337366,-459.613726063315,-458.614565789265,
-457.615405515214,-456.616245241163,-456.482574836954),.UNSPECIFIED.);
#3059=B_SPLINE_CURVE_WITH_KNOTS('',3,(#74018,#74019,#74020,#74021,#74022,
#74023,#74024,#74025,#74026,#74027,#74028,#74029,#74030,#74031,#74032,#74033,
#74034,#74035,#74036,#74037,#74038,#74039,#74040,#74041,#74042),
 .UNSPECIFIED.,.F.,.F.,(4,3,3,3,3,3,3,3,4),(453.51873452106,453.618764419011,
454.617924693062,455.617084967112,456.616245241163,457.615405515214,458.614565789265,
459.613726063315,459.80191982824),.UNSPECIFIED.);
#3060=B_SPLINE_CURVE_WITH_KNOTS('',3,(#74047,#74048,#74049,#74050,#74051,
#74052,#74053,#74054,#74055,#74056,#74057,#74058,#74059,#74060,#74061,#74062,
#74063,#74064,#74065,#74066,#74067,#74068),.UNSPECIFIED.,.F.,.F.,(4,3,3,
3,3,3,3,4),(-469.048945451313,-468.606168529771,-467.607008255721,-466.60784798167,
-465.608687707619,-464.609527433569,-463.610367159518,-462.765760144133),
 .UNSPECIFIED.);
#3061=B_SPLINE_CURVE_WITH_KNOTS('',3,(#74069,#74070,#74071,#74072,#74073,
#74074,#74075,#74076,#74077,#74078,#74079,#74080,#74081,#74082,#74083,#74084,
#74085,#74086,#74087,#74088,#74089,#74090),.UNSPECIFIED.,.F.,.F.,(4,3,3,
3,3,3,3,4),(459.80191982824,460.612886337366,461.612046611417,462.611206885467,
463.610367159518,464.609527433569,465.608687707619,466.085105135419),
 .UNSPECIFIED.);
#3062=B_SPLINE_CURVE_WITH_KNOTS('',3,(#74096,#74097,#74098,#74099,#74100),
 .UNSPECIFIED.,.F.,.F.,(4,1,4),(480.663675999238,481.220059351747,482.136507703335),
 .UNSPECIFIED.);
#3063=B_SPLINE_CURVE_WITH_KNOTS('',3,(#74103,#74104,#74105,#74106),
 .UNSPECIFIED.,.F.,.F.,(4,4),(480.663675999238,480.898195182615),
 .UNSPECIFIED.);
#3064=B_SPLINE_CURVE_WITH_KNOTS('',3,(#74111,#74112,#74113,#74114,#74115,
#74116,#74117,#74118,#74119,#74120),.UNSPECIFIED.,.F.,.F.,(4,1,1,1,1,1,
1,4),(474.380490692059,475.225097707443,476.224257981494,477.223418255545,
478.222578529595,479.221738803646,480.220899077697,480.663675999238),
 .UNSPECIFIED.);
#3065=B_SPLINE_CURVE_WITH_KNOTS('',3,(#74121,#74122,#74123,#74124,#74125,
#74126,#74127,#74128,#74129,#74130,#74131),.UNSPECIFIED.,.F.,.F.,(4,1,1,
1,1,1,1,1,4),(474.380490692059,474.903233538311,475.902393812361,476.901554086412,
477.900714360463,478.899874634513,479.899034908564,480.398615045589,480.663675999238),
 .UNSPECIFIED.);
#3066=B_SPLINE_CURVE_WITH_KNOTS('',3,(#74136,#74137,#74138,#74139,#74140,
#74141,#74142,#74143,#74144,#74145,#74146),.UNSPECIFIED.,.F.,.F.,(4,1,1,
1,1,1,1,1,4),(468.097305384879,468.230975789088,469.230136063139,470.22929633719,
471.228456611241,472.227616885291,473.226777159342,474.225937433393,474.380490692059),
 .UNSPECIFIED.);
#3067=B_SPLINE_CURVE_WITH_KNOTS('',3,(#74147,#74148,#74149,#74150,#74151,
#74152,#74153,#74154,#74155,#74156),.UNSPECIFIED.,.F.,.F.,(4,1,1,1,1,1,
1,4),(468.097305384879,468.908271894006,469.907432168057,470.906592442108,
471.905752716158,472.904912990209,473.90407326426,474.380490692059),
 .UNSPECIFIED.);
#3068=B_SPLINE_CURVE_WITH_KNOTS('',3,(#74161,#74162,#74163,#74164,#74165,
#74166,#74167,#74168,#74169,#74170),.UNSPECIFIED.,.F.,.F.,(4,1,1,1,1,1,
1,4),(461.814120077699,462.236014144784,463.235174418835,464.234334692886,
465.233494966936,466.232655240987,467.231815515038,468.097305384879),
 .UNSPECIFIED.);
#3069=B_SPLINE_CURVE_WITH_KNOTS('',3,(#74171,#74172,#74173,#74174,#74175,
#74176,#74177,#74178,#74179,#74180,#74181),.UNSPECIFIED.,.F.,.F.,(4,1,1,
1,1,1,1,1,4),(461.8141200777,461.914149975652,462.913310249702,463.912470523753,
464.911630797804,465.910791071854,466.909951345905,467.909111619956,468.097305384879),
 .UNSPECIFIED.);
#3070=B_SPLINE_CURVE_WITH_KNOTS('',3,(#74186,#74187,#74188,#74189,#74190,
#74191,#74192,#74193,#74194,#74195),.UNSPECIFIED.,.F.,.F.,(4,1,1,1,1,1,
1,4),(455.53093477052,456.24105250048,457.240212774531,458.239373048582,
459.238533322632,460.237693596683,461.236853870734,461.814120077699),
 .UNSPECIFIED.);
#3071=B_SPLINE_CURVE_WITH_KNOTS('',3,(#74196,#74197,#74198,#74199,#74200,
#74201,#74202,#74203,#74204,#74205),.UNSPECIFIED.,.F.,.F.,(4,1,1,1,1,1,
1,4),(455.53093477052,455.919188331348,456.918348605398,457.917508879449,
458.9166691535,459.91582942755,460.914989701601,461.8141200777),
 .UNSPECIFIED.);
#3072=B_SPLINE_CURVE_WITH_KNOTS('',3,(#74210,#74211,#74212,#74213,#74214,
#74215,#74216,#74217,#74218,#74219),.UNSPECIFIED.,.F.,.F.,(4,1,1,1,1,1,
1,4),(449.24774946334,450.246090856176,451.245251130227,452.244411404278,
453.243571678328,454.242731952379,455.24189222643,455.53093477052),
 .UNSPECIFIED.);
#3073=B_SPLINE_CURVE_WITH_KNOTS('',3,(#74220,#74221,#74222,#74223,#74224,
#74225,#74226,#74227,#74228,#74229),.UNSPECIFIED.,.F.,.F.,(4,1,1,1,1,1,
1,4),(449.24774946334,449.924226687043,450.923386961094,451.922547235145,
452.921707509195,453.920867783246,454.920028057297,455.53093477052),
 .UNSPECIFIED.);
#3074=B_SPLINE_CURVE_WITH_KNOTS('',3,(#74234,#74235,#74236,#74237,#74238,
#74239,#74240,#74241,#74242,#74243,#74244),.UNSPECIFIED.,.F.,.F.,(4,1,1,
1,1,1,1,1,4),(442.964564156161,443.251968937821,444.251129211872,445.250289485923,
446.249449759973,447.248610034024,448.247770308075,449.246930582125,449.24774946334),
 .UNSPECIFIED.);
#3075=B_SPLINE_CURVE_WITH_KNOTS('',3,(#74245,#74246,#74247,#74248,#74249,
#74250,#74251,#74252,#74253,#74254),.UNSPECIFIED.,.F.,.F.,(4,1,1,1,1,1,
1,4),(442.964564156161,443.929265042739,444.92842531679,445.927585590841,
446.926745864891,447.925906138942,448.925066412993,449.24774946334),
 .UNSPECIFIED.);
#3076=B_SPLINE_CURVE_WITH_KNOTS('',3,(#74259,#74260,#74261,#74262,#74263,
#74264,#74265,#74266,#74267,#74268),.UNSPECIFIED.,.F.,.F.,(4,1,1,1,1,1,
1,4),(436.681378848981,437.257007293517,438.256167567568,439.255327841619,
440.254488115669,441.25364838972,442.252808663771,442.964564156161),
 .UNSPECIFIED.);
#3077=B_SPLINE_CURVE_WITH_KNOTS('',3,(#74269,#74270,#74271,#74272,#74273,
#74274,#74275,#74276,#74277,#74278,#74279),.UNSPECIFIED.,.F.,.F.,(4,1,1,
1,1,1,1,1,4),(436.681378848981,436.935143124384,437.934303398435,438.933463672486,
439.932623946537,440.931784220587,441.930944494638,442.930104768689,442.964564156161),
 .UNSPECIFIED.);
#3078=B_SPLINE_CURVE_WITH_KNOTS('',3,(#74284,#74285,#74286,#74287,#74288,
#74289,#74290,#74291,#74292,#74293),.UNSPECIFIED.,.F.,.F.,(4,1,1,1,1,1,
1,4),(430.398193541802,431.262045649213,432.261205923264,433.260366197314,
434.259526471365,435.258686745416,436.257847019467,436.681378848981),
 .UNSPECIFIED.);
#3079=B_SPLINE_CURVE_WITH_KNOTS('',3,(#74294,#74295,#74296,#74297,#74298,
#74299,#74300,#74301,#74302,#74303),.UNSPECIFIED.,.F.,.F.,(4,1,1,1,1,1,
1,4),(430.398193541802,430.94018148008,431.939341754131,432.938502028182,
433.937662302232,434.936822576283,435.935982850334,436.681378848981),
 .UNSPECIFIED.);
#3080=B_SPLINE_CURVE_WITH_KNOTS('',3,(#74308,#74309,#74310,#74311,#74312,
#74313,#74314,#74315,#74316,#74317,#74318),.UNSPECIFIED.,.F.,.F.,(4,1,1,
1,1,1,1,1,4),(424.115008234622,424.267923730858,425.267084004909,426.26624427896,
427.26540455301,428.264564827061,429.263725101112,430.262885375162,430.398193541802),
 .UNSPECIFIED.);
#3081=B_SPLINE_CURVE_WITH_KNOTS('',3,(#74319,#74320,#74321,#74322,#74323,
#74324,#74325,#74326,#74327,#74328),.UNSPECIFIED.,.F.,.F.,(4,1,1,1,1,1,
1,4),(424.115008234622,424.945219835776,425.944380109827,426.943540383878,
427.942700657928,428.941860931979,429.94102120603,430.398193541802),
 .UNSPECIFIED.);
#3082=B_SPLINE_CURVE_WITH_KNOTS('',3,(#74333,#74334,#74335,#74336,#74337,
#74338,#74339,#74340,#74341,#74342),.UNSPECIFIED.,.F.,.F.,(4,1,1,1,1,1,
1,4),(417.831822927443,418.272962086554,419.272122360605,420.271282634656,
421.270442908706,422.269603182757,423.268763456808,424.115008234622),
 .UNSPECIFIED.);
#3083=B_SPLINE_CURVE_WITH_KNOTS('',3,(#74343,#74344,#74345,#74346,#74347,
#74348,#74349,#74350,#74351,#74352,#74353),.UNSPECIFIED.,.F.,.F.,(4,1,1,
1,1,1,1,1,4),(417.831822927443,417.951097917421,418.950258191472,419.949418465523,
420.948578739574,421.947739013624,422.946899287675,423.946059561726,424.115008234622),
 .UNSPECIFIED.);
#3084=B_SPLINE_CURVE_WITH_KNOTS('',3,(#74358,#74359,#74360,#74361,#74362,
#74363,#74364,#74365,#74366,#74367),.UNSPECIFIED.,.F.,.F.,(4,1,1,1,1,1,
1,4),(411.548637620263,412.27800044225,413.277160716301,414.276320990351,
415.275481264402,416.274641538453,417.273801812504,417.831822927443),
 .UNSPECIFIED.);
#3085=B_SPLINE_CURVE_WITH_KNOTS('',3,(#74368,#74369,#74370,#74371,#74372,
#74373,#74374,#74375,#74376,#74377),.UNSPECIFIED.,.F.,.F.,(4,1,1,1,1,1,
1,4),(411.548637620263,411.956136273117,412.955296547168,413.954456821219,
414.953617095269,415.95277736932,416.951937643371,417.831822927443),
 .UNSPECIFIED.);
#3086=B_SPLINE_CURVE_WITH_KNOTS('',3,(#74382,#74383,#74384,#74385,#74386,
#74387,#74388,#74389,#74390,#74391,#74392),.UNSPECIFIED.,.F.,.F.,(4,1,1,
1,1,1,1,1,4),(405.265452313083,405.283878523895,406.283038797946,407.282199071997,
408.281359346047,409.280519620098,410.279679894149,411.278840168199,411.548637620263),
 .UNSPECIFIED.);
#3087=B_SPLINE_CURVE_WITH_KNOTS('',3,(#74393,#74394,#74395,#74396,#74397,
#74398,#74399,#74400,#74401,#74402),.UNSPECIFIED.,.F.,.F.,(4,1,1,1,1,1,
1,4),(405.265452313083,405.961174628813,406.960334902864,407.959495176915,
408.958655450965,409.957815725016,410.956975999067,411.548637620263),
 .UNSPECIFIED.);
#3088=B_SPLINE_CURVE_WITH_KNOTS('',3,(#74407,#74408,#74409,#74410,#74411,
#74412,#74413,#74414,#74415,#74416),.UNSPECIFIED.,.F.,.F.,(4,1,1,1,1,1,
1,4),(398.982267005904,399.288916879591,400.288077153642,401.287237427693,
402.286397701743,403.285557975794,404.284718249845,405.265452313083),
 .UNSPECIFIED.);
#3089=B_SPLINE_CURVE_WITH_KNOTS('',3,(#74417,#74418,#74419,#74420,#74421,
#74422,#74423,#74424,#74425,#74426),.UNSPECIFIED.,.F.,.F.,(4,1,1,1,1,1,
1,4),(398.982267005904,399.966212984509,400.96537325856,401.964533532611,
402.963693806661,403.962854080712,404.962014354763,405.265452313083),
 .UNSPECIFIED.);
#3090=B_SPLINE_CURVE_WITH_KNOTS('',3,(#74431,#74432,#74433,#74434,#74435,
#74436,#74437,#74438,#74439,#74440),.UNSPECIFIED.,.F.,.F.,(4,1,1,1,1,1,
1,4),(392.699081698724,393.293955235287,394.293115509338,395.292275783388,
396.291436057439,397.29059633149,398.289756605541,398.982267005904),
 .UNSPECIFIED.);
#3091=B_SPLINE_CURVE_WITH_KNOTS('',3,(#74441,#74442,#74443,#74444,#74445,
#74446,#74447,#74448,#74449,#74450,#74451),.UNSPECIFIED.,.F.,.F.,(4,1,1,
1,1,1,1,1,4),(392.699081698724,392.972091066154,393.971251340205,394.970411614256,
395.969571888306,396.968732162357,397.967892436408,398.967052710458,398.982267005904),
 .UNSPECIFIED.);
#3092=B_SPLINE_CURVE_WITH_KNOTS('',3,(#74456,#74457,#74458,#74459,#74460,
#74461,#74462,#74463,#74464,#74465),.UNSPECIFIED.,.F.,.F.,(4,1,1,1,1,1,
1,4),(386.415896391545,387.298993590983,388.298153865034,389.297314139084,
390.296474413135,391.295634687186,392.294794961236,392.699081698724),
 .UNSPECIFIED.);
#3093=B_SPLINE_CURVE_WITH_KNOTS('',3,(#74466,#74467,#74468,#74469,#74470,
#74471,#74472,#74473,#74474,#74475),.UNSPECIFIED.,.F.,.F.,(4,1,1,1,1,1,
1,4),(386.415896391545,386.97712942185,387.976289695901,388.975449969952,
389.974610244002,390.973770518053,391.972930792104,392.699081698724),
 .UNSPECIFIED.);
#3094=B_SPLINE_CURVE_WITH_KNOTS('',3,(#74480,#74481,#74482,#74483,#74484,
#74485,#74486,#74487,#74488,#74489,#74490),.UNSPECIFIED.,.F.,.F.,(4,1,1,
1,1,1,1,1,4),(380.132711084365,380.304871672628,381.304031946679,382.303192220729,
383.30235249478,384.301512768831,385.300673042882,386.299833316932,386.415896391545),
 .UNSPECIFIED.);
#3095=B_SPLINE_CURVE_WITH_KNOTS('',3,(#74491,#74492,#74493,#74494,#74495,
#74496,#74497,#74498,#74499,#74500),.UNSPECIFIED.,.F.,.F.,(4,1,1,1,1,1,
1,4),(380.132711084365,380.982167777546,381.981328051597,382.980488325648,
383.979648599698,384.978808873749,385.9779691478,386.415896391545),
 .UNSPECIFIED.);
#3096=B_SPLINE_CURVE_WITH_KNOTS('',3,(#74505,#74506,#74507,#74508,#74509,
#74510,#74511,#74512,#74513,#74514),.UNSPECIFIED.,.F.,.F.,(4,1,1,1,1,1,
1,4),(373.849525777186,374.309910028324,375.309070302375,376.308230576425,
377.307390850476,378.306551124527,379.305711398577,380.132711084365),
 .UNSPECIFIED.);
#3097=B_SPLINE_CURVE_WITH_KNOTS('',3,(#74515,#74516,#74517,#74518,#74519,
#74520,#74521,#74522,#74523,#74524,#74525),.UNSPECIFIED.,.F.,.F.,(4,1,1,
1,1,1,1,1,4),(373.849525777186,373.988045859191,374.987206133242,375.986366407293,
376.985526681343,377.984686955394,378.983847229445,379.983007503495,380.132711084365),
 .UNSPECIFIED.);
#3098=B_SPLINE_CURVE_WITH_KNOTS('',3,(#74530,#74531,#74532,#74533,#74534,
#74535,#74536,#74537,#74538,#74539),.UNSPECIFIED.,.F.,.F.,(4,1,1,1,1,1,
1,4),(367.566340470006,368.31494838402,369.314108658071,370.313268932121,
371.312429206172,372.311589480223,373.310749754273,373.849525777186),
 .UNSPECIFIED.);
#3099=B_SPLINE_CURVE_WITH_KNOTS('',3,(#74540,#74541,#74542,#74543,#74544,
#74545,#74546,#74547,#74548,#74549),.UNSPECIFIED.,.F.,.F.,(4,1,1,1,1,1,
1,4),(367.566340470006,367.993084214887,368.992244488938,369.991404762989,
370.990565037039,371.98972531109,372.988885585141,373.849525777186),
 .UNSPECIFIED.);
#3100=B_SPLINE_CURVE_WITH_KNOTS('',3,(#74554,#74555,#74556,#74557,#74558,
#74559,#74560,#74561,#74562,#74563,#74564),.UNSPECIFIED.,.F.,.F.,(4,1,1,
1,1,1,1,1,4),(361.283155162826,361.320826465665,362.319986739716,363.319147013766,
364.318307287817,365.317467561868,366.316627835919,367.315788109969,367.566340470006),
 .UNSPECIFIED.);
#3101=B_SPLINE_CURVE_WITH_KNOTS('',3,(#74565,#74566,#74567,#74568,#74569,
#74570,#74571,#74572,#74573,#74574),.UNSPECIFIED.,.F.,.F.,(4,1,1,1,1,1,
1,4),(361.283155162827,361.998122570583,362.997282844634,363.996443118684,
364.995603392735,365.994763666786,366.993923940837,367.566340470006),
 .UNSPECIFIED.);
#3102=B_SPLINE_CURVE_WITH_KNOTS('',3,(#74579,#74580,#74581,#74582,#74583,
#74584,#74585,#74586,#74587,#74588),.UNSPECIFIED.,.F.,.F.,(4,1,1,1,1,1,
1,4),(354.999969855647,355.325864821361,356.325025095412,357.324185369462,
358.323345643513,359.322505917564,360.321666191614,361.283155162826),
 .UNSPECIFIED.);
#3103=B_SPLINE_CURVE_WITH_KNOTS('',3,(#74589,#74590,#74591,#74592,#74593,
#74594,#74595,#74596,#74597,#74598,#74599),.UNSPECIFIED.,.F.,.F.,(4,1,1,
1,1,1,1,1,4),(354.999969855647,355.004000652228,356.003160926279,357.00232120033,
358.00148147438,359.000641748431,359.999802022482,360.998962296532,361.283155162827),
 .UNSPECIFIED.);
#3104=B_SPLINE_CURVE_WITH_KNOTS('',3,(#74604,#74605,#74606,#74607,#74608,
#74609,#74610,#74611,#74612,#74613),.UNSPECIFIED.,.F.,.F.,(4,1,1,1,1,1,
1,4),(348.716784548467,349.330903177057,350.330063451108,351.329223725158,
352.328383999209,353.32754427326,354.32670454731,354.999969855647),
 .UNSPECIFIED.);
#3105=B_SPLINE_CURVE_WITH_KNOTS('',3,(#74614,#74615,#74616,#74617,#74618,
#74619,#74620,#74621,#74622,#74623),.UNSPECIFIED.,.F.,.F.,(4,1,1,1,1,1,
1,4),(348.716784548468,349.009039007924,350.008199281975,351.007359556026,
352.006519830076,353.005680104127,354.004840378178,354.999969855647),
 .UNSPECIFIED.);
#3106=B_SPLINE_CURVE_WITH_KNOTS('',3,(#74628,#74629,#74630,#74631,#74632,
#74633,#74634,#74635,#74636,#74637),.UNSPECIFIED.,.F.,.F.,(4,1,1,1,1,1,
1,4),(342.433599241288,343.335941532753,344.335101806803,345.334262080854,
346.333422354905,347.332582628956,348.331742903006,348.716784548467),
 .UNSPECIFIED.);
#3107=B_SPLINE_CURVE_WITH_KNOTS('',3,(#74638,#74639,#74640,#74641,#74642,
#74643,#74644,#74645,#74646,#74647),.UNSPECIFIED.,.F.,.F.,(4,1,1,1,1,1,
1,4),(342.433599241288,343.01407736362,344.013237637671,345.012397911721,
346.011558185772,347.010718459823,348.009878733874,348.716784548468),
 .UNSPECIFIED.);
#3108=B_SPLINE_CURVE_WITH_KNOTS('',3,(#74652,#74653,#74654,#74655,#74656,
#74657,#74658,#74659,#74660,#74661,#74662),.UNSPECIFIED.,.F.,.F.,(4,1,1,
1,1,1,1,1,4),(336.150413934108,336.341819614398,337.340979888449,338.340140162499,
339.33930043655,340.338460710601,341.337620984651,342.336781258702,342.433599241288),
 .UNSPECIFIED.);
#3109=B_SPLINE_CURVE_WITH_KNOTS('',3,(#74663,#74664,#74665,#74666,#74667,
#74668,#74669,#74670,#74671,#74672),.UNSPECIFIED.,.F.,.F.,(4,1,1,1,1,1,
1,4),(336.150413934108,337.019115719316,338.018275993367,339.017436267417,
340.016596541468,341.015756815519,342.014917089569,342.433599241288),
 .UNSPECIFIED.);
#3110=B_SPLINE_CURVE_WITH_KNOTS('',3,(#74677,#74678,#74679,#74680,#74681,
#74682,#74683,#74684,#74685,#74686),.UNSPECIFIED.,.F.,.F.,(4,1,1,1,1,1,
1,4),(329.867228626929,330.346857970094,331.346018244145,332.345178518195,
333.344338792246,334.343499066297,335.342659340347,336.150413934108),
 .UNSPECIFIED.);
#3111=B_SPLINE_CURVE_WITH_KNOTS('',3,(#74687,#74688,#74689,#74690,#74691,
#74692,#74693,#74694,#74695,#74696,#74697),.UNSPECIFIED.,.F.,.F.,(4,1,1,
1,1,1,1,1,4),(329.867228626929,330.024993800961,331.024154075012,332.023314349063,
333.022474623113,334.021634897164,335.020795171215,336.019955445265,336.150413934108),
 .UNSPECIFIED.);
#3112=B_SPLINE_CURVE_WITH_KNOTS('',3,(#74702,#74703,#74704,#74705,#74706,
#74707,#74708,#74709,#74710,#74711),.UNSPECIFIED.,.F.,.F.,(4,1,1,1,1,1,
1,4),(323.584043319749,324.35189632579,325.35105659984,326.350216873891,
327.349377147942,328.348537421993,329.347697696043,329.867228626929),
 .UNSPECIFIED.);
#3113=B_SPLINE_CURVE_WITH_KNOTS('',3,(#74712,#74713,#74714,#74715,#74716,
#74717,#74718,#74719,#74720,#74721),.UNSPECIFIED.,.F.,.F.,(4,1,1,1,1,1,
1,4),(323.584043319749,324.030032156657,325.029192430708,326.028352704758,
327.027512978809,328.02667325286,329.025833526911,329.867228626929),
 .UNSPECIFIED.);
#3114=B_SPLINE_CURVE_WITH_KNOTS('',3,(#74726,#74727,#74728,#74729,#74730,
#74731,#74732,#74733,#74734,#74735,#74736),.UNSPECIFIED.,.F.,.F.,(4,1,1,
1,1,1,1,1,4),(317.30085801257,317.357774407435,318.356934681486,319.356094955536,
320.355255229587,321.354415503638,322.353575777688,323.352736051739,323.584043319749),
 .UNSPECIFIED.);
#3115=B_SPLINE_CURVE_WITH_KNOTS('',3,(#74737,#74738,#74739,#74740,#74741,
#74742,#74743,#74744,#74745,#74746),.UNSPECIFIED.,.F.,.F.,(4,1,1,1,1,1,
1,4),(317.30085801257,318.035070512353,319.034230786404,320.033391060454,
321.032551334505,322.031711608556,323.030871882606,323.584043319749),
 .UNSPECIFIED.);
#3116=B_SPLINE_CURVE_WITH_KNOTS('',3,(#74751,#74752,#74753,#74754,#74755,
#74756,#74757,#74758,#74759,#74760),.UNSPECIFIED.,.F.,.F.,(4,1,1,1,1,1,
1,4),(311.01767270539,311.362812763131,312.361973037182,313.361133311232,
314.360293585283,315.359453859334,316.358614133384,317.30085801257),
 .UNSPECIFIED.);
#3117=B_SPLINE_CURVE_WITH_KNOTS('',3,(#74761,#74762,#74763,#74764,#74765,
#74766,#74767,#74768,#74769,#74770,#74771),.UNSPECIFIED.,.F.,.F.,(4,1,1,
1,1,1,1,1,4),(311.01767270539,311.040948593998,312.040108868049,313.039269142099,
314.03842941615,315.037589690201,316.036749964252,317.035910238302,317.30085801257),
 .UNSPECIFIED.);
#3118=B_SPLINE_CURVE_WITH_KNOTS('',3,(#74776,#74777,#74778,#74779,#74780,
#74781,#74782,#74783,#74784,#74785),.UNSPECIFIED.,.F.,.F.,(4,1,1,1,1,1,
1,4),(304.73448739821,305.367851118827,306.367011392877,307.366171666928,
308.365331940979,309.364492215029,310.36365248908,311.01767270539),
 .UNSPECIFIED.);
#3119=B_SPLINE_CURVE_WITH_KNOTS('',3,(#74786,#74787,#74788,#74789,#74790,
#74791,#74792,#74793,#74794,#74795),.UNSPECIFIED.,.F.,.F.,(4,1,1,1,1,1,
1,4),(304.73448739821,305.045986949694,306.045147223745,307.044307497795,
308.043467771846,309.042628045897,310.041788319947,311.01767270539),
 .UNSPECIFIED.);
#3120=B_SPLINE_CURVE_WITH_KNOTS('',3,(#74800,#74801,#74802,#74803,#74804,
#74805,#74806,#74807,#74808,#74809),.UNSPECIFIED.,.F.,.F.,(4,1,1,1,1,1,
1,4),(298.451302091031,299.372889474523,300.372049748573,301.371210022624,
302.370370296675,303.369530570725,304.368690844776,304.73448739821),
 .UNSPECIFIED.);
#3121=B_SPLINE_CURVE_WITH_KNOTS('',3,(#74810,#74811,#74812,#74813,#74814,
#74815,#74816,#74817,#74818,#74819),.UNSPECIFIED.,.F.,.F.,(4,1,1,1,1,1,
1,4),(298.451302091031,299.05102530539,300.050185579441,301.049345853491,
302.048506127542,303.047666401593,304.046826675643,304.73448739821),
 .UNSPECIFIED.);
#3122=B_SPLINE_CURVE_WITH_KNOTS('',3,(#74824,#74825,#74826,#74827,#74828,
#74829,#74830,#74831,#74832,#74833,#74834),.UNSPECIFIED.,.F.,.F.,(4,1,1,
1,1,1,1,1,4),(292.168116783851,292.378767556168,293.377927830219,294.377088104269,
295.37624837832,296.375408652371,297.374568926421,298.373729200472,298.451302091031),
 .UNSPECIFIED.);
#3123=B_SPLINE_CURVE_WITH_KNOTS('',3,(#74835,#74836,#74837,#74838,#74839,
#74840,#74841,#74842,#74843,#74844),.UNSPECIFIED.,.F.,.F.,(4,1,1,1,1,1,
1,4),(292.168116783851,293.056063661086,294.055223935136,295.054384209187,
296.053544483238,297.052704757289,298.051865031339,298.451302091031),
 .UNSPECIFIED.);
#3124=B_SPLINE_CURVE_WITH_KNOTS('',3,(#74849,#74850,#74851,#74852,#74853,
#74854,#74855,#74856,#74857,#74858),.UNSPECIFIED.,.F.,.F.,(4,1,1,1,1,1,
1,4),(285.884931476672,286.383805911864,287.382966185914,288.382126459965,
289.381286734016,290.380447008066,291.379607282117,292.168116783851),
 .UNSPECIFIED.);
#3125=B_SPLINE_CURVE_WITH_KNOTS('',3,(#74859,#74860,#74861,#74862,#74863,
#74864,#74865,#74866,#74867,#74868,#74869),.UNSPECIFIED.,.F.,.F.,(4,1,1,
1,1,1,1,1,4),(285.884931476672,286.061941742731,287.061102016782,288.060262290832,
289.059422564883,290.058582838934,291.057743112984,292.056903387035,292.168116783851),
 .UNSPECIFIED.);
#3126=B_SPLINE_CURVE_WITH_KNOTS('',3,(#74874,#74875,#74876,#74877,#74878,
#74879,#74880,#74881,#74882,#74883),.UNSPECIFIED.,.F.,.F.,(4,1,1,1,1,1,
1,4),(279.601746169492,280.38884426756,281.38800454161,282.387164815661,
283.386325089712,284.385485363762,285.384645637813,285.884931476672),
 .UNSPECIFIED.);
#3127=B_SPLINE_CURVE_WITH_KNOTS('',3,(#74884,#74885,#74886,#74887,#74888,
#74889,#74890,#74891,#74892,#74893),.UNSPECIFIED.,.F.,.F.,(4,1,1,1,1,1,
1,4),(279.601746169492,280.066980098427,281.066140372478,282.065300646528,
283.064460920579,284.06362119463,285.06278146868,285.884931476672),
 .UNSPECIFIED.);
#3128=B_SPLINE_CURVE_WITH_KNOTS('',3,(#74898,#74899,#74900,#74901,#74902,
#74903,#74904,#74905,#74906,#74907,#74908),.UNSPECIFIED.,.F.,.F.,(4,1,1,
1,1,1,1,1,4),(273.318560862313,273.394722349205,274.393882623256,275.393042897306,
276.392203171357,277.391363445408,278.390523719458,279.389683993509,279.601746169492),
 .UNSPECIFIED.);
#3129=B_SPLINE_CURVE_WITH_KNOTS('',3,(#74909,#74910,#74911,#74912,#74913,
#74914,#74915,#74916,#74917,#74918),.UNSPECIFIED.,.F.,.F.,(4,1,1,1,1,1,
1,4),(273.318560862313,274.072018454123,275.071178728173,276.070339002224,
277.069499276275,278.068659550326,279.067819824376,279.601746169492),
 .UNSPECIFIED.);
#3130=B_SPLINE_CURVE_WITH_KNOTS('',3,(#74923,#74924,#74925,#74926,#74927,
#74928,#74929,#74930,#74931,#74932),.UNSPECIFIED.,.F.,.F.,(4,1,1,1,1,1,
1,4),(267.035375555133,267.399760704901,268.398920978951,269.398081253002,
270.397241527053,271.396401801103,272.395562075154,273.318560862313),
 .UNSPECIFIED.);
#3131=B_SPLINE_CURVE_WITH_KNOTS('',3,(#74933,#74934,#74935,#74936,#74937,
#74938,#74939,#74940,#74941,#74942,#74943),.UNSPECIFIED.,.F.,.F.,(4,1,1,
1,1,1,1,1,4),(267.035375555133,267.077896535768,268.077056809819,269.076217083869,
270.07537735792,271.074537631971,272.073697906021,273.072858180072,273.318560862313),
 .UNSPECIFIED.);
#3132=B_SPLINE_CURVE_WITH_KNOTS('',3,(#74948,#74949,#74950,#74951,#74952,
#74953,#74954,#74955,#74956,#74957),.UNSPECIFIED.,.F.,.F.,(4,1,1,1,1,1,
1,4),(260.752190247953,261.404799060597,262.403959334647,263.403119608698,
264.402279882749,265.401440156799,266.40060043085,267.035375555133),
 .UNSPECIFIED.);
#3133=B_SPLINE_CURVE_WITH_KNOTS('',3,(#74958,#74959,#74960,#74961,#74962,
#74963,#74964,#74965,#74966,#74967),.UNSPECIFIED.,.F.,.F.,(4,1,1,1,1,1,
1,4),(260.752190247954,261.082934891464,262.082095165515,263.081255439565,
264.080415713616,265.079575987667,266.078736261717,267.035375555133),
 .UNSPECIFIED.);
#3134=B_SPLINE_CURVE_WITH_KNOTS('',3,(#74972,#74973,#74974,#74975,#74976,
#74977,#74978,#74979,#74980,#74981),.UNSPECIFIED.,.F.,.F.,(4,1,1,1,1,1,
1,4),(254.469004940774,255.409837416293,256.408997690343,257.408157964394,
258.407318238445,259.406478512495,260.405638786546,260.752190247953),
 .UNSPECIFIED.);
#3135=B_SPLINE_CURVE_WITH_KNOTS('',3,(#74982,#74983,#74984,#74985,#74986,
#74987,#74988,#74989,#74990,#74991),.UNSPECIFIED.,.F.,.F.,(4,1,1,1,1,1,
1,4),(254.469004940774,255.08797324716,256.08713352121,257.086293795261,
258.085454069312,259.084614343362,260.083774617413,260.752190247954),
 .UNSPECIFIED.);
#3136=B_SPLINE_CURVE_WITH_KNOTS('',3,(#74996,#74997,#74998,#74999,#75000,
#75001,#75002,#75003,#75004,#75005,#75006),.UNSPECIFIED.,.F.,.F.,(4,1,1,
1,1,1,1,1,4),(248.185819633594,248.415715497938,249.414875771988,250.414036046039,
251.41319632009,252.41235659414,253.411516868191,254.410677142242,254.469004940774),
 .UNSPECIFIED.);
#3137=B_SPLINE_CURVE_WITH_KNOTS('',3,(#75007,#75008,#75009,#75010,#75011,
#75012,#75013,#75014,#75015,#75016),.UNSPECIFIED.,.F.,.F.,(4,1,1,1,1,1,
1,4),(248.185819633594,249.093011602856,250.092171876906,251.091332150957,
252.090492425008,253.089652699058,254.088812973109,254.469004940774),
 .UNSPECIFIED.);
#3138=B_SPLINE_CURVE_WITH_KNOTS('',3,(#75021,#75022,#75023,#75024,#75025,
#75026,#75027,#75028,#75029,#75030),.UNSPECIFIED.,.F.,.F.,(4,1,1,1,1,1,
1,4),(241.902634326415,242.420753853634,243.419914127684,244.419074401735,
245.418234675786,246.417394949836,247.416555223887,248.185819633594),
 .UNSPECIFIED.);
#3139=B_SPLINE_CURVE_WITH_KNOTS('',3,(#75031,#75032,#75033,#75034,#75035,
#75036,#75037,#75038,#75039,#75040,#75041),.UNSPECIFIED.,.F.,.F.,(4,1,1,
1,1,1,1,1,4),(241.902634326415,242.098889684501,243.098049958552,244.097210232602,
245.096370506653,246.095530780704,247.094691054754,248.093851328805,248.185819633594),
 .UNSPECIFIED.);
#3140=B_SPLINE_CURVE_WITH_KNOTS('',3,(#75046,#75047,#75048,#75049,#75050,
#75051,#75052,#75053,#75054,#75055),.UNSPECIFIED.,.F.,.F.,(4,1,1,1,1,1,
1,4),(235.619449019235,236.42579220933,237.42495248338,238.424112757431,
239.423273031482,240.422433305532,241.421593579583,241.902634326415),
 .UNSPECIFIED.);
#3141=B_SPLINE_CURVE_WITH_KNOTS('',3,(#75056,#75057,#75058,#75059,#75060,
#75061,#75062,#75063,#75064,#75065),.UNSPECIFIED.,.F.,.F.,(4,1,1,1,1,1,
1,4),(235.619449019235,236.103928040197,237.103088314247,238.102248588298,
239.101408862349,240.100569136399,241.09972941045,241.902634326415),
 .UNSPECIFIED.);
#3142=B_SPLINE_CURVE_WITH_KNOTS('',3,(#75070,#75071,#75072,#75073,#75074,
#75075,#75076,#75077,#75078,#75079,#75080),.UNSPECIFIED.,.F.,.F.,(4,1,1,
1,1,1,1,1,4),(229.336263712056,229.431670290975,230.430830565025,231.429990839076,
232.429151113127,233.428311387177,234.427471661228,235.426631935279,235.619449019235),
 .UNSPECIFIED.);
#3143=B_SPLINE_CURVE_WITH_KNOTS('',3,(#75081,#75082,#75083,#75084,#75085,
#75086,#75087,#75088,#75089,#75090),.UNSPECIFIED.,.F.,.F.,(4,1,1,1,1,1,
1,4),(229.336263712056,230.108966395893,231.108126669943,232.107286943994,
233.106447218045,234.105607492095,235.104767766146,235.619449019235),
 .UNSPECIFIED.);
#3144=B_SPLINE_CURVE_WITH_KNOTS('',3,(#75095,#75096,#75097,#75098,#75099,
#75100,#75101,#75102,#75103,#75104),.UNSPECIFIED.,.F.,.F.,(4,1,1,1,1,1,
1,4),(223.053078404876,223.436708646671,224.435868920721,225.435029194772,
226.434189468823,227.433349742873,228.432510016924,229.336263712056),
 .UNSPECIFIED.);
#3145=B_SPLINE_CURVE_WITH_KNOTS('',3,(#75105,#75106,#75107,#75108,#75109,
#75110,#75111,#75112,#75113,#75114,#75115),.UNSPECIFIED.,.F.,.F.,(4,1,1,
1,1,1,1,1,4),(223.053078404876,223.114844477538,224.114004751588,225.113165025639,
226.11232529969,227.111485573741,228.110645847791,229.109806121842,229.336263712056),
 .UNSPECIFIED.);
#3146=B_SPLINE_CURVE_WITH_KNOTS('',3,(#75120,#75121,#75122,#75123,#75124,
#75125,#75126,#75127,#75128,#75129),.UNSPECIFIED.,.F.,.F.,(4,1,1,1,1,1,
1,4),(216.769893097696,217.441747002366,218.440907276417,219.440067550468,
220.439227824519,221.438388098569,222.43754837262,223.053078404876),
 .UNSPECIFIED.);
#3147=B_SPLINE_CURVE_WITH_KNOTS('',3,(#75130,#75131,#75132,#75133,#75134,
#75135,#75136,#75137,#75138,#75139),.UNSPECIFIED.,.F.,.F.,(4,1,1,1,1,1,
1,4),(216.769893097697,217.119882833234,218.119043107284,219.118203381335,
220.117363655386,221.116523929436,222.115684203487,223.053078404876),
 .UNSPECIFIED.);
#3148=B_SPLINE_CURVE_WITH_KNOTS('',3,(#75144,#75145,#75146,#75147,#75148,
#75149,#75150,#75151,#75152,#75153),.UNSPECIFIED.,.F.,.F.,(4,1,1,1,1,1,
1,4),(210.486707790517,211.446785358062,212.445945632113,213.445105906164,
214.444266180214,215.443426454265,216.442586728316,216.769893097696),
 .UNSPECIFIED.);
#3149=B_SPLINE_CURVE_WITH_KNOTS('',3,(#75154,#75155,#75156,#75157,#75158,
#75159,#75160,#75161,#75162,#75163),.UNSPECIFIED.,.F.,.F.,(4,1,1,1,1,1,
1,4),(210.486707790517,211.12492118893,212.12408146298,213.123241737031,
214.122402011082,215.121562285132,216.120722559183,216.769893097697),
 .UNSPECIFIED.);
#3150=B_SPLINE_CURVE_WITH_KNOTS('',3,(#75168,#75169,#75170,#75171,#75172,
#75173,#75174,#75175,#75176,#75177,#75178),.UNSPECIFIED.,.F.,.F.,(4,1,1,
1,1,1,1,1,4),(204.203522483337,204.452663439708,205.451823713758,206.450983987809,
207.45014426186,208.44930453591,209.448464809961,210.447625084012,210.486707790517),
 .UNSPECIFIED.);
#3151=B_SPLINE_CURVE_WITH_KNOTS('',3,(#75179,#75180,#75181,#75182,#75183,
#75184,#75185,#75186,#75187,#75188),.UNSPECIFIED.,.F.,.F.,(4,1,1,1,1,1,
1,4),(204.203522483338,205.129959544625,206.129119818676,207.128280092727,
208.127440366778,209.126600640828,210.125760914879,210.486707790517),
 .UNSPECIFIED.);
#3152=B_SPLINE_CURVE_WITH_KNOTS('',3,(#75193,#75194,#75195,#75196,#75197,
#75198,#75199,#75200,#75201,#75202),.UNSPECIFIED.,.F.,.F.,(4,1,1,1,1,1,
1,4),(197.920337176158,198.457701795403,199.456862069454,200.456022343505,
201.455182617555,202.454342891606,203.453503165657,204.203522483337),
 .UNSPECIFIED.);
#3153=B_SPLINE_CURVE_WITH_KNOTS('',3,(#75203,#75204,#75205,#75206,#75207,
#75208,#75209,#75210,#75211,#75212,#75213),.UNSPECIFIED.,.F.,.F.,(4,1,1,
1,1,1,1,1,4),(197.920337176158,198.135837626271,199.134997900321,200.134158174372,
201.133318448423,202.132478722473,203.131638996524,204.130799270575,204.203522483338),
 .UNSPECIFIED.);
#3154=B_SPLINE_CURVE_WITH_KNOTS('',3,(#75218,#75219,#75220,#75221,#75222,
#75223,#75224,#75225,#75226,#75227),.UNSPECIFIED.,.F.,.F.,(4,1,1,1,1,1,
1,4),(191.637151868978,192.462740151099,193.46190042515,194.461060699201,
195.460220973251,196.459381247302,197.458541521353,197.920337176158),
 .UNSPECIFIED.);
#3155=B_SPLINE_CURVE_WITH_KNOTS('',3,(#75228,#75229,#75230,#75231,#75232,
#75233,#75234,#75235,#75236,#75237),.UNSPECIFIED.,.F.,.F.,(4,1,1,1,1,1,
1,4),(191.637151868978,192.140875981967,193.140036256017,194.139196530068,
195.138356804119,196.137517078169,197.13667735222,197.920337176158),
 .UNSPECIFIED.);
#3156=B_SPLINE_CURVE_WITH_KNOTS('',3,(#75242,#75243,#75244,#75245,#75246,
#75247,#75248,#75249,#75250,#75251,#75252),.UNSPECIFIED.,.F.,.F.,(4,1,1,
1,1,1,1,1,4),(185.353966561799,185.468618232745,186.467778506795,187.466938780846,
188.466099054897,189.465259328947,190.464419602998,191.463579877049,191.637151868978),
 .UNSPECIFIED.);
#3157=B_SPLINE_CURVE_WITH_KNOTS('',3,(#75253,#75254,#75255,#75256,#75257,
#75258,#75259,#75260,#75261,#75262),.UNSPECIFIED.,.F.,.F.,(4,1,1,1,1,1,
1,4),(185.353966561799,186.145914337662,187.145074611713,188.144234885764,
189.143395159815,190.142555433865,191.141715707916,191.637151868978),
 .UNSPECIFIED.);
#3158=B_SPLINE_CURVE_WITH_KNOTS('',3,(#75267,#75268,#75269,#75270,#75271,
#75272,#75273,#75274,#75275,#75276),.UNSPECIFIED.,.F.,.F.,(4,1,1,1,1,1,
1,4),(179.070781254619,179.47365658844,180.472816862491,181.471977136542,
182.471137410592,183.470297684643,184.469457958694,185.353966561799),
 .UNSPECIFIED.);
#3159=B_SPLINE_CURVE_WITH_KNOTS('',3,(#75277,#75278,#75279,#75280,#75281,
#75282,#75283,#75284,#75285,#75286,#75287),.UNSPECIFIED.,.F.,.F.,(4,1,1,
1,1,1,1,1,4),(179.070781254619,179.151792419308,180.150952693358,181.150112967409,
182.14927324146,183.14843351551,184.147593789561,185.146754063612,185.353966561799),
 .UNSPECIFIED.);
#3160=B_SPLINE_CURVE_WITH_KNOTS('',3,(#75292,#75293,#75294,#75295,#75296,
#75297,#75298,#75299,#75300,#75301),.UNSPECIFIED.,.F.,.F.,(4,1,1,1,1,1,
1,4),(172.78759594744,173.478694944136,174.477855218187,175.477015492238,
176.476175766288,177.475336040339,178.47449631439,179.070781254619),
 .UNSPECIFIED.);
#3161=B_SPLINE_CURVE_WITH_KNOTS('',3,(#75302,#75303,#75304,#75305,#75306,
#75307,#75308,#75309,#75310,#75311),.UNSPECIFIED.,.F.,.F.,(4,1,1,1,1,1,
1,4),(172.78759594744,173.156830775004,174.155991049054,175.155151323105,
176.154311597156,177.153471871206,178.152632145257,179.070781254619),
 .UNSPECIFIED.);
#3162=B_SPLINE_CURVE_WITH_KNOTS('',3,(#75316,#75317,#75318,#75319,#75320,
#75321,#75322,#75323,#75324,#75325),.UNSPECIFIED.,.F.,.F.,(4,1,1,1,1,1,
1,4),(166.50441064026,167.483733299832,168.482893573883,169.482053847934,
170.481214121984,171.480374396035,172.479534670086,172.78759594744),
 .UNSPECIFIED.);
#3163=B_SPLINE_CURVE_WITH_KNOTS('',3,(#75326,#75327,#75328,#75329,#75330,
#75331,#75332,#75333,#75334,#75335),.UNSPECIFIED.,.F.,.F.,(4,1,1,1,1,1,
1,4),(166.50441064026,167.161869130699,168.16102940475,169.160189678801,
170.159349952851,171.158510226902,172.157670500953,172.78759594744),
 .UNSPECIFIED.);
#3164=B_SPLINE_CURVE_WITH_KNOTS('',3,(#75340,#75341,#75342,#75343,#75344,
#75345,#75346,#75347,#75348,#75349,#75350),.UNSPECIFIED.,.F.,.F.,(4,1,1,
1,1,1,1,1,4),(160.22122533308,160.489611381477,161.488771655528,162.487931929579,
163.487092203629,164.48625247768,165.485412751731,166.484573025782,166.50441064026),
 .UNSPECIFIED.);
#3165=B_SPLINE_CURVE_WITH_KNOTS('',3,(#75351,#75352,#75353,#75354,#75355,
#75356,#75357,#75358,#75359,#75360),.UNSPECIFIED.,.F.,.F.,(4,1,1,1,1,1,
1,4),(160.221225333081,161.166907486395,162.166067760446,163.165228034497,
164.164388308547,165.163548582598,166.162708856649,166.50441064026),
 .UNSPECIFIED.);
#3166=B_SPLINE_CURVE_WITH_KNOTS('',3,(#75365,#75366,#75367,#75368,#75369,
#75370,#75371,#75372,#75373,#75374),.UNSPECIFIED.,.F.,.F.,(4,1,1,1,1,1,
1,4),(153.938040025901,154.494649737173,155.493810011224,156.492970285275,
157.492130559325,158.491290833376,159.490451107427,160.22122533308),
 .UNSPECIFIED.);
#3167=B_SPLINE_CURVE_WITH_KNOTS('',3,(#75375,#75376,#75377,#75378,#75379,
#75380,#75381,#75382,#75383,#75384,#75385),.UNSPECIFIED.,.F.,.F.,(4,1,1,
1,1,1,1,1,4),(153.938040025901,154.172785568041,155.171945842091,156.171106116142,
157.170266390193,158.169426664243,159.168586938294,160.167747212345,160.221225333081),
 .UNSPECIFIED.);
#3168=B_SPLINE_CURVE_WITH_KNOTS('',3,(#75390,#75391,#75392,#75393,#75394,
#75395,#75396,#75397,#75398,#75399),.UNSPECIFIED.,.F.,.F.,(4,1,1,1,1,1,
1,4),(147.654854718721,148.499688092869,149.49884836692,150.498008640971,
151.497168915021,152.496329189072,153.495489463123,153.938040025901),
 .UNSPECIFIED.);
#3169=B_SPLINE_CURVE_WITH_KNOTS('',3,(#75400,#75401,#75402,#75403,#75404,
#75405,#75406,#75407,#75408,#75409),.UNSPECIFIED.,.F.,.F.,(4,1,1,1,1,1,
1,4),(147.654854718721,148.177823923736,149.176984197787,150.176144471838,
151.175304745888,152.174465019939,153.17362529399,153.938040025901),
 .UNSPECIFIED.);
#3170=B_SPLINE_CURVE_WITH_KNOTS('',3,(#75414,#75415,#75416,#75417,#75418,
#75419,#75420,#75421,#75422,#75423,#75424),.UNSPECIFIED.,.F.,.F.,(4,1,1,
1,1,1,1,1,4),(141.371669411542,141.505566174514,142.504726448565,143.503886722616,
144.503046996666,145.502207270717,146.501367544768,147.500527818819,147.654854718721),
 .UNSPECIFIED.);
#3171=B_SPLINE_CURVE_WITH_KNOTS('',3,(#75425,#75426,#75427,#75428,#75429,
#75430,#75431,#75432,#75433,#75434),.UNSPECIFIED.,.F.,.F.,(4,1,1,1,1,1,
1,4),(141.371669411542,142.182862279432,143.182022553483,144.181182827534,
145.180343101584,146.179503375635,147.178663649686,147.654854718721),
 .UNSPECIFIED.);
#3172=B_SPLINE_CURVE_WITH_KNOTS('',3,(#75439,#75440,#75441,#75442,#75443,
#75444,#75445,#75446,#75447,#75448),.UNSPECIFIED.,.F.,.F.,(4,1,1,1,1,1,
1,4),(135.088484104362,135.51060453021,136.509764804261,137.508925078312,
138.508085352362,139.507245626413,140.506405900464,141.371669411542),
 .UNSPECIFIED.);
#3173=B_SPLINE_CURVE_WITH_KNOTS('',3,(#75449,#75450,#75451,#75452,#75453,
#75454,#75455,#75456,#75457,#75458,#75459),.UNSPECIFIED.,.F.,.F.,(4,1,1,
1,1,1,1,1,4),(135.088484104362,135.188740361078,136.187900635128,137.187060909179,
138.18622118323,139.18538145728,140.184541731331,141.183702005382,141.371669411542),
 .UNSPECIFIED.);
#3174=B_SPLINE_CURVE_WITH_KNOTS('',3,(#75464,#75465,#75466,#75467,#75468,
#75469,#75470,#75471,#75472,#75473),.UNSPECIFIED.,.F.,.F.,(4,1,1,1,1,1,
1,4),(128.805298797183,129.515642885906,130.514803159957,131.513963434008,
132.513123708058,133.512283982109,134.51144425616,135.088484104362),
 .UNSPECIFIED.);
#3175=B_SPLINE_CURVE_WITH_KNOTS('',3,(#75474,#75475,#75476,#75477,#75478,
#75479,#75480,#75481,#75482,#75483),.UNSPECIFIED.,.F.,.F.,(4,1,1,1,1,1,
1,4),(128.805298797183,129.193778716773,130.192938990824,131.192099264875,
132.191259538925,133.190419812976,134.189580087027,135.088484104362),
 .UNSPECIFIED.);
#3176=B_SPLINE_CURVE_WITH_KNOTS('',3,(#75488,#75489,#75490,#75491,#75492,
#75493,#75494,#75495,#75496,#75497),.UNSPECIFIED.,.F.,.F.,(4,1,1,1,1,1,
1,4),(122.522113490003,123.520681241602,124.519841515653,125.519001789703,
126.518162063754,127.517322337805,128.516482611855,128.805298797183),
 .UNSPECIFIED.);
#3177=B_SPLINE_CURVE_WITH_KNOTS('',3,(#75498,#75499,#75500,#75501,#75502,
#75503,#75504,#75505,#75506,#75507),.UNSPECIFIED.,.F.,.F.,(4,1,1,1,1,1,
1,4),(122.522113490003,123.198817072469,124.19797734652,125.197137620571,
126.196297894621,127.195458168672,128.194618442723,128.805298797183),
 .UNSPECIFIED.);
#3178=B_SPLINE_CURVE_WITH_KNOTS('',3,(#75512,#75513,#75514,#75515,#75516,
#75517,#75518,#75519,#75520,#75521,#75522),.UNSPECIFIED.,.F.,.F.,(4,1,1,
1,1,1,1,1,4),(116.238928182823,116.526559323247,117.525719597298,118.524879871349,
119.524040145399,120.52320041945,121.522360693501,122.521520967551,122.522113490003),
 .UNSPECIFIED.);
#3179=B_SPLINE_CURVE_WITH_KNOTS('',3,(#75523,#75524,#75525,#75526,#75527,
#75528,#75529,#75530,#75531,#75532),.UNSPECIFIED.,.F.,.F.,(4,1,1,1,1,1,
1,4),(116.238928182824,117.203855428165,118.203015702216,119.202175976267,
120.201336250317,121.200496524368,122.199656798419,122.522113490003),
 .UNSPECIFIED.);
#3180=B_SPLINE_CURVE_WITH_KNOTS('',3,(#75537,#75538,#75539,#75540,#75541,
#75542,#75543,#75544,#75545,#75546),.UNSPECIFIED.,.F.,.F.,(4,1,1,1,1,1,
1,4),(109.955742875644,110.531597678943,111.530757952994,112.529918227045,
113.529078501095,114.528238775146,115.527399049197,116.238928182823),
 .UNSPECIFIED.);
#3181=B_SPLINE_CURVE_WITH_KNOTS('',3,(#75547,#75548,#75549,#75550,#75551,
#75552,#75553,#75554,#75555,#75556,#75557),.UNSPECIFIED.,.F.,.F.,(4,1,1,
1,1,1,1,1,4),(109.955742875644,110.20973350981,111.208893783861,112.208054057912,
113.207214331962,114.206374606013,115.205534880064,116.204695154114,116.238928182824),
 .UNSPECIFIED.);
#3182=B_SPLINE_CURVE_WITH_KNOTS('',3,(#75562,#75563,#75564,#75565,#75566,
#75567,#75568,#75569,#75570,#75571),.UNSPECIFIED.,.F.,.F.,(4,1,1,1,1,1,
1,4),(103.672557568464,104.536636034639,105.53579630869,106.53495658274,
107.534116856791,108.533277130842,109.532437404892,109.955742875644),
 .UNSPECIFIED.);
#3183=B_SPLINE_CURVE_WITH_KNOTS('',3,(#75572,#75573,#75574,#75575,#75576,
#75577,#75578,#75579,#75580,#75581),.UNSPECIFIED.,.F.,.F.,(4,1,1,1,1,1,
1,4),(103.672557568464,104.214771865506,105.213932139557,106.213092413608,
107.212252687658,108.211412961709,109.21057323576,109.955742875644),
 .UNSPECIFIED.);
#3184=B_SPLINE_CURVE_WITH_KNOTS('',3,(#75586,#75587,#75588,#75589,#75590,
#75591,#75592,#75593,#75594,#75595,#75596),.UNSPECIFIED.,.F.,.F.,(4,1,1,
1,1,1,1,1,4),(97.3893722612846,97.5425141162843,98.5416743903349,99.5408346643856,
100.539994938436,101.539155212487,102.538315486538,103.537475760588,103.672557568464),
 .UNSPECIFIED.);
#3185=B_SPLINE_CURVE_WITH_KNOTS('',3,(#75597,#75598,#75599,#75600,#75601,
#75602,#75603,#75604,#75605,#75606),.UNSPECIFIED.,.F.,.F.,(4,1,1,1,1,1,
1,4),(97.3893722612848,98.2198102212022,99.2189704952528,100.218130769304,
101.217291043354,102.216451317405,103.215611591456,103.672557568464),
 .UNSPECIFIED.);
#3186=B_SPLINE_CURVE_WITH_KNOTS('',3,(#75611,#75612,#75613,#75614,#75615,
#75616,#75617,#75618,#75619,#75620),.UNSPECIFIED.,.F.,.F.,(4,1,1,1,1,1,
1,4),(91.106186954105,91.5475524719801,92.5467127460308,93.5458730200815,
94.5450332941322,95.5441935681829,96.5433538422336,97.3893722612846),
 .UNSPECIFIED.);
#3187=B_SPLINE_CURVE_WITH_KNOTS('',3,(#75621,#75622,#75623,#75624,#75625,
#75626,#75627,#75628,#75629,#75630,#75631),.UNSPECIFIED.,.F.,.F.,(4,1,1,
1,1,1,1,1,4),(91.1061869541051,91.2256883028474,92.2248485768981,93.2240088509487,
94.2231691249994,95.2223293990501,96.2214896731008,97.2206499471515,97.3893722612848),
 .UNSPECIFIED.);
#3188=B_SPLINE_CURVE_WITH_KNOTS('',3,(#75636,#75637,#75638,#75639,#75640,
#75641,#75642,#75643,#75644,#75645),.UNSPECIFIED.,.F.,.F.,(4,1,1,1,1,1,
1,4),(84.8230016469254,85.552590827676,86.5517511017267,87.5509113757774,
88.5500716498281,89.5492319238788,90.5483921979294,91.106186954105),
 .UNSPECIFIED.);
#3189=B_SPLINE_CURVE_WITH_KNOTS('',3,(#75646,#75647,#75648,#75649,#75650,
#75651,#75652,#75653,#75654,#75655),.UNSPECIFIED.,.F.,.F.,(4,1,1,1,1,1,
1,4),(84.8230016469256,85.2307266585432,86.2298869325939,87.2290472066446,
88.2282074806953,89.227367754746,90.2265280287967,91.1061869541051),
 .UNSPECIFIED.);
#3190=B_SPLINE_CURVE_WITH_KNOTS('',3,(#75660,#75661,#75662,#75663,#75664,
#75665,#75666,#75667,#75668,#75669,#75670),.UNSPECIFIED.,.F.,.F.,(4,1,1,
1,1,1,1,1,4),(78.5398163397459,78.5584689093212,79.5576291833719,80.5567894574226,
81.5559497314733,82.555110005524,83.5542702795747,84.5534305536253,84.8230016469254),
 .UNSPECIFIED.);
#3191=B_SPLINE_CURVE_WITH_KNOTS('',3,(#75671,#75672,#75673,#75674,#75675,
#75676,#75677,#75678,#75679,#75680),.UNSPECIFIED.,.F.,.F.,(4,1,1,1,1,1,
1,4),(78.539816339746,79.2357650142391,80.2349252882898,81.2340855623405,
82.2332458363912,83.2324061104419,84.2315663844926,84.8230016469256),
 .UNSPECIFIED.);
#3192=B_SPLINE_CURVE_WITH_KNOTS('',3,(#75685,#75686,#75687,#75688,#75689,
#75690,#75691,#75692,#75693,#75694),.UNSPECIFIED.,.F.,.F.,(4,1,1,1,1,1,
1,4),(72.2566310325663,72.5635072650171,73.5626675390678,74.5618278131185,
75.5609880871692,76.5601483612199,77.5593086352705,78.5398163397459),
 .UNSPECIFIED.);
#3193=B_SPLINE_CURVE_WITH_KNOTS('',3,(#75695,#75696,#75697,#75698,#75699,
#75700,#75701,#75702,#75703,#75704),.UNSPECIFIED.,.F.,.F.,(4,1,1,1,1,1,
1,4),(72.2566310325664,73.240803369935,74.2399636439857,75.2391239180364,
76.2382841920871,77.2374444661378,78.2366047401885,78.539816339746),
 .UNSPECIFIED.);
#3194=B_SPLINE_CURVE_WITH_KNOTS('',3,(#75709,#75710,#75711,#75712,#75713,
#75714,#75715,#75716,#75717,#75718),.UNSPECIFIED.,.F.,.F.,(4,1,1,1,1,1,
1,4),(65.9734457253867,66.568545620713,67.5677058947637,68.5668661688144,
69.5660264428651,70.5651867169157,71.5643469909664,72.2566310325663),
 .UNSPECIFIED.);
#3195=B_SPLINE_CURVE_WITH_KNOTS('',3,(#75719,#75720,#75721,#75722,#75723,
#75724,#75725,#75726,#75727,#75728,#75729),.UNSPECIFIED.,.F.,.F.,(4,1,1,
1,1,1,1,1,4),(65.9734457253868,66.2466814515802,67.2458417256309,68.2450019996816,
69.2441622737323,70.243322547783,71.2424828218336,72.2416430958843,72.2566310325664),
 .UNSPECIFIED.);
#3196=B_SPLINE_CURVE_WITH_KNOTS('',3,(#75734,#75735,#75736,#75737,#75738,
#75739,#75740,#75741,#75742,#75743),.UNSPECIFIED.,.F.,.F.,(4,1,1,1,1,1,
1,4),(59.6902604182071,60.5735839764089,61.5727442504596,62.5719045245103,
63.5710647985609,64.5702250726116,65.5693853466623,65.9734457253867),
 .UNSPECIFIED.);
#3197=B_SPLINE_CURVE_WITH_KNOTS('',3,(#75744,#75745,#75746,#75747,#75748,
#75749,#75750,#75751,#75752,#75753),.UNSPECIFIED.,.F.,.F.,(4,1,1,1,1,1,
1,4),(59.6902604182072,60.2517198072761,61.2508800813268,62.2500403553775,
63.2492006294282,64.2483609034789,65.2475211775295,65.9734457253868),
 .UNSPECIFIED.);
#3198=B_SPLINE_CURVE_WITH_KNOTS('',3,(#75758,#75759,#75760,#75761,#75762,
#75763,#75764,#75765,#75766,#75767,#75768),.UNSPECIFIED.,.F.,.F.,(4,1,1,
1,1,1,1,1,4),(53.4070751110275,53.5794620580541,54.5786223321048,55.5777826061555,
56.5769428802061,57.5761031542568,58.5752634283075,59.5744237023582,59.6902604182071),
 .UNSPECIFIED.);
#3199=B_SPLINE_CURVE_WITH_KNOTS('',3,(#75769,#75770,#75771,#75772,#75773,
#75774,#75775,#75776,#75777,#75778),.UNSPECIFIED.,.F.,.F.,(4,1,1,1,1,1,
1,4),(53.4070751110276,54.256758162972,55.2559184370227,56.2550787110734,
57.2542389851241,58.2533992591747,59.2525595332254,59.6902604182072),
 .UNSPECIFIED.);
#3200=B_SPLINE_CURVE_WITH_KNOTS('',3,(#75783,#75784,#75785,#75786,#75787,
#75788,#75789,#75790,#75791,#75792),.UNSPECIFIED.,.F.,.F.,(4,1,1,1,1,1,
1,4),(47.1238898038479,47.58450041375,48.5836606878007,49.5828209618514,
50.581981235902,51.5811415099527,52.5803017840034,53.4070751110275),
 .UNSPECIFIED.);
#3201=B_SPLINE_CURVE_WITH_KNOTS('',3,(#75793,#75794,#75795,#75796,#75797,
#75798,#75799,#75800,#75801,#75802,#75803),.UNSPECIFIED.,.F.,.F.,(4,1,1,
1,1,1,1,1,4),(47.123889803848,47.2626362446172,48.2617965186679,49.2609567927186,
50.2601170667693,51.2592773408199,52.2584376148706,53.2575978889213,53.4070751110276),
 .UNSPECIFIED.);
#3202=B_SPLINE_CURVE_WITH_KNOTS('',3,(#75808,#75809,#75810,#75811,#75812,
#75813,#75814,#75815,#75816,#75817),.UNSPECIFIED.,.F.,.F.,(4,1,1,1,1,1,
1,4),(40.8407044966683,41.5895387694459,42.5886990434966,43.5878593175472,
44.5870195915979,45.5861798656486,46.5853401396993,47.1238898038479),
 .UNSPECIFIED.);
#3203=B_SPLINE_CURVE_WITH_KNOTS('',3,(#75818,#75819,#75820,#75821,#75822,
#75823,#75824,#75825,#75826,#75827),.UNSPECIFIED.,.F.,.F.,(4,1,1,1,1,1,
1,4),(40.8407044966684,41.2676746003131,42.2668348743638,43.2659951484145,
44.2651554224651,45.2643156965158,46.2634759705665,47.123889803848),
 .UNSPECIFIED.);
#3204=B_SPLINE_CURVE_WITH_KNOTS('',3,(#75832,#75833,#75834,#75835,#75836,
#75837,#75838,#75839,#75840,#75841,#75842),.UNSPECIFIED.,.F.,.F.,(4,1,1,
1,1,1,1,1,4),(34.5575191894887,34.5954168510911,35.5945771251418,36.5937373991924,
37.5928976732431,38.5920579472938,39.5912182213445,40.5903784953952,40.8407044966683),
 .UNSPECIFIED.);
#3205=B_SPLINE_CURVE_WITH_KNOTS('',3,(#75843,#75844,#75845,#75846,#75847,
#75848,#75849,#75850,#75851,#75852),.UNSPECIFIED.,.F.,.F.,(4,1,1,1,1,1,
1,4),(34.5575191894888,35.272712956009,36.2718732300597,37.2710335041103,
38.270193778161,39.2693540522117,40.2685143262624,40.8407044966684),
 .UNSPECIFIED.);
#3206=B_SPLINE_CURVE_WITH_KNOTS('',3,(#75857,#75858,#75859,#75860,#75861,
#75862,#75863,#75864,#75865,#75866),.UNSPECIFIED.,.F.,.F.,(4,1,1,1,1,1,
1,4),(28.2743338823091,28.600455206787,29.5996154808376,30.5987757548883,
31.597936028939,32.5970963029897,33.5962565770404,34.5575191894887),
 .UNSPECIFIED.);
#3207=B_SPLINE_CURVE_WITH_KNOTS('',3,(#75867,#75868,#75869,#75870,#75871,
#75872,#75873,#75874,#75875,#75876,#75877),.UNSPECIFIED.,.F.,.F.,(4,1,1,
1,1,1,1,1,4),(28.2743338823092,28.2785910376542,29.2777513117049,30.2769115857556,
31.2760718598062,32.2752321338569,33.2743924079076,34.2735526819583,34.5575191894888),
 .UNSPECIFIED.);
#3208=B_SPLINE_CURVE_WITH_KNOTS('',3,(#75882,#75883,#75884,#75885,#75886,
#75887,#75888,#75889,#75890,#75891),.UNSPECIFIED.,.F.,.F.,(4,1,1,1,1,1,
1,4),(21.9911485751295,22.6054935624829,23.6046538365335,24.6038141105842,
25.6029743846349,26.6021346586856,27.6012949327363,28.2743338823091),
 .UNSPECIFIED.);
#3209=B_SPLINE_CURVE_WITH_KNOTS('',3,(#75892,#75893,#75894,#75895,#75896,
#75897,#75898,#75899,#75900,#75901),.UNSPECIFIED.,.F.,.F.,(4,1,1,1,1,1,
1,4),(21.9911485751297,22.2836293933501,23.2827896674008,24.2819499414514,
25.2811102155021,26.2802704895528,27.2794307636035,28.2743338823092),
 .UNSPECIFIED.);
#3210=B_SPLINE_CURVE_WITH_KNOTS('',3,(#75906,#75907,#75908,#75909,#75910,
#75911,#75912,#75913,#75914,#75915),.UNSPECIFIED.,.F.,.F.,(4,1,1,1,1,1,
1,4),(15.70796326795,16.6105319181787,17.6096921922294,18.6088524662801,
19.6080127403308,20.6071730143815,21.6063332884322,21.9911485751295),
 .UNSPECIFIED.);
#3211=B_SPLINE_CURVE_WITH_KNOTS('',3,(#75916,#75917,#75918,#75919,#75920,
#75921,#75922,#75923,#75924,#75925),.UNSPECIFIED.,.F.,.F.,(4,1,1,1,1,1,
1,4),(15.7079632679501,16.288667749046,17.2878280230966,18.2869882971473,
19.286148571198,20.2853088452487,21.2844691192994,21.9911485751297),
 .UNSPECIFIED.);
#3212=B_SPLINE_CURVE_WITH_KNOTS('',3,(#75928,#75929,#75930,#75931,#75932,
#75933,#75934,#75935,#75936,#75937,#75938,#75939,#75940,#75941,#75942,#75943,
#75944,#75945,#75946,#75947,#75948,#75949,#75950,#75951,#75952,#75953,#75954,
#75955,#75956,#75957,#75958,#75959,#75960,#75961,#75962,#75963,#75964,#75965,
#75966,#75967,#75968,#75969,#75970,#75971,#75972,#75973,#75974,#75975,#75976,
#75977,#75978,#75979,#75980,#75981,#75982,#75983,#75984,#75985,#75986,#75987,
#75988,#75989,#75990,#75991,#75992,#75993,#75994,#75995,#75996,#75997,#75998,
#75999,#76000,#76001,#76002,#76003,#76004,#76005,#76006,#76007,#76008,#76009,
#76010,#76011,#76012,#76013,#76014,#76015,#76016,#76017,#76018,#76019,#76020,
#76021,#76022,#76023,#76024,#76025,#76026,#76027,#76028,#76029,#76030,#76031,
#76032,#76033),.UNSPECIFIED.,.F.,.F.,(4,3,3,3,3,3,3,3,3,3,3,3,3,3,3,3,3,
3,3,3,3,3,3,3,3,3,3,3,3,3,3,3,3,3,3,4),(-0.990745149397272,-0.953116208297139,
-0.912523111179552,-0.885921211171593,-0.874931108620643,-0.86587654099025,
-0.824728242628866,-0.782498801181784,-0.764023420548686,-0.749177983835952,
-0.743080509582649,-0.700694026797518,-0.657915923258967,-0.615160120207279,
-0.583093267918513,-0.569303123526439,-0.56234430900736,-0.519192848994169,
-0.486892711052215,-0.444701478410969,-0.401945206516134,-0.389788368451242,
-0.382758910740908,-0.376896545121776,-0.334227892709294,-0.290071518416692,
-0.245915144124089,-0.215175751108578,-0.20168695137348,-0.194154816283721,
-0.188100426560717,-0.144404214510165,-0.100314778095157,-0.0563889878319668,
-0.0131683088431834,0.),.UNSPECIFIED.);
#3213=B_SPLINE_CURVE_WITH_KNOTS('',3,(#76038,#76039,#76040,#76041,#76042,
#76043,#76044,#76045,#76046,#76047,#76048,#76049,#76050,#76051,#76052,#76053,
#76054,#76055,#76056,#76057,#76058,#76059,#76060,#76061,#76062,#76063,#76064,
#76065,#76066,#76067,#76068,#76069,#76070,#76071,#76072,#76073,#76074,#76075,
#76076,#76077,#76078,#76079,#76080,#76081,#76082,#76083,#76084,#76085,#76086,
#76087,#76088,#76089,#76090,#76091,#76092,#76093,#76094,#76095,#76096,#76097,
#76098,#76099,#76100,#76101,#76102,#76103,#76104,#76105,#76106,#76107,#76108,
#76109,#76110,#76111,#76112,#76113,#76114,#76115,#76116,#76117,#76118,#76119,
#76120,#76121,#76122,#76123,#76124,#76125,#76126,#76127,#76128,#76129,#76130,
#76131,#76132,#76133,#76134,#76135,#76136,#76137,#76138,#76139,#76140,#76141,
#76142,#76143,#76144,#76145,#76146),.UNSPECIFIED.,.F.,.F.,(4,3,3,3,3,3,
3,3,3,3,3,3,3,3,3,3,3,3,3,3,3,3,3,3,3,3,3,3,3,3,3,3,3,3,3,3,4),(-0.988861763753148,
-0.947944861719371,-0.904266293393393,-0.876752649619069,-0.860521193082487,
-0.854366172475187,-0.810876688531655,-0.767523101590724,-0.747924850769826,
-0.737059406202786,-0.730926332354279,-0.724875966528802,-0.681346469766453,
-0.637840230036599,-0.594392170778502,-0.561806126334929,-0.548626870943788,
-0.543243028328661,-0.500823502880395,-0.46404799300421,-0.421566751277432,
-0.378898569390552,-0.365114758790781,-0.359674607894455,-0.353937374020393,
-0.31200686520388,-0.269901000253992,-0.229433896916033,-0.200754659801529,
-0.187320188163563,-0.179359914434182,-0.174478120366766,-0.130858590275074,
-0.0893323551625696,-0.0481739323171706,-0.00783840924613729,0.),
 .UNSPECIFIED.);
#3214=B_SPLINE_CURVE_WITH_KNOTS('',3,(#78059,#78060,#78061,#78062,#78063,
#78064,#78065,#78066,#78067,#78068,#78069,#78070,#78071,#78072,#78073,#78074),
 .UNSPECIFIED.,.F.,.F.,(4,3,3,3,3,4),(466.085105135419,466.60784798167,
467.607008255721,468.606168529772,469.605328803822,470.521777155409),
 .UNSPECIFIED.);
#3215=B_SPLINE_CURVE_WITH_KNOTS('',3,(#78076,#78077,#78078,#78079,#78080,
#78081,#78082,#78083,#78084,#78085,#78086,#78087,#78088,#78089,#78090,#78091,
#78092,#78093,#78094,#78095,#78096,#78097,#78098,#78099,#78100,#78101,#78102,
#78103,#78104,#78105,#78106,#78107,#78108,#78109,#78110,#78111,#78112,#78113,
#78114,#78115,#78116,#78117,#78118,#78119,#78120,#78121,#78122,#78123,#78124,
#78125,#78126,#78127,#78128,#78129,#78130,#78131,#78132,#78133,#78134,#78135,
#78136,#78137,#78138,#78139,#78140,#78141,#78142,#78143,#78144,#78145,#78146,
#78147,#78148,#78149,#78150,#78151,#78152,#78153,#78154,#78155,#78156,#78157,
#78158,#78159,#78160,#78161,#78162,#78163,#78164,#78165,#78166,#78167,#78168,
#78169,#78170,#78171,#78172,#78173,#78174,#78175,#78176,#78177,#78178,#78179,
#78180,#78181),.UNSPECIFIED.,.F.,.F.,(4,3,3,3,3,3,3,3,3,3,3,3,3,3,3,3,3,
3,3,3,3,3,3,3,3,3,3,3,3,3,3,3,3,3,3,4),(-0.990745149397179,-0.953116208297015,
-0.912523118726293,-0.885921218246659,-0.87493112265529,-0.865876539744951,
-0.824728248358261,-0.782498806194998,-0.76402342524857,-0.749177977734278,
-0.743080507741458,-0.700694026269302,-0.657915914033916,-0.615160113288475,
-0.583093262729394,-0.569303115883233,-0.562344307517487,-0.519192825285289,
-0.486892711052151,-0.444701445163227,-0.401945182425889,-0.389788318046496,
-0.382757232744068,-0.376896437396706,-0.334227749510469,-0.290071446817269,
-0.24591514412407,-0.215175751108561,-0.201686951004493,-0.194154818601853,
-0.188100426670343,-0.144404320209132,-0.100314907674269,-0.0563891000384953,
-0.0131683692741428,0.),.UNSPECIFIED.);
#3216=B_SPLINE_CURVE_WITH_KNOTS('',3,(#78182,#78183,#78184,#78185,#78186,
#78187,#78188,#78189,#78190),.UNSPECIFIED.,.F.,.F.,(4,1,1,1,1,1,4),(10.3764180272052,
11.2928663787925,12.2920266528432,13.2911869268939,14.2903472009446,15.2895074749953,
15.7079632679501),.UNSPECIFIED.);
#3217=B_SPLINE_CURVE_WITH_KNOTS('',3,(#78196,#78197,#78198,#78199,#78200,
#78201,#78202,#78203,#78204,#78205,#78206,#78207,#78208,#78209,#78210,#78211,
#78212,#78213,#78214,#78215,#78216,#78217,#78218,#78219,#78220,#78221,#78222,
#78223,#78224,#78225,#78226,#78227,#78228,#78229,#78230,#78231,#78232,#78233,
#78234,#78235,#78236,#78237,#78238,#78239,#78240,#78241,#78242,#78243,#78244,
#78245,#78246,#78247,#78248,#78249,#78250,#78251,#78252,#78253,#78254,#78255,
#78256,#78257,#78258,#78259,#78260,#78261,#78262,#78263,#78264,#78265,#78266,
#78267,#78268,#78269,#78270,#78271,#78272,#78273,#78274,#78275,#78276,#78277,
#78278,#78279,#78280,#78281,#78282,#78283,#78284,#78285,#78286,#78287,#78288,
#78289,#78290,#78291,#78292,#78293,#78294,#78295,#78296,#78297,#78298,#78299,
#78300,#78301,#78302,#78303,#78304),.UNSPECIFIED.,.F.,.F.,(4,3,3,3,3,3,
3,3,3,3,3,3,3,3,3,3,3,3,3,3,3,3,3,3,3,3,3,3,3,3,3,3,3,3,3,3,4),(-0.988861763753244,
-0.947944861719434,-0.904266288020023,-0.876752644581534,-0.860521185641252,
-0.854366163559061,-0.810876676220037,-0.767523090818058,-0.747924853089199,
-0.737059410276204,-0.730926341162295,-0.724875968929562,-0.681346480687655,
-0.637840262092946,-0.59439219482076,-0.56180614436662,-0.54862689554501,
-0.543243028959436,-0.500823535537494,-0.4640479930042,-0.4215667470188,
-0.378898519968392,-0.365114586359317,-0.359674094222405,-0.353937304897961,
-0.312006788845363,-0.269900865492287,-0.229433896916071,-0.200754659801562,
-0.187320188967778,-0.179359911830878,-0.17447811560387,-0.130858586702903,
-0.0893323660352711,-0.0481739755722922,-0.00783848836599452,0.),
 .UNSPECIFIED.);
#3218=B_SPLINE_CURVE_WITH_KNOTS('',3,(#78307,#78308,#78309,#78310,#78311,
#78312,#78313,#78314,#78315),.UNSPECIFIED.,.F.,.F.,(4,1,1,1,1,1,4),(11.6147305479253,
12.1143106849507,12.613890821976,13.6130510960267,14.6122113700774,15.6113716441281,
15.70796326795),.UNSPECIFIED.);
#3219=B_SPLINE_CURVE_WITH_KNOTS('',3,(#80228,#80229,#80230,#80231,#80232,
#80233,#80234,#80235,#80236,#80237,#80238,#80239,#80240,#80241,#80242,#80243),
 .UNSPECIFIED.,.F.,.F.,(4,3,3,3,3,4),(-472.602809625974,-472.103229488949,
-471.603649351923,-470.604489077873,-469.605328803822,-469.048945451313),
 .UNSPECIFIED.);
#3572=FACE_BOUND('',#7249,.T.);
#5044=FACE_OUTER_BOUND('',#7088,.T.);
#5045=FACE_OUTER_BOUND('',#7089,.T.);
#5046=FACE_OUTER_BOUND('',#7090,.T.);
#5047=FACE_OUTER_BOUND('',#7091,.T.);
#5048=FACE_OUTER_BOUND('',#7092,.T.);
#5049=FACE_OUTER_BOUND('',#7093,.T.);
#5050=FACE_OUTER_BOUND('',#7094,.T.);
#5051=FACE_OUTER_BOUND('',#7095,.T.);
#5052=FACE_OUTER_BOUND('',#7096,.T.);
#5053=FACE_OUTER_BOUND('',#7097,.T.);
#5054=FACE_OUTER_BOUND('',#7098,.T.);
#5055=FACE_OUTER_BOUND('',#7099,.T.);
#5056=FACE_OUTER_BOUND('',#7100,.T.);
#5057=FACE_OUTER_BOUND('',#7101,.T.);
#5058=FACE_OUTER_BOUND('',#7102,.T.);
#5059=FACE_OUTER_BOUND('',#7103,.T.);
#5060=FACE_OUTER_BOUND('',#7104,.T.);
#5061=FACE_OUTER_BOUND('',#7105,.T.);
#5062=FACE_OUTER_BOUND('',#7106,.T.);
#5063=FACE_OUTER_BOUND('',#7107,.T.);
#5064=FACE_OUTER_BOUND('',#7108,.T.);
#5065=FACE_OUTER_BOUND('',#7109,.T.);
#5066=FACE_OUTER_BOUND('',#7110,.T.);
#5067=FACE_OUTER_BOUND('',#7111,.T.);
#5068=FACE_OUTER_BOUND('',#7112,.T.);
#5069=FACE_OUTER_BOUND('',#7113,.T.);
#5070=FACE_OUTER_BOUND('',#7114,.T.);
#5071=FACE_OUTER_BOUND('',#7115,.T.);
#5072=FACE_OUTER_BOUND('',#7116,.T.);
#5073=FACE_OUTER_BOUND('',#7117,.T.);
#5074=FACE_OUTER_BOUND('',#7118,.T.);
#5075=FACE_OUTER_BOUND('',#7119,.T.);
#5076=FACE_OUTER_BOUND('',#7120,.T.);
#5077=FACE_OUTER_BOUND('',#7121,.T.);
#5078=FACE_OUTER_BOUND('',#7122,.T.);
#5079=FACE_OUTER_BOUND('',#7123,.T.);
#5080=FACE_OUTER_BOUND('',#7124,.T.);
#5081=FACE_OUTER_BOUND('',#7125,.T.);
#5082=FACE_OUTER_BOUND('',#7126,.T.);
#5083=FACE_OUTER_BOUND('',#7127,.T.);
#5084=FACE_OUTER_BOUND('',#7128,.T.);
#5085=FACE_OUTER_BOUND('',#7129,.T.);
#5086=FACE_OUTER_BOUND('',#7130,.T.);
#5087=FACE_OUTER_BOUND('',#7131,.T.);
#5088=FACE_OUTER_BOUND('',#7132,.T.);
#5089=FACE_OUTER_BOUND('',#7133,.T.);
#5090=FACE_OUTER_BOUND('',#7134,.T.);
#5091=FACE_OUTER_BOUND('',#7135,.T.);
#5092=FACE_OUTER_BOUND('',#7136,.T.);
#5093=FACE_OUTER_BOUND('',#7137,.T.);
#5094=FACE_OUTER_BOUND('',#7138,.T.);
#5095=FACE_OUTER_BOUND('',#7139,.T.);
#5096=FACE_OUTER_BOUND('',#7140,.T.);
#5097=FACE_OUTER_BOUND('',#7141,.T.);
#5098=FACE_OUTER_BOUND('',#7142,.T.);
#5099=FACE_OUTER_BOUND('',#7143,.T.);
#5100=FACE_OUTER_BOUND('',#7144,.T.);
#5101=FACE_OUTER_BOUND('',#7145,.T.);
#5102=FACE_OUTER_BOUND('',#7146,.T.);
#5103=FACE_OUTER_BOUND('',#7147,.T.);
#5104=FACE_OUTER_BOUND('',#7148,.T.);
#5105=FACE_OUTER_BOUND('',#7149,.T.);
#5106=FACE_OUTER_BOUND('',#7150,.T.);
#5107=FACE_OUTER_BOUND('',#7151,.T.);
#5108=FACE_OUTER_BOUND('',#7152,.T.);
#5109=FACE_OUTER_BOUND('',#7153,.T.);
#5110=FACE_OUTER_BOUND('',#7154,.T.);
#5111=FACE_OUTER_BOUND('',#7155,.T.);
#5112=FACE_OUTER_BOUND('',#7156,.T.);
#5113=FACE_OUTER_BOUND('',#7157,.T.);
#5114=FACE_OUTER_BOUND('',#7158,.T.);
#5115=FACE_OUTER_BOUND('',#7159,.T.);
#5116=FACE_OUTER_BOUND('',#7160,.T.);
#5117=FACE_OUTER_BOUND('',#7161,.T.);
#5118=FACE_OUTER_BOUND('',#7162,.T.);
#5119=FACE_OUTER_BOUND('',#7163,.T.);
#5120=FACE_OUTER_BOUND('',#7164,.T.);
#5121=FACE_OUTER_BOUND('',#7165,.T.);
#5122=FACE_OUTER_BOUND('',#7166,.T.);
#5123=FACE_OUTER_BOUND('',#7167,.T.);
#5124=FACE_OUTER_BOUND('',#7168,.T.);
#5125=FACE_OUTER_BOUND('',#7169,.T.);
#5126=FACE_OUTER_BOUND('',#7170,.T.);
#5127=FACE_OUTER_BOUND('',#7171,.T.);
#5128=FACE_OUTER_BOUND('',#7172,.T.);
#5129=FACE_OUTER_BOUND('',#7173,.T.);
#5130=FACE_OUTER_BOUND('',#7174,.T.);
#5131=FACE_OUTER_BOUND('',#7175,.T.);
#5132=FACE_OUTER_BOUND('',#7176,.T.);
#5133=FACE_OUTER_BOUND('',#7177,.T.);
#5134=FACE_OUTER_BOUND('',#7178,.T.);
#5135=FACE_OUTER_BOUND('',#7179,.T.);
#5136=FACE_OUTER_BOUND('',#7180,.T.);
#5137=FACE_OUTER_BOUND('',#7181,.T.);
#5138=FACE_OUTER_BOUND('',#7182,.T.);
#5139=FACE_OUTER_BOUND('',#7183,.T.);
#5140=FACE_OUTER_BOUND('',#7184,.T.);
#5141=FACE_OUTER_BOUND('',#7185,.T.);
#5142=FACE_OUTER_BOUND('',#7186,.T.);
#5143=FACE_OUTER_BOUND('',#7187,.T.);
#5144=FACE_OUTER_BOUND('',#7188,.T.);
#5145=FACE_OUTER_BOUND('',#7189,.T.);
#5146=FACE_OUTER_BOUND('',#7190,.T.);
#5147=FACE_OUTER_BOUND('',#7191,.T.);
#5148=FACE_OUTER_BOUND('',#7192,.T.);
#5149=FACE_OUTER_BOUND('',#7193,.T.);
#5150=FACE_OUTER_BOUND('',#7194,.T.);
#5151=FACE_OUTER_BOUND('',#7195,.T.);
#5152=FACE_OUTER_BOUND('',#7196,.T.);
#5153=FACE_OUTER_BOUND('',#7197,.T.);
#5154=FACE_OUTER_BOUND('',#7198,.T.);
#5155=FACE_OUTER_BOUND('',#7199,.T.);
#5156=FACE_OUTER_BOUND('',#7200,.T.);
#5157=FACE_OUTER_BOUND('',#7201,.T.);
#5158=FACE_OUTER_BOUND('',#7202,.T.);
#5159=FACE_OUTER_BOUND('',#7203,.T.);
#5160=FACE_OUTER_BOUND('',#7204,.T.);
#5161=FACE_OUTER_BOUND('',#7205,.T.);
#5162=FACE_OUTER_BOUND('',#7206,.T.);
#5163=FACE_OUTER_BOUND('',#7207,.T.);
#5164=FACE_OUTER_BOUND('',#7208,.T.);
#5165=FACE_OUTER_BOUND('',#7209,.T.);
#5166=FACE_OUTER_BOUND('',#7210,.T.);
#5167=FACE_OUTER_BOUND('',#7211,.T.);
#5168=FACE_OUTER_BOUND('',#7212,.T.);
#5169=FACE_OUTER_BOUND('',#7213,.T.);
#5170=FACE_OUTER_BOUND('',#7214,.T.);
#5171=FACE_OUTER_BOUND('',#7215,.T.);
#5172=FACE_OUTER_BOUND('',#7216,.T.);
#5173=FACE_OUTER_BOUND('',#7217,.T.);
#5174=FACE_OUTER_BOUND('',#7218,.T.);
#5175=FACE_OUTER_BOUND('',#7219,.T.);
#5176=FACE_OUTER_BOUND('',#7220,.T.);
#5177=FACE_OUTER_BOUND('',#7221,.T.);
#5178=FACE_OUTER_BOUND('',#7222,.T.);
#5179=FACE_OUTER_BOUND('',#7223,.T.);
#5180=FACE_OUTER_BOUND('',#7224,.T.);
#5181=FACE_OUTER_BOUND('',#7225,.T.);
#5182=FACE_OUTER_BOUND('',#7226,.T.);
#5183=FACE_OUTER_BOUND('',#7227,.T.);
#5184=FACE_OUTER_BOUND('',#7228,.T.);
#5185=FACE_OUTER_BOUND('',#7229,.T.);
#5186=FACE_OUTER_BOUND('',#7230,.T.);
#5187=FACE_OUTER_BOUND('',#7231,.T.);
#5188=FACE_OUTER_BOUND('',#7232,.T.);
#5189=FACE_OUTER_BOUND('',#7233,.T.);
#5190=FACE_OUTER_BOUND('',#7234,.T.);
#5191=FACE_OUTER_BOUND('',#7235,.T.);
#5192=FACE_OUTER_BOUND('',#7236,.T.);
#5193=FACE_OUTER_BOUND('',#7237,.T.);
#5194=FACE_OUTER_BOUND('',#7238,.T.);
#5195=FACE_OUTER_BOUND('',#7239,.T.);
#5196=FACE_OUTER_BOUND('',#7240,.T.);
#5197=FACE_OUTER_BOUND('',#7241,.T.);
#5198=FACE_OUTER_BOUND('',#7242,.T.);
#5199=FACE_OUTER_BOUND('',#7243,.T.);
#5200=FACE_OUTER_BOUND('',#7244,.T.);
#5201=FACE_OUTER_BOUND('',#7245,.T.);
#5202=FACE_OUTER_BOUND('',#7246,.T.);
#5203=FACE_OUTER_BOUND('',#7247,.T.);
#5204=FACE_OUTER_BOUND('',#7248,.T.);
#7088=EDGE_LOOP('',(#26453,#26454,#26455,#26456));
#7089=EDGE_LOOP('',(#26457,#26458,#26459,#26460));
#7090=EDGE_LOOP('',(#26461,#26462,#26463,#26464));
#7091=EDGE_LOOP('',(#26465,#26466,#26467,#26468));
#7092=EDGE_LOOP('',(#26469,#26470,#26471,#26472));
#7093=EDGE_LOOP('',(#26473,#26474,#26475,#26476));
#7094=EDGE_LOOP('',(#26477,#26478,#26479,#26480));
#7095=EDGE_LOOP('',(#26481,#26482,#26483,#26484));
#7096=EDGE_LOOP('',(#26485,#26486,#26487,#26488));
#7097=EDGE_LOOP('',(#26489,#26490,#26491,#26492));
#7098=EDGE_LOOP('',(#26493,#26494,#26495,#26496));
#7099=EDGE_LOOP('',(#26497,#26498,#26499,#26500));
#7100=EDGE_LOOP('',(#26501,#26502,#26503,#26504));
#7101=EDGE_LOOP('',(#26505,#26506,#26507,#26508));
#7102=EDGE_LOOP('',(#26509,#26510,#26511,#26512));
#7103=EDGE_LOOP('',(#26513,#26514,#26515,#26516));
#7104=EDGE_LOOP('',(#26517,#26518,#26519,#26520));
#7105=EDGE_LOOP('',(#26521,#26522,#26523,#26524));
#7106=EDGE_LOOP('',(#26525,#26526,#26527,#26528));
#7107=EDGE_LOOP('',(#26529,#26530,#26531,#26532));
#7108=EDGE_LOOP('',(#26533,#26534,#26535,#26536));
#7109=EDGE_LOOP('',(#26537,#26538,#26539,#26540));
#7110=EDGE_LOOP('',(#26541,#26542,#26543,#26544));
#7111=EDGE_LOOP('',(#26545,#26546,#26547,#26548));
#7112=EDGE_LOOP('',(#26549,#26550,#26551,#26552));
#7113=EDGE_LOOP('',(#26553,#26554,#26555,#26556));
#7114=EDGE_LOOP('',(#26557,#26558,#26559,#26560));
#7115=EDGE_LOOP('',(#26561,#26562,#26563,#26564));
#7116=EDGE_LOOP('',(#26565,#26566,#26567,#26568));
#7117=EDGE_LOOP('',(#26569,#26570,#26571,#26572));
#7118=EDGE_LOOP('',(#26573,#26574,#26575,#26576));
#7119=EDGE_LOOP('',(#26577,#26578,#26579,#26580));
#7120=EDGE_LOOP('',(#26581,#26582,#26583,#26584));
#7121=EDGE_LOOP('',(#26585,#26586,#26587,#26588));
#7122=EDGE_LOOP('',(#26589,#26590,#26591,#26592));
#7123=EDGE_LOOP('',(#26593,#26594,#26595,#26596));
#7124=EDGE_LOOP('',(#26597,#26598,#26599,#26600));
#7125=EDGE_LOOP('',(#26601,#26602,#26603,#26604));
#7126=EDGE_LOOP('',(#26605,#26606,#26607,#26608));
#7127=EDGE_LOOP('',(#26609,#26610,#26611,#26612));
#7128=EDGE_LOOP('',(#26613,#26614,#26615,#26616));
#7129=EDGE_LOOP('',(#26617,#26618,#26619,#26620));
#7130=EDGE_LOOP('',(#26621,#26622,#26623,#26624));
#7131=EDGE_LOOP('',(#26625,#26626,#26627,#26628));
#7132=EDGE_LOOP('',(#26629,#26630,#26631,#26632));
#7133=EDGE_LOOP('',(#26633,#26634,#26635,#26636));
#7134=EDGE_LOOP('',(#26637,#26638,#26639,#26640));
#7135=EDGE_LOOP('',(#26641,#26642,#26643,#26644));
#7136=EDGE_LOOP('',(#26645,#26646,#26647,#26648));
#7137=EDGE_LOOP('',(#26649,#26650,#26651,#26652));
#7138=EDGE_LOOP('',(#26653,#26654,#26655,#26656));
#7139=EDGE_LOOP('',(#26657,#26658,#26659,#26660));
#7140=EDGE_LOOP('',(#26661,#26662,#26663,#26664));
#7141=EDGE_LOOP('',(#26665,#26666,#26667,#26668));
#7142=EDGE_LOOP('',(#26669,#26670,#26671,#26672));
#7143=EDGE_LOOP('',(#26673,#26674,#26675,#26676));
#7144=EDGE_LOOP('',(#26677,#26678,#26679,#26680));
#7145=EDGE_LOOP('',(#26681,#26682,#26683,#26684));
#7146=EDGE_LOOP('',(#26685,#26686,#26687,#26688));
#7147=EDGE_LOOP('',(#26689,#26690,#26691,#26692));
#7148=EDGE_LOOP('',(#26693,#26694,#26695,#26696));
#7149=EDGE_LOOP('',(#26697,#26698,#26699,#26700));
#7150=EDGE_LOOP('',(#26701,#26702,#26703,#26704));
#7151=EDGE_LOOP('',(#26705,#26706,#26707,#26708));
#7152=EDGE_LOOP('',(#26709,#26710,#26711,#26712));
#7153=EDGE_LOOP('',(#26713,#26714,#26715,#26716));
#7154=EDGE_LOOP('',(#26717,#26718,#26719,#26720));
#7155=EDGE_LOOP('',(#26721,#26722,#26723,#26724));
#7156=EDGE_LOOP('',(#26725,#26726,#26727,#26728));
#7157=EDGE_LOOP('',(#26729,#26730,#26731,#26732));
#7158=EDGE_LOOP('',(#26733,#26734,#26735,#26736));
#7159=EDGE_LOOP('',(#26737,#26738,#26739,#26740));
#7160=EDGE_LOOP('',(#26741,#26742,#26743,#26744));
#7161=EDGE_LOOP('',(#26745,#26746,#26747,#26748));
#7162=EDGE_LOOP('',(#26749,#26750,#26751,#26752));
#7163=EDGE_LOOP('',(#26753,#26754,#26755,#26756));
#7164=EDGE_LOOP('',(#26757,#26758,#26759,#26760));
#7165=EDGE_LOOP('',(#26761,#26762,#26763,#26764));
#7166=EDGE_LOOP('',(#26765,#26766,#26767,#26768));
#7167=EDGE_LOOP('',(#26769,#26770,#26771,#26772));
#7168=EDGE_LOOP('',(#26773,#26774,#26775,#26776));
#7169=EDGE_LOOP('',(#26777,#26778,#26779,#26780));
#7170=EDGE_LOOP('',(#26781,#26782,#26783,#26784));
#7171=EDGE_LOOP('',(#26785,#26786,#26787,#26788));
#7172=EDGE_LOOP('',(#26789,#26790,#26791,#26792));
#7173=EDGE_LOOP('',(#26793,#26794,#26795,#26796));
#7174=EDGE_LOOP('',(#26797,#26798,#26799,#26800));
#7175=EDGE_LOOP('',(#26801,#26802,#26803,#26804));
#7176=EDGE_LOOP('',(#26805,#26806,#26807,#26808));
#7177=EDGE_LOOP('',(#26809,#26810,#26811,#26812));
#7178=EDGE_LOOP('',(#26813,#26814,#26815,#26816));
#7179=EDGE_LOOP('',(#26817,#26818,#26819,#26820));
#7180=EDGE_LOOP('',(#26821,#26822,#26823,#26824));
#7181=EDGE_LOOP('',(#26825,#26826,#26827,#26828));
#7182=EDGE_LOOP('',(#26829,#26830,#26831,#26832));
#7183=EDGE_LOOP('',(#26833,#26834,#26835,#26836));
#7184=EDGE_LOOP('',(#26837,#26838,#26839,#26840));
#7185=EDGE_LOOP('',(#26841,#26842,#26843,#26844));
#7186=EDGE_LOOP('',(#26845,#26846,#26847,#26848));
#7187=EDGE_LOOP('',(#26849,#26850,#26851,#26852));
#7188=EDGE_LOOP('',(#26853,#26854,#26855,#26856));
#7189=EDGE_LOOP('',(#26857,#26858,#26859,#26860));
#7190=EDGE_LOOP('',(#26861,#26862,#26863,#26864));
#7191=EDGE_LOOP('',(#26865,#26866,#26867,#26868));
#7192=EDGE_LOOP('',(#26869,#26870,#26871,#26872));
#7193=EDGE_LOOP('',(#26873,#26874,#26875,#26876));
#7194=EDGE_LOOP('',(#26877,#26878,#26879,#26880));
#7195=EDGE_LOOP('',(#26881,#26882,#26883,#26884));
#7196=EDGE_LOOP('',(#26885,#26886,#26887,#26888));
#7197=EDGE_LOOP('',(#26889,#26890,#26891,#26892));
#7198=EDGE_LOOP('',(#26893,#26894,#26895,#26896));
#7199=EDGE_LOOP('',(#26897,#26898,#26899,#26900));
#7200=EDGE_LOOP('',(#26901,#26902,#26903,#26904));
#7201=EDGE_LOOP('',(#26905,#26906,#26907,#26908));
#7202=EDGE_LOOP('',(#26909,#26910,#26911,#26912));
#7203=EDGE_LOOP('',(#26913,#26914,#26915,#26916));
#7204=EDGE_LOOP('',(#26917,#26918,#26919,#26920));
#7205=EDGE_LOOP('',(#26921,#26922,#26923,#26924));
#7206=EDGE_LOOP('',(#26925,#26926,#26927,#26928));
#7207=EDGE_LOOP('',(#26929,#26930,#26931,#26932));
#7208=EDGE_LOOP('',(#26933,#26934,#26935,#26936));
#7209=EDGE_LOOP('',(#26937,#26938,#26939,#26940));
#7210=EDGE_LOOP('',(#26941,#26942,#26943,#26944));
#7211=EDGE_LOOP('',(#26945,#26946,#26947,#26948));
#7212=EDGE_LOOP('',(#26949,#26950,#26951,#26952));
#7213=EDGE_LOOP('',(#26953,#26954,#26955,#26956));
#7214=EDGE_LOOP('',(#26957,#26958,#26959,#26960));
#7215=EDGE_LOOP('',(#26961,#26962,#26963,#26964));
#7216=EDGE_LOOP('',(#26965,#26966,#26967,#26968));
#7217=EDGE_LOOP('',(#26969,#26970,#26971,#26972));
#7218=EDGE_LOOP('',(#26973,#26974,#26975,#26976));
#7219=EDGE_LOOP('',(#26977,#26978,#26979,#26980));
#7220=EDGE_LOOP('',(#26981,#26982,#26983,#26984));
#7221=EDGE_LOOP('',(#26985,#26986,#26987,#26988));
#7222=EDGE_LOOP('',(#26989,#26990,#26991,#26992));
#7223=EDGE_LOOP('',(#26993,#26994,#26995,#26996));
#7224=EDGE_LOOP('',(#26997,#26998,#26999,#27000));
#7225=EDGE_LOOP('',(#27001,#27002,#27003,#27004));
#7226=EDGE_LOOP('',(#27005,#27006,#27007,#27008));
#7227=EDGE_LOOP('',(#27009,#27010,#27011,#27012));
#7228=EDGE_LOOP('',(#27013,#27014,#27015,#27016));
#7229=EDGE_LOOP('',(#27017,#27018,#27019,#27020));
#7230=EDGE_LOOP('',(#27021,#27022,#27023,#27024));
#7231=EDGE_LOOP('',(#27025,#27026,#27027,#27028));
#7232=EDGE_LOOP('',(#27029,#27030,#27031,#27032));
#7233=EDGE_LOOP('',(#27033,#27034,#27035,#27036));
#7234=EDGE_LOOP('',(#27037,#27038,#27039,#27040));
#7235=EDGE_LOOP('',(#27041,#27042,#27043,#27044));
#7236=EDGE_LOOP('',(#27045,#27046,#27047,#27048));
#7237=EDGE_LOOP('',(#27049,#27050,#27051,#27052));
#7238=EDGE_LOOP('',(#27053,#27054,#27055,#27056,#27057));
#7239=EDGE_LOOP('',(#27058,#27059,#27060,#27061,#27062,#27063,#27064,#27065,
#27066,#27067,#27068,#27069,#27070,#27071,#27072,#27073,#27074,#27075,#27076,
#27077,#27078,#27079,#27080,#27081,#27082,#27083,#27084,#27085,#27086,#27087,
#27088,#27089,#27090,#27091,#27092,#27093,#27094,#27095,#27096,#27097,#27098,
#27099,#27100,#27101,#27102,#27103,#27104,#27105,#27106,#27107,#27108,#27109,
#27110,#27111,#27112,#27113,#27114,#27115,#27116,#27117,#27118,#27119,#27120,
#27121,#27122,#27123,#27124,#27125,#27126,#27127,#27128,#27129,#27130,#27131,
#27132,#27133,#27134,#27135,#27136,#27137,#27138,#27139,#27140,#27141,#27142,
#27143,#27144,#27145,#27146,#27147,#27148,#27149,#27150,#27151,#27152,#27153,
#27154,#27155,#27156,#27157,#27158,#27159,#27160,#27161,#27162,#27163,#27164,
#27165,#27166,#27167,#27168,#27169,#27170,#27171,#27172,#27173,#27174,#27175,
#27176,#27177,#27178,#27179,#27180,#27181,#27182,#27183,#27184,#27185,#27186,
#27187,#27188,#27189,#27190,#27191,#27192,#27193,#27194,#27195,#27196,#27197,
#27198,#27199,#27200,#27201,#27202,#27203,#27204,#27205,#27206,#27207,#27208,
#27209,#27210,#27211));
#7240=EDGE_LOOP('',(#27212,#27213,#27214,#27215,#27216));
#7241=EDGE_LOOP('',(#27217,#27218,#27219,#27220));
#7242=EDGE_LOOP('',(#27221,#27222,#27223,#27224,#27225,#27226,#27227,#27228,
#27229,#27230,#27231,#27232,#27233,#27234,#27235,#27236,#27237,#27238,#27239,
#27240,#27241,#27242,#27243,#27244,#27245,#27246,#27247,#27248,#27249,#27250,
#27251,#27252,#27253,#27254,#27255,#27256,#27257,#27258,#27259,#27260,#27261,
#27262,#27263,#27264,#27265,#27266,#27267,#27268,#27269,#27270,#27271,#27272,
#27273,#27274,#27275,#27276,#27277,#27278,#27279,#27280,#27281,#27282,#27283,
#27284,#27285,#27286,#27287,#27288,#27289,#27290,#27291,#27292,#27293,#27294,
#27295,#27296,#27297,#27298,#27299,#27300,#27301,#27302,#27303,#27304,#27305,
#27306,#27307,#27308,#27309,#27310,#27311,#27312,#27313,#27314,#27315,#27316,
#27317,#27318,#27319,#27320,#27321,#27322,#27323,#27324,#27325,#27326,#27327,
#27328,#27329,#27330,#27331,#27332,#27333,#27334,#27335,#27336,#27337,#27338,
#27339,#27340,#27341,#27342,#27343,#27344,#27345,#27346,#27347,#27348,#27349,
#27350,#27351,#27352,#27353,#27354,#27355,#27356,#27357,#27358,#27359,#27360,
#27361,#27362,#27363,#27364,#27365,#27366,#27367,#27368,#27369,#27370,#27371,
#27372,#27373,#27374));
#7243=EDGE_LOOP('',(#27375,#27376,#27377,#27378));
#7244=EDGE_LOOP('',(#27379,#27380,#27381,#27382,#27383,#27384));
#7245=EDGE_LOOP('',(#27385,#27386,#27387,#27388));
#7246=EDGE_LOOP('',(#27389,#27390,#27391,#27392,#27393,#27394));
#7247=EDGE_LOOP('',(#27395));
#7248=EDGE_LOOP('',(#27396,#27397));
#7249=EDGE_LOOP('',(#27398));
#9376=LINE('',#70395,#11682);
#9377=LINE('',#70422,#11683);
#9378=LINE('',#70470,#11684);
#9379=LINE('',#70518,#11685);
#9380=LINE('',#70566,#11686);
#9381=LINE('',#70620,#11687);
#9382=LINE('',#70668,#11688);
#9383=LINE('',#70716,#11689);
#9384=LINE('',#70770,#11690);
#9385=LINE('',#70818,#11691);
#9386=LINE('',#70866,#11692);
#9387=LINE('',#70917,#11693);
#9388=LINE('',#70968,#11694);
#9389=LINE('',#71016,#11695);
#9390=LINE('',#71064,#11696);
#9391=LINE('',#71118,#11697);
#9392=LINE('',#71166,#11698);
#9393=LINE('',#71214,#11699);
#9394=LINE('',#71265,#11700);
#9395=LINE('',#71313,#11701);
#9396=LINE('',#71361,#11702);
#9397=LINE('',#71409,#11703);
#9398=LINE('',#71463,#11704);
#9399=LINE('',#71511,#11705);
#9400=LINE('',#71559,#11706);
#9401=LINE('',#71613,#11707);
#9402=LINE('',#71661,#11708);
#9403=LINE('',#71709,#11709);
#9404=LINE('',#71757,#11710);
#9405=LINE('',#71811,#11711);
#9406=LINE('',#71859,#11712);
#9407=LINE('',#71907,#11713);
#9408=LINE('',#71961,#11714);
#9409=LINE('',#72009,#11715);
#9410=LINE('',#72057,#11716);
#9411=LINE('',#72105,#11717);
#9412=LINE('',#72159,#11718);
#9413=LINE('',#72207,#11719);
#9414=LINE('',#72255,#11720);
#9415=LINE('',#72309,#11721);
#9416=LINE('',#72357,#11722);
#9417=LINE('',#72405,#11723);
#9418=LINE('',#72453,#11724);
#9419=LINE('',#72507,#11725);
#9420=LINE('',#72555,#11726);
#9421=LINE('',#72603,#11727);
#9422=LINE('',#72657,#11728);
#9423=LINE('',#72705,#11729);
#9424=LINE('',#72753,#11730);
#9425=LINE('',#72801,#11731);
#9426=LINE('',#72855,#11732);
#9427=LINE('',#72903,#11733);
#9428=LINE('',#72951,#11734);
#9429=LINE('',#73005,#11735);
#9430=LINE('',#73053,#11736);
#9431=LINE('',#73101,#11737);
#9432=LINE('',#73149,#11738);
#9433=LINE('',#73203,#11739);
#9434=LINE('',#73251,#11740);
#9435=LINE('',#73299,#11741);
#9436=LINE('',#73353,#11742);
#9437=LINE('',#73401,#11743);
#9438=LINE('',#73449,#11744);
#9439=LINE('',#73500,#11745);
#9440=LINE('',#73551,#11746);
#9441=LINE('',#73599,#11747);
#9442=LINE('',#73647,#11748);
#9443=LINE('',#73701,#11749);
#9444=LINE('',#73749,#11750);
#9445=LINE('',#73797,#11751);
#9446=LINE('',#73848,#11752);
#9447=LINE('',#73896,#11753);
#9448=LINE('',#73944,#11754);
#9449=LINE('',#73992,#11755);
#9450=LINE('',#74046,#11756);
#9451=LINE('',#74094,#11757);
#9452=LINE('',#74110,#11758);
#9453=LINE('',#74135,#11759);
#9454=LINE('',#74160,#11760);
#9455=LINE('',#74185,#11761);
#9456=LINE('',#74209,#11762);
#9457=LINE('',#74233,#11763);
#9458=LINE('',#74258,#11764);
#9459=LINE('',#74283,#11765);
#9460=LINE('',#74307,#11766);
#9461=LINE('',#74332,#11767);
#9462=LINE('',#74357,#11768);
#9463=LINE('',#74381,#11769);
#9464=LINE('',#74406,#11770);
#9465=LINE('',#74430,#11771);
#9466=LINE('',#74455,#11772);
#9467=LINE('',#74479,#11773);
#9468=LINE('',#74504,#11774);
#9469=LINE('',#74529,#11775);
#9470=LINE('',#74553,#11776);
#9471=LINE('',#74578,#11777);
#9472=LINE('',#74603,#11778);
#9473=LINE('',#74627,#11779);
#9474=LINE('',#74651,#11780);
#9475=LINE('',#74676,#11781);
#9476=LINE('',#74701,#11782);
#9477=LINE('',#74725,#11783);
#9478=LINE('',#74750,#11784);
#9479=LINE('',#74775,#11785);
#9480=LINE('',#74799,#11786);
#9481=LINE('',#74823,#11787);
#9482=LINE('',#74848,#11788);
#9483=LINE('',#74873,#11789);
#9484=LINE('',#74897,#11790);
#9485=LINE('',#74922,#11791);
#9486=LINE('',#74947,#11792);
#9487=LINE('',#74971,#11793);
#9488=LINE('',#74995,#11794);
#9489=LINE('',#75020,#11795);
#9490=LINE('',#75045,#11796);
#9491=LINE('',#75069,#11797);
#9492=LINE('',#75094,#11798);
#9493=LINE('',#75119,#11799);
#9494=LINE('',#75143,#11800);
#9495=LINE('',#75167,#11801);
#9496=LINE('',#75192,#11802);
#9497=LINE('',#75217,#11803);
#9498=LINE('',#75241,#11804);
#9499=LINE('',#75266,#11805);
#9500=LINE('',#75291,#11806);
#9501=LINE('',#75315,#11807);
#9502=LINE('',#75339,#11808);
#9503=LINE('',#75364,#11809);
#9504=LINE('',#75389,#11810);
#9505=LINE('',#75413,#11811);
#9506=LINE('',#75438,#11812);
#9507=LINE('',#75463,#11813);
#9508=LINE('',#75487,#11814);
#9509=LINE('',#75511,#11815);
#9510=LINE('',#75536,#11816);
#9511=LINE('',#75561,#11817);
#9512=LINE('',#75585,#11818);
#9513=LINE('',#75610,#11819);
#9514=LINE('',#75635,#11820);
#9515=LINE('',#75659,#11821);
#9516=LINE('',#75684,#11822);
#9517=LINE('',#75708,#11823);
#9518=LINE('',#75733,#11824);
#9519=LINE('',#75757,#11825);
#9520=LINE('',#75782,#11826);
#9521=LINE('',#75807,#11827);
#9522=LINE('',#75831,#11828);
#9523=LINE('',#75856,#11829);
#9524=LINE('',#75881,#11830);
#9525=LINE('',#75905,#11831);
#9526=LINE('',#80248,#11832);
#9527=LINE('',#80251,#11833);
#9528=LINE('',#80257,#11834);
#11682=VECTOR('',#39595,5.);
#11683=VECTOR('',#39600,5.);
#11684=VECTOR('',#39603,5.);
#11685=VECTOR('',#39606,5.);
#11686=VECTOR('',#39609,5.);
#11687=VECTOR('',#39612,5.);
#11688=VECTOR('',#39615,5.);
#11689=VECTOR('',#39618,5.);
#11690=VECTOR('',#39621,5.);
#11691=VECTOR('',#39624,5.);
#11692=VECTOR('',#39627,5.);
#11693=VECTOR('',#39630,5.);
#11694=VECTOR('',#39633,5.);
#11695=VECTOR('',#39636,5.);
#11696=VECTOR('',#39639,5.);
#11697=VECTOR('',#39642,5.);
#11698=VECTOR('',#39645,5.);
#11699=VECTOR('',#39648,5.);
#11700=VECTOR('',#39651,5.);
#11701=VECTOR('',#39654,5.);
#11702=VECTOR('',#39657,5.);
#11703=VECTOR('',#39660,5.);
#11704=VECTOR('',#39663,5.);
#11705=VECTOR('',#39666,5.);
#11706=VECTOR('',#39669,5.);
#11707=VECTOR('',#39672,5.);
#11708=VECTOR('',#39675,5.);
#11709=VECTOR('',#39678,5.);
#11710=VECTOR('',#39681,5.);
#11711=VECTOR('',#39684,5.);
#11712=VECTOR('',#39687,5.);
#11713=VECTOR('',#39690,5.);
#11714=VECTOR('',#39693,5.);
#11715=VECTOR('',#39696,5.);
#11716=VECTOR('',#39699,5.);
#11717=VECTOR('',#39702,5.);
#11718=VECTOR('',#39705,5.);
#11719=VECTOR('',#39708,5.);
#11720=VECTOR('',#39711,5.);
#11721=VECTOR('',#39714,5.);
#11722=VECTOR('',#39717,5.);
#11723=VECTOR('',#39720,5.);
#11724=VECTOR('',#39723,5.);
#11725=VECTOR('',#39726,5.);
#11726=VECTOR('',#39729,5.);
#11727=VECTOR('',#39732,5.);
#11728=VECTOR('',#39735,5.);
#11729=VECTOR('',#39738,5.);
#11730=VECTOR('',#39741,5.);
#11731=VECTOR('',#39744,5.);
#11732=VECTOR('',#39747,5.);
#11733=VECTOR('',#39750,5.);
#11734=VECTOR('',#39753,5.);
#11735=VECTOR('',#39756,5.);
#11736=VECTOR('',#39759,5.);
#11737=VECTOR('',#39762,5.);
#11738=VECTOR('',#39765,5.);
#11739=VECTOR('',#39768,5.);
#11740=VECTOR('',#39771,5.);
#11741=VECTOR('',#39774,5.);
#11742=VECTOR('',#39777,5.);
#11743=VECTOR('',#39780,5.);
#11744=VECTOR('',#39783,5.);
#11745=VECTOR('',#39786,5.);
#11746=VECTOR('',#39789,5.);
#11747=VECTOR('',#39792,5.);
#11748=VECTOR('',#39795,5.);
#11749=VECTOR('',#39798,5.);
#11750=VECTOR('',#39801,5.);
#11751=VECTOR('',#39804,5.);
#11752=VECTOR('',#39807,5.);
#11753=VECTOR('',#39810,5.);
#11754=VECTOR('',#39813,5.);
#11755=VECTOR('',#39816,5.);
#11756=VECTOR('',#39819,5.);
#11757=VECTOR('',#39822,4.52375);
#11758=VECTOR('',#39827,4.52375);
#11759=VECTOR('',#39830,4.52375);
#11760=VECTOR('',#39833,4.52375);
#11761=VECTOR('',#39836,4.52375);
#11762=VECTOR('',#39839,4.52375);
#11763=VECTOR('',#39842,4.52375);
#11764=VECTOR('',#39845,4.52375);
#11765=VECTOR('',#39848,4.52375);
#11766=VECTOR('',#39851,4.52375);
#11767=VECTOR('',#39854,4.52375);
#11768=VECTOR('',#39857,4.52375);
#11769=VECTOR('',#39860,4.52375);
#11770=VECTOR('',#39863,4.52375);
#11771=VECTOR('',#39866,4.52375);
#11772=VECTOR('',#39869,4.52375);
#11773=VECTOR('',#39872,4.52375);
#11774=VECTOR('',#39875,4.52375);
#11775=VECTOR('',#39878,4.52375);
#11776=VECTOR('',#39881,4.52375);
#11777=VECTOR('',#39884,4.52375);
#11778=VECTOR('',#39887,4.52375);
#11779=VECTOR('',#39890,4.52375);
#11780=VECTOR('',#39893,4.52375);
#11781=VECTOR('',#39896,4.52375);
#11782=VECTOR('',#39899,4.52375);
#11783=VECTOR('',#39902,4.52375);
#11784=VECTOR('',#39905,4.52375);
#11785=VECTOR('',#39908,4.52375);
#11786=VECTOR('',#39911,4.52375);
#11787=VECTOR('',#39914,4.52375);
#11788=VECTOR('',#39917,4.52375);
#11789=VECTOR('',#39920,4.52375);
#11790=VECTOR('',#39923,4.52375);
#11791=VECTOR('',#39926,4.52375);
#11792=VECTOR('',#39929,4.52375);
#11793=VECTOR('',#39932,4.52375);
#11794=VECTOR('',#39935,4.52375);
#11795=VECTOR('',#39938,4.52375);
#11796=VECTOR('',#39941,4.52375);
#11797=VECTOR('',#39944,4.52375);
#11798=VECTOR('',#39947,4.52375);
#11799=VECTOR('',#39950,4.52375);
#11800=VECTOR('',#39953,4.52375);
#11801=VECTOR('',#39956,4.52375);
#11802=VECTOR('',#39959,4.52375);
#11803=VECTOR('',#39962,4.52375);
#11804=VECTOR('',#39965,4.52375);
#11805=VECTOR('',#39968,4.52375);
#11806=VECTOR('',#39971,4.52375);
#11807=VECTOR('',#39974,4.52375);
#11808=VECTOR('',#39977,4.52375);
#11809=VECTOR('',#39980,4.52375);
#11810=VECTOR('',#39983,4.52375);
#11811=VECTOR('',#39986,4.52375);
#11812=VECTOR('',#39989,4.52375);
#11813=VECTOR('',#39992,4.52375);
#11814=VECTOR('',#39995,4.52375);
#11815=VECTOR('',#39998,4.52375);
#11816=VECTOR('',#40001,4.52375);
#11817=VECTOR('',#40004,4.52375);
#11818=VECTOR('',#40007,4.52375);
#11819=VECTOR('',#40010,4.52375);
#11820=VECTOR('',#40013,4.52375);
#11821=VECTOR('',#40016,4.52375);
#11822=VECTOR('',#40019,4.52375);
#11823=VECTOR('',#40022,4.52375);
#11824=VECTOR('',#40025,4.52375);
#11825=VECTOR('',#40028,4.52375);
#11826=VECTOR('',#40031,4.52375);
#11827=VECTOR('',#40034,4.52375);
#11828=VECTOR('',#40037,4.52375);
#11829=VECTOR('',#40040,4.52375);
#11830=VECTOR('',#40043,4.52375);
#11831=VECTOR('',#40046,4.52375);
#11832=VECTOR('',#40067,2.5);
#11833=VECTOR('',#40072,3.75);
#11834=VECTOR('',#40081,4.75);
#14313=VERTEX_POINT('',#70393);
#14314=VERTEX_POINT('',#70394);
#14315=VERTEX_POINT('',#70396);
#14316=VERTEX_POINT('',#70407);
#14317=VERTEX_POINT('',#70420);
#14318=VERTEX_POINT('',#70421);
#14319=VERTEX_POINT('',#70468);
#14320=VERTEX_POINT('',#70469);
#14321=VERTEX_POINT('',#70516);
#14322=VERTEX_POINT('',#70517);
#14323=VERTEX_POINT('',#70564);
#14324=VERTEX_POINT('',#70565);
#14325=VERTEX_POINT('',#70618);
#14326=VERTEX_POINT('',#70619);
#14327=VERTEX_POINT('',#70666);
#14328=VERTEX_POINT('',#70667);
#14329=VERTEX_POINT('',#70714);
#14330=VERTEX_POINT('',#70715);
#14331=VERTEX_POINT('',#70768);
#14332=VERTEX_POINT('',#70769);
#14333=VERTEX_POINT('',#70816);
#14334=VERTEX_POINT('',#70817);
#14335=VERTEX_POINT('',#70864);
#14336=VERTEX_POINT('',#70865);
#14337=VERTEX_POINT('',#70915);
#14338=VERTEX_POINT('',#70916);
#14339=VERTEX_POINT('',#70966);
#14340=VERTEX_POINT('',#70967);
#14341=VERTEX_POINT('',#71014);
#14342=VERTEX_POINT('',#71015);
#14343=VERTEX_POINT('',#71062);
#14344=VERTEX_POINT('',#71063);
#14345=VERTEX_POINT('',#71116);
#14346=VERTEX_POINT('',#71117);
#14347=VERTEX_POINT('',#71164);
#14348=VERTEX_POINT('',#71165);
#14349=VERTEX_POINT('',#71212);
#14350=VERTEX_POINT('',#71213);
#14351=VERTEX_POINT('',#71263);
#14352=VERTEX_POINT('',#71264);
#14353=VERTEX_POINT('',#71311);
#14354=VERTEX_POINT('',#71312);
#14355=VERTEX_POINT('',#71359);
#14356=VERTEX_POINT('',#71360);
#14357=VERTEX_POINT('',#71407);
#14358=VERTEX_POINT('',#71408);
#14359=VERTEX_POINT('',#71461);
#14360=VERTEX_POINT('',#71462);
#14361=VERTEX_POINT('',#71509);
#14362=VERTEX_POINT('',#71510);
#14363=VERTEX_POINT('',#71557);
#14364=VERTEX_POINT('',#71558);
#14365=VERTEX_POINT('',#71611);
#14366=VERTEX_POINT('',#71612);
#14367=VERTEX_POINT('',#71659);
#14368=VERTEX_POINT('',#71660);
#14369=VERTEX_POINT('',#71707);
#14370=VERTEX_POINT('',#71708);
#14371=VERTEX_POINT('',#71755);
#14372=VERTEX_POINT('',#71756);
#14373=VERTEX_POINT('',#71809);
#14374=VERTEX_POINT('',#71810);
#14375=VERTEX_POINT('',#71857);
#14376=VERTEX_POINT('',#71858);
#14377=VERTEX_POINT('',#71905);
#14378=VERTEX_POINT('',#71906);
#14379=VERTEX_POINT('',#71959);
#14380=VERTEX_POINT('',#71960);
#14381=VERTEX_POINT('',#72007);
#14382=VERTEX_POINT('',#72008);
#14383=VERTEX_POINT('',#72055);
#14384=VERTEX_POINT('',#72056);
#14385=VERTEX_POINT('',#72103);
#14386=VERTEX_POINT('',#72104);
#14387=VERTEX_POINT('',#72157);
#14388=VERTEX_POINT('',#72158);
#14389=VERTEX_POINT('',#72205);
#14390=VERTEX_POINT('',#72206);
#14391=VERTEX_POINT('',#72253);
#14392=VERTEX_POINT('',#72254);
#14393=VERTEX_POINT('',#72307);
#14394=VERTEX_POINT('',#72308);
#14395=VERTEX_POINT('',#72355);
#14396=VERTEX_POINT('',#72356);
#14397=VERTEX_POINT('',#72403);
#14398=VERTEX_POINT('',#72404);
#14399=VERTEX_POINT('',#72451);
#14400=VERTEX_POINT('',#72452);
#14401=VERTEX_POINT('',#72505);
#14402=VERTEX_POINT('',#72506);
#14403=VERTEX_POINT('',#72553);
#14404=VERTEX_POINT('',#72554);
#14405=VERTEX_POINT('',#72601);
#14406=VERTEX_POINT('',#72602);
#14407=VERTEX_POINT('',#72655);
#14408=VERTEX_POINT('',#72656);
#14409=VERTEX_POINT('',#72703);
#14410=VERTEX_POINT('',#72704);
#14411=VERTEX_POINT('',#72751);
#14412=VERTEX_POINT('',#72752);
#14413=VERTEX_POINT('',#72799);
#14414=VERTEX_POINT('',#72800);
#14415=VERTEX_POINT('',#72853);
#14416=VERTEX_POINT('',#72854);
#14417=VERTEX_POINT('',#72901);
#14418=VERTEX_POINT('',#72902);
#14419=VERTEX_POINT('',#72949);
#14420=VERTEX_POINT('',#72950);
#14421=VERTEX_POINT('',#73003);
#14422=VERTEX_POINT('',#73004);
#14423=VERTEX_POINT('',#73051);
#14424=VERTEX_POINT('',#73052);
#14425=VERTEX_POINT('',#73099);
#14426=VERTEX_POINT('',#73100);
#14427=VERTEX_POINT('',#73147);
#14428=VERTEX_POINT('',#73148);
#14429=VERTEX_POINT('',#73201);
#14430=VERTEX_POINT('',#73202);
#14431=VERTEX_POINT('',#73249);
#14432=VERTEX_POINT('',#73250);
#14433=VERTEX_POINT('',#73297);
#14434=VERTEX_POINT('',#73298);
#14435=VERTEX_POINT('',#73351);
#14436=VERTEX_POINT('',#73352);
#14437=VERTEX_POINT('',#73399);
#14438=VERTEX_POINT('',#73400);
#14439=VERTEX_POINT('',#73447);
#14440=VERTEX_POINT('',#73448);
#14441=VERTEX_POINT('',#73498);
#14442=VERTEX_POINT('',#73499);
#14443=VERTEX_POINT('',#73549);
#14444=VERTEX_POINT('',#73550);
#14445=VERTEX_POINT('',#73597);
#14446=VERTEX_POINT('',#73598);
#14447=VERTEX_POINT('',#73645);
#14448=VERTEX_POINT('',#73646);
#14449=VERTEX_POINT('',#73699);
#14450=VERTEX_POINT('',#73700);
#14451=VERTEX_POINT('',#73747);
#14452=VERTEX_POINT('',#73748);
#14453=VERTEX_POINT('',#73795);
#14454=VERTEX_POINT('',#73796);
#14455=VERTEX_POINT('',#73846);
#14456=VERTEX_POINT('',#73847);
#14457=VERTEX_POINT('',#73894);
#14458=VERTEX_POINT('',#73895);
#14459=VERTEX_POINT('',#73942);
#14460=VERTEX_POINT('',#73943);
#14461=VERTEX_POINT('',#73990);
#14462=VERTEX_POINT('',#73991);
#14463=VERTEX_POINT('',#74044);
#14464=VERTEX_POINT('',#74045);
#14465=VERTEX_POINT('',#74092);
#14466=VERTEX_POINT('',#74093);
#14467=VERTEX_POINT('',#74095);
#14468=VERTEX_POINT('',#74101);
#14469=VERTEX_POINT('',#74108);
#14470=VERTEX_POINT('',#74109);
#14471=VERTEX_POINT('',#74133);
#14472=VERTEX_POINT('',#74134);
#14473=VERTEX_POINT('',#74158);
#14474=VERTEX_POINT('',#74159);
#14475=VERTEX_POINT('',#74183);
#14476=VERTEX_POINT('',#74184);
#14477=VERTEX_POINT('',#74207);
#14478=VERTEX_POINT('',#74208);
#14479=VERTEX_POINT('',#74231);
#14480=VERTEX_POINT('',#74232);
#14481=VERTEX_POINT('',#74256);
#14482=VERTEX_POINT('',#74257);
#14483=VERTEX_POINT('',#74281);
#14484=VERTEX_POINT('',#74282);
#14485=VERTEX_POINT('',#74305);
#14486=VERTEX_POINT('',#74306);
#14487=VERTEX_POINT('',#74330);
#14488=VERTEX_POINT('',#74331);
#14489=VERTEX_POINT('',#74355);
#14490=VERTEX_POINT('',#74356);
#14491=VERTEX_POINT('',#74379);
#14492=VERTEX_POINT('',#74380);
#14493=VERTEX_POINT('',#74404);
#14494=VERTEX_POINT('',#74405);
#14495=VERTEX_POINT('',#74428);
#14496=VERTEX_POINT('',#74429);
#14497=VERTEX_POINT('',#74453);
#14498=VERTEX_POINT('',#74454);
#14499=VERTEX_POINT('',#74477);
#14500=VERTEX_POINT('',#74478);
#14501=VERTEX_POINT('',#74502);
#14502=VERTEX_POINT('',#74503);
#14503=VERTEX_POINT('',#74527);
#14504=VERTEX_POINT('',#74528);
#14505=VERTEX_POINT('',#74551);
#14506=VERTEX_POINT('',#74552);
#14507=VERTEX_POINT('',#74576);
#14508=VERTEX_POINT('',#74577);
#14509=VERTEX_POINT('',#74601);
#14510=VERTEX_POINT('',#74602);
#14511=VERTEX_POINT('',#74625);
#14512=VERTEX_POINT('',#74626);
#14513=VERTEX_POINT('',#74649);
#14514=VERTEX_POINT('',#74650);
#14515=VERTEX_POINT('',#74674);
#14516=VERTEX_POINT('',#74675);
#14517=VERTEX_POINT('',#74699);
#14518=VERTEX_POINT('',#74700);
#14519=VERTEX_POINT('',#74723);
#14520=VERTEX_POINT('',#74724);
#14521=VERTEX_POINT('',#74748);
#14522=VERTEX_POINT('',#74749);
#14523=VERTEX_POINT('',#74773);
#14524=VERTEX_POINT('',#74774);
#14525=VERTEX_POINT('',#74797);
#14526=VERTEX_POINT('',#74798);
#14527=VERTEX_POINT('',#74821);
#14528=VERTEX_POINT('',#74822);
#14529=VERTEX_POINT('',#74846);
#14530=VERTEX_POINT('',#74847);
#14531=VERTEX_POINT('',#74871);
#14532=VERTEX_POINT('',#74872);
#14533=VERTEX_POINT('',#74895);
#14534=VERTEX_POINT('',#74896);
#14535=VERTEX_POINT('',#74920);
#14536=VERTEX_POINT('',#74921);
#14537=VERTEX_POINT('',#74945);
#14538=VERTEX_POINT('',#74946);
#14539=VERTEX_POINT('',#74969);
#14540=VERTEX_POINT('',#74970);
#14541=VERTEX_POINT('',#74993);
#14542=VERTEX_POINT('',#74994);
#14543=VERTEX_POINT('',#75018);
#14544=VERTEX_POINT('',#75019);
#14545=VERTEX_POINT('',#75043);
#14546=VERTEX_POINT('',#75044);
#14547=VERTEX_POINT('',#75067);
#14548=VERTEX_POINT('',#75068);
#14549=VERTEX_POINT('',#75092);
#14550=VERTEX_POINT('',#75093);
#14551=VERTEX_POINT('',#75117);
#14552=VERTEX_POINT('',#75118);
#14553=VERTEX_POINT('',#75141);
#14554=VERTEX_POINT('',#75142);
#14555=VERTEX_POINT('',#75165);
#14556=VERTEX_POINT('',#75166);
#14557=VERTEX_POINT('',#75190);
#14558=VERTEX_POINT('',#75191);
#14559=VERTEX_POINT('',#75215);
#14560=VERTEX_POINT('',#75216);
#14561=VERTEX_POINT('',#75239);
#14562=VERTEX_POINT('',#75240);
#14563=VERTEX_POINT('',#75264);
#14564=VERTEX_POINT('',#75265);
#14565=VERTEX_POINT('',#75289);
#14566=VERTEX_POINT('',#75290);
#14567=VERTEX_POINT('',#75313);
#14568=VERTEX_POINT('',#75314);
#14569=VERTEX_POINT('',#75337);
#14570=VERTEX_POINT('',#75338);
#14571=VERTEX_POINT('',#75362);
#14572=VERTEX_POINT('',#75363);
#14573=VERTEX_POINT('',#75387);
#14574=VERTEX_POINT('',#75388);
#14575=VERTEX_POINT('',#75411);
#14576=VERTEX_POINT('',#75412);
#14577=VERTEX_POINT('',#75436);
#14578=VERTEX_POINT('',#75437);
#14579=VERTEX_POINT('',#75461);
#14580=VERTEX_POINT('',#75462);
#14581=VERTEX_POINT('',#75485);
#14582=VERTEX_POINT('',#75486);
#14583=VERTEX_POINT('',#75509);
#14584=VERTEX_POINT('',#75510);
#14585=VERTEX_POINT('',#75534);
#14586=VERTEX_POINT('',#75535);
#14587=VERTEX_POINT('',#75559);
#14588=VERTEX_POINT('',#75560);
#14589=VERTEX_POINT('',#75583);
#14590=VERTEX_POINT('',#75584);
#14591=VERTEX_POINT('',#75608);
#14592=VERTEX_POINT('',#75609);
#14593=VERTEX_POINT('',#75633);
#14594=VERTEX_POINT('',#75634);
#14595=VERTEX_POINT('',#75657);
#14596=VERTEX_POINT('',#75658);
#14597=VERTEX_POINT('',#75682);
#14598=VERTEX_POINT('',#75683);
#14599=VERTEX_POINT('',#75706);
#14600=VERTEX_POINT('',#75707);
#14601=VERTEX_POINT('',#75731);
#14602=VERTEX_POINT('',#75732);
#14603=VERTEX_POINT('',#75755);
#14604=VERTEX_POINT('',#75756);
#14605=VERTEX_POINT('',#75780);
#14606=VERTEX_POINT('',#75781);
#14607=VERTEX_POINT('',#75805);
#14608=VERTEX_POINT('',#75806);
#14609=VERTEX_POINT('',#75829);
#14610=VERTEX_POINT('',#75830);
#14611=VERTEX_POINT('',#75854);
#14612=VERTEX_POINT('',#75855);
#14613=VERTEX_POINT('',#75879);
#14614=VERTEX_POINT('',#75880);
#14615=VERTEX_POINT('',#75903);
#14616=VERTEX_POINT('',#75904);
#14617=VERTEX_POINT('',#75927);
#14618=VERTEX_POINT('',#76034);
#14619=VERTEX_POINT('',#76036);
#14620=VERTEX_POINT('',#78075);
#14621=VERTEX_POINT('',#78192);
#14622=VERTEX_POINT('',#78195);
#14623=VERTEX_POINT('',#80245);
#14624=VERTEX_POINT('',#80247);
#14625=VERTEX_POINT('',#80255);
#14626=VERTEX_POINT('',#80260);
#14627=VERTEX_POINT('',#80261);
#18448=EDGE_CURVE('',#14313,#14314,#9376,.T.);
#18449=EDGE_CURVE('',#14313,#14315,#2912,.T.);
#18450=EDGE_CURVE('',#14315,#14316,#1765,.T.);
#18451=EDGE_CURVE('',#14316,#14314,#2913,.T.);
#18452=EDGE_CURVE('',#14317,#14318,#9377,.T.);
#18453=EDGE_CURVE('',#14317,#14313,#2914,.T.);
#18454=EDGE_CURVE('',#14314,#14318,#2915,.T.);
#18455=EDGE_CURVE('',#14319,#14320,#9378,.T.);
#18456=EDGE_CURVE('',#14319,#14317,#2916,.T.);
#18457=EDGE_CURVE('',#14318,#14320,#2917,.T.);
#18458=EDGE_CURVE('',#14321,#14322,#9379,.T.);
#18459=EDGE_CURVE('',#14321,#14319,#2918,.T.);
#18460=EDGE_CURVE('',#14320,#14322,#2919,.T.);
#18461=EDGE_CURVE('',#14323,#14324,#9380,.T.);
#18462=EDGE_CURVE('',#14323,#14321,#2920,.T.);
#18463=EDGE_CURVE('',#14322,#14324,#2921,.T.);
#18464=EDGE_CURVE('',#14325,#14326,#9381,.T.);
#18465=EDGE_CURVE('',#14325,#14323,#2922,.T.);
#18466=EDGE_CURVE('',#14324,#14326,#2923,.T.);
#18467=EDGE_CURVE('',#14327,#14328,#9382,.T.);
#18468=EDGE_CURVE('',#14327,#14325,#2924,.T.);
#18469=EDGE_CURVE('',#14326,#14328,#2925,.T.);
#18470=EDGE_CURVE('',#14329,#14330,#9383,.T.);
#18471=EDGE_CURVE('',#14329,#14327,#2926,.T.);
#18472=EDGE_CURVE('',#14328,#14330,#2927,.T.);
#18473=EDGE_CURVE('',#14331,#14332,#9384,.T.);
#18474=EDGE_CURVE('',#14331,#14329,#2928,.T.);
#18475=EDGE_CURVE('',#14330,#14332,#2929,.T.);
#18476=EDGE_CURVE('',#14333,#14334,#9385,.T.);
#18477=EDGE_CURVE('',#14333,#14331,#2930,.T.);
#18478=EDGE_CURVE('',#14332,#14334,#2931,.T.);
#18479=EDGE_CURVE('',#14335,#14336,#9386,.T.);
#18480=EDGE_CURVE('',#14335,#14333,#2932,.T.);
#18481=EDGE_CURVE('',#14334,#14336,#2933,.T.);
#18482=EDGE_CURVE('',#14337,#14338,#9387,.T.);
#18483=EDGE_CURVE('',#14337,#14335,#2934,.T.);
#18484=EDGE_CURVE('',#14336,#14338,#2935,.T.);
#18485=EDGE_CURVE('',#14339,#14340,#9388,.T.);
#18486=EDGE_CURVE('',#14339,#14337,#2936,.T.);
#18487=EDGE_CURVE('',#14338,#14340,#2937,.T.);
#18488=EDGE_CURVE('',#14341,#14342,#9389,.T.);
#18489=EDGE_CURVE('',#14341,#14339,#2938,.T.);
#18490=EDGE_CURVE('',#14340,#14342,#2939,.T.);
#18491=EDGE_CURVE('',#14343,#14344,#9390,.T.);
#18492=EDGE_CURVE('',#14343,#14341,#2940,.T.);
#18493=EDGE_CURVE('',#14342,#14344,#2941,.T.);
#18494=EDGE_CURVE('',#14345,#14346,#9391,.T.);
#18495=EDGE_CURVE('',#14345,#14343,#2942,.T.);
#18496=EDGE_CURVE('',#14344,#14346,#2943,.T.);
#18497=EDGE_CURVE('',#14347,#14348,#9392,.T.);
#18498=EDGE_CURVE('',#14347,#14345,#2944,.T.);
#18499=EDGE_CURVE('',#14346,#14348,#2945,.T.);
#18500=EDGE_CURVE('',#14349,#14350,#9393,.T.);
#18501=EDGE_CURVE('',#14349,#14347,#2946,.T.);
#18502=EDGE_CURVE('',#14348,#14350,#2947,.T.);
#18503=EDGE_CURVE('',#14351,#14352,#9394,.T.);
#18504=EDGE_CURVE('',#14351,#14349,#2948,.T.);
#18505=EDGE_CURVE('',#14350,#14352,#2949,.T.);
#18506=EDGE_CURVE('',#14353,#14354,#9395,.T.);
#18507=EDGE_CURVE('',#14353,#14351,#2950,.T.);
#18508=EDGE_CURVE('',#14352,#14354,#2951,.T.);
#18509=EDGE_CURVE('',#14355,#14356,#9396,.T.);
#18510=EDGE_CURVE('',#14355,#14353,#2952,.T.);
#18511=EDGE_CURVE('',#14354,#14356,#2953,.T.);
#18512=EDGE_CURVE('',#14357,#14358,#9397,.T.);
#18513=EDGE_CURVE('',#14357,#14355,#2954,.T.);
#18514=EDGE_CURVE('',#14356,#14358,#2955,.T.);
#18515=EDGE_CURVE('',#14359,#14360,#9398,.T.);
#18516=EDGE_CURVE('',#14359,#14357,#2956,.T.);
#18517=EDGE_CURVE('',#14358,#14360,#2957,.T.);
#18518=EDGE_CURVE('',#14361,#14362,#9399,.T.);
#18519=EDGE_CURVE('',#14361,#14359,#2958,.T.);
#18520=EDGE_CURVE('',#14360,#14362,#2959,.T.);
#18521=EDGE_CURVE('',#14363,#14364,#9400,.T.);
#18522=EDGE_CURVE('',#14363,#14361,#2960,.T.);
#18523=EDGE_CURVE('',#14362,#14364,#2961,.T.);
#18524=EDGE_CURVE('',#14365,#14366,#9401,.T.);
#18525=EDGE_CURVE('',#14365,#14363,#2962,.T.);
#18526=EDGE_CURVE('',#14364,#14366,#2963,.T.);
#18527=EDGE_CURVE('',#14367,#14368,#9402,.T.);
#18528=EDGE_CURVE('',#14367,#14365,#2964,.T.);
#18529=EDGE_CURVE('',#14366,#14368,#2965,.T.);
#18530=EDGE_CURVE('',#14369,#14370,#9403,.T.);
#18531=EDGE_CURVE('',#14369,#14367,#2966,.T.);
#18532=EDGE_CURVE('',#14368,#14370,#2967,.T.);
#18533=EDGE_CURVE('',#14371,#14372,#9404,.T.);
#18534=EDGE_CURVE('',#14371,#14369,#2968,.T.);
#18535=EDGE_CURVE('',#14370,#14372,#2969,.T.);
#18536=EDGE_CURVE('',#14373,#14374,#9405,.T.);
#18537=EDGE_CURVE('',#14373,#14371,#2970,.T.);
#18538=EDGE_CURVE('',#14372,#14374,#2971,.T.);
#18539=EDGE_CURVE('',#14375,#14376,#9406,.T.);
#18540=EDGE_CURVE('',#14375,#14373,#2972,.T.);
#18541=EDGE_CURVE('',#14374,#14376,#2973,.T.);
#18542=EDGE_CURVE('',#14377,#14378,#9407,.T.);
#18543=EDGE_CURVE('',#14377,#14375,#2974,.T.);
#18544=EDGE_CURVE('',#14376,#14378,#2975,.T.);
#18545=EDGE_CURVE('',#14379,#14380,#9408,.T.);
#18546=EDGE_CURVE('',#14379,#14377,#2976,.T.);
#18547=EDGE_CURVE('',#14378,#14380,#2977,.T.);
#18548=EDGE_CURVE('',#14381,#14382,#9409,.T.);
#18549=EDGE_CURVE('',#14381,#14379,#2978,.T.);
#18550=EDGE_CURVE('',#14380,#14382,#2979,.T.);
#18551=EDGE_CURVE('',#14383,#14384,#9410,.T.);
#18552=EDGE_CURVE('',#14383,#14381,#2980,.T.);
#18553=EDGE_CURVE('',#14382,#14384,#2981,.T.);
#18554=EDGE_CURVE('',#14385,#14386,#9411,.T.);
#18555=EDGE_CURVE('',#14385,#14383,#2982,.T.);
#18556=EDGE_CURVE('',#14384,#14386,#2983,.T.);
#18557=EDGE_CURVE('',#14387,#14388,#9412,.T.);
#18558=EDGE_CURVE('',#14387,#14385,#2984,.T.);
#18559=EDGE_CURVE('',#14386,#14388,#2985,.T.);
#18560=EDGE_CURVE('',#14389,#14390,#9413,.T.);
#18561=EDGE_CURVE('',#14389,#14387,#2986,.T.);
#18562=EDGE_CURVE('',#14388,#14390,#2987,.T.);
#18563=EDGE_CURVE('',#14391,#14392,#9414,.T.);
#18564=EDGE_CURVE('',#14391,#14389,#2988,.T.);
#18565=EDGE_CURVE('',#14390,#14392,#2989,.T.);
#18566=EDGE_CURVE('',#14393,#14394,#9415,.T.);
#18567=EDGE_CURVE('',#14393,#14391,#2990,.T.);
#18568=EDGE_CURVE('',#14392,#14394,#2991,.T.);
#18569=EDGE_CURVE('',#14395,#14396,#9416,.T.);
#18570=EDGE_CURVE('',#14395,#14393,#2992,.T.);
#18571=EDGE_CURVE('',#14394,#14396,#2993,.T.);
#18572=EDGE_CURVE('',#14397,#14398,#9417,.T.);
#18573=EDGE_CURVE('',#14397,#14395,#2994,.T.);
#18574=EDGE_CURVE('',#14396,#14398,#2995,.T.);
#18575=EDGE_CURVE('',#14399,#14400,#9418,.T.);
#18576=EDGE_CURVE('',#14399,#14397,#2996,.T.);
#18577=EDGE_CURVE('',#14398,#14400,#2997,.T.);
#18578=EDGE_CURVE('',#14401,#14402,#9419,.T.);
#18579=EDGE_CURVE('',#14401,#14399,#2998,.T.);
#18580=EDGE_CURVE('',#14400,#14402,#2999,.T.);
#18581=EDGE_CURVE('',#14403,#14404,#9420,.T.);
#18582=EDGE_CURVE('',#14403,#14401,#3000,.T.);
#18583=EDGE_CURVE('',#14402,#14404,#3001,.T.);
#18584=EDGE_CURVE('',#14405,#14406,#9421,.T.);
#18585=EDGE_CURVE('',#14405,#14403,#3002,.T.);
#18586=EDGE_CURVE('',#14404,#14406,#3003,.T.);
#18587=EDGE_CURVE('',#14407,#14408,#9422,.T.);
#18588=EDGE_CURVE('',#14407,#14405,#3004,.T.);
#18589=EDGE_CURVE('',#14406,#14408,#3005,.T.);
#18590=EDGE_CURVE('',#14409,#14410,#9423,.T.);
#18591=EDGE_CURVE('',#14409,#14407,#3006,.T.);
#18592=EDGE_CURVE('',#14408,#14410,#3007,.T.);
#18593=EDGE_CURVE('',#14411,#14412,#9424,.T.);
#18594=EDGE_CURVE('',#14411,#14409,#3008,.T.);
#18595=EDGE_CURVE('',#14410,#14412,#3009,.T.);
#18596=EDGE_CURVE('',#14413,#14414,#9425,.T.);
#18597=EDGE_CURVE('',#14413,#14411,#3010,.T.);
#18598=EDGE_CURVE('',#14412,#14414,#3011,.T.);
#18599=EDGE_CURVE('',#14415,#14416,#9426,.T.);
#18600=EDGE_CURVE('',#14415,#14413,#3012,.T.);
#18601=EDGE_CURVE('',#14414,#14416,#3013,.T.);
#18602=EDGE_CURVE('',#14417,#14418,#9427,.T.);
#18603=EDGE_CURVE('',#14417,#14415,#3014,.T.);
#18604=EDGE_CURVE('',#14416,#14418,#3015,.T.);
#18605=EDGE_CURVE('',#14419,#14420,#9428,.T.);
#18606=EDGE_CURVE('',#14419,#14417,#3016,.T.);
#18607=EDGE_CURVE('',#14418,#14420,#3017,.T.);
#18608=EDGE_CURVE('',#14421,#14422,#9429,.T.);
#18609=EDGE_CURVE('',#14421,#14419,#3018,.T.);
#18610=EDGE_CURVE('',#14420,#14422,#3019,.T.);
#18611=EDGE_CURVE('',#14423,#14424,#9430,.T.);
#18612=EDGE_CURVE('',#14423,#14421,#3020,.T.);
#18613=EDGE_CURVE('',#14422,#14424,#3021,.T.);
#18614=EDGE_CURVE('',#14425,#14426,#9431,.T.);
#18615=EDGE_CURVE('',#14425,#14423,#3022,.T.);
#18616=EDGE_CURVE('',#14424,#14426,#3023,.T.);
#18617=EDGE_CURVE('',#14427,#14428,#9432,.T.);
#18618=EDGE_CURVE('',#14427,#14425,#3024,.T.);
#18619=EDGE_CURVE('',#14426,#14428,#3025,.T.);
#18620=EDGE_CURVE('',#14429,#14430,#9433,.T.);
#18621=EDGE_CURVE('',#14429,#14427,#3026,.T.);
#18622=EDGE_CURVE('',#14428,#14430,#3027,.T.);
#18623=EDGE_CURVE('',#14431,#14432,#9434,.T.);
#18624=EDGE_CURVE('',#14431,#14429,#3028,.T.);
#18625=EDGE_CURVE('',#14430,#14432,#3029,.T.);
#18626=EDGE_CURVE('',#14433,#14434,#9435,.T.);
#18627=EDGE_CURVE('',#14433,#14431,#3030,.T.);
#18628=EDGE_CURVE('',#14432,#14434,#3031,.T.);
#18629=EDGE_CURVE('',#14435,#14436,#9436,.T.);
#18630=EDGE_CURVE('',#14435,#14433,#3032,.T.);
#18631=EDGE_CURVE('',#14434,#14436,#3033,.T.);
#18632=EDGE_CURVE('',#14437,#14438,#9437,.T.);
#18633=EDGE_CURVE('',#14437,#14435,#3034,.T.);
#18634=EDGE_CURVE('',#14436,#14438,#3035,.T.);
#18635=EDGE_CURVE('',#14439,#14440,#9438,.T.);
#18636=EDGE_CURVE('',#14439,#14437,#3036,.T.);
#18637=EDGE_CURVE('',#14438,#14440,#3037,.T.);
#18638=EDGE_CURVE('',#14441,#14442,#9439,.T.);
#18639=EDGE_CURVE('',#14441,#14439,#3038,.T.);
#18640=EDGE_CURVE('',#14440,#14442,#3039,.T.);
#18641=EDGE_CURVE('',#14443,#14444,#9440,.T.);
#18642=EDGE_CURVE('',#14443,#14441,#3040,.T.);
#18643=EDGE_CURVE('',#14442,#14444,#3041,.T.);
#18644=EDGE_CURVE('',#14445,#14446,#9441,.T.);
#18645=EDGE_CURVE('',#14445,#14443,#3042,.T.);
#18646=EDGE_CURVE('',#14444,#14446,#3043,.T.);
#18647=EDGE_CURVE('',#14447,#14448,#9442,.T.);
#18648=EDGE_CURVE('',#14447,#14445,#3044,.T.);
#18649=EDGE_CURVE('',#14446,#14448,#3045,.T.);
#18650=EDGE_CURVE('',#14449,#14450,#9443,.T.);
#18651=EDGE_CURVE('',#14449,#14447,#3046,.T.);
#18652=EDGE_CURVE('',#14448,#14450,#3047,.T.);
#18653=EDGE_CURVE('',#14451,#14452,#9444,.T.);
#18654=EDGE_CURVE('',#14451,#14449,#3048,.T.);
#18655=EDGE_CURVE('',#14450,#14452,#3049,.T.);
#18656=EDGE_CURVE('',#14453,#14454,#9445,.T.);
#18657=EDGE_CURVE('',#14453,#14451,#3050,.T.);
#18658=EDGE_CURVE('',#14452,#14454,#3051,.T.);
#18659=EDGE_CURVE('',#14455,#14456,#9446,.T.);
#18660=EDGE_CURVE('',#14455,#14453,#3052,.T.);
#18661=EDGE_CURVE('',#14454,#14456,#3053,.T.);
#18662=EDGE_CURVE('',#14457,#14458,#9447,.T.);
#18663=EDGE_CURVE('',#14457,#14455,#3054,.T.);
#18664=EDGE_CURVE('',#14456,#14458,#3055,.T.);
#18665=EDGE_CURVE('',#14459,#14460,#9448,.T.);
#18666=EDGE_CURVE('',#14459,#14457,#3056,.T.);
#18667=EDGE_CURVE('',#14458,#14460,#3057,.T.);
#18668=EDGE_CURVE('',#14461,#14462,#9449,.T.);
#18669=EDGE_CURVE('',#14461,#14459,#3058,.T.);
#18670=EDGE_CURVE('',#14460,#14462,#3059,.T.);
#18671=EDGE_CURVE('',#14463,#14464,#9450,.T.);
#18672=EDGE_CURVE('',#14463,#14461,#3060,.T.);
#18673=EDGE_CURVE('',#14462,#14464,#3061,.T.);
#18674=EDGE_CURVE('',#14465,#14466,#9451,.T.);
#18675=EDGE_CURVE('',#14465,#14467,#3062,.T.);
#18676=EDGE_CURVE('',#14468,#14467,#1766,.T.);
#18677=EDGE_CURVE('',#14466,#14468,#3063,.T.);
#18678=EDGE_CURVE('',#14469,#14470,#9452,.T.);
#18679=EDGE_CURVE('',#14469,#14465,#3064,.T.);
#18680=EDGE_CURVE('',#14470,#14466,#3065,.T.);
#18681=EDGE_CURVE('',#14471,#14472,#9453,.T.);
#18682=EDGE_CURVE('',#14471,#14469,#3066,.T.);
#18683=EDGE_CURVE('',#14472,#14470,#3067,.T.);
#18684=EDGE_CURVE('',#14473,#14474,#9454,.T.);
#18685=EDGE_CURVE('',#14473,#14471,#3068,.T.);
#18686=EDGE_CURVE('',#14474,#14472,#3069,.T.);
#18687=EDGE_CURVE('',#14475,#14476,#9455,.T.);
#18688=EDGE_CURVE('',#14475,#14473,#3070,.T.);
#18689=EDGE_CURVE('',#14476,#14474,#3071,.T.);
#18690=EDGE_CURVE('',#14477,#14478,#9456,.T.);
#18691=EDGE_CURVE('',#14477,#14475,#3072,.T.);
#18692=EDGE_CURVE('',#14478,#14476,#3073,.T.);
#18693=EDGE_CURVE('',#14479,#14480,#9457,.T.);
#18694=EDGE_CURVE('',#14479,#14477,#3074,.T.);
#18695=EDGE_CURVE('',#14480,#14478,#3075,.T.);
#18696=EDGE_CURVE('',#14481,#14482,#9458,.T.);
#18697=EDGE_CURVE('',#14481,#14479,#3076,.T.);
#18698=EDGE_CURVE('',#14482,#14480,#3077,.T.);
#18699=EDGE_CURVE('',#14483,#14484,#9459,.T.);
#18700=EDGE_CURVE('',#14483,#14481,#3078,.T.);
#18701=EDGE_CURVE('',#14484,#14482,#3079,.T.);
#18702=EDGE_CURVE('',#14485,#14486,#9460,.T.);
#18703=EDGE_CURVE('',#14485,#14483,#3080,.T.);
#18704=EDGE_CURVE('',#14486,#14484,#3081,.T.);
#18705=EDGE_CURVE('',#14487,#14488,#9461,.T.);
#18706=EDGE_CURVE('',#14487,#14485,#3082,.T.);
#18707=EDGE_CURVE('',#14488,#14486,#3083,.T.);
#18708=EDGE_CURVE('',#14489,#14490,#9462,.T.);
#18709=EDGE_CURVE('',#14489,#14487,#3084,.T.);
#18710=EDGE_CURVE('',#14490,#14488,#3085,.T.);
#18711=EDGE_CURVE('',#14491,#14492,#9463,.T.);
#18712=EDGE_CURVE('',#14491,#14489,#3086,.T.);
#18713=EDGE_CURVE('',#14492,#14490,#3087,.T.);
#18714=EDGE_CURVE('',#14493,#14494,#9464,.T.);
#18715=EDGE_CURVE('',#14493,#14491,#3088,.T.);
#18716=EDGE_CURVE('',#14494,#14492,#3089,.T.);
#18717=EDGE_CURVE('',#14495,#14496,#9465,.T.);
#18718=EDGE_CURVE('',#14495,#14493,#3090,.T.);
#18719=EDGE_CURVE('',#14496,#14494,#3091,.T.);
#18720=EDGE_CURVE('',#14497,#14498,#9466,.T.);
#18721=EDGE_CURVE('',#14497,#14495,#3092,.T.);
#18722=EDGE_CURVE('',#14498,#14496,#3093,.T.);
#18723=EDGE_CURVE('',#14499,#14500,#9467,.T.);
#18724=EDGE_CURVE('',#14499,#14497,#3094,.T.);
#18725=EDGE_CURVE('',#14500,#14498,#3095,.T.);
#18726=EDGE_CURVE('',#14501,#14502,#9468,.T.);
#18727=EDGE_CURVE('',#14501,#14499,#3096,.T.);
#18728=EDGE_CURVE('',#14502,#14500,#3097,.T.);
#18729=EDGE_CURVE('',#14503,#14504,#9469,.T.);
#18730=EDGE_CURVE('',#14503,#14501,#3098,.T.);
#18731=EDGE_CURVE('',#14504,#14502,#3099,.T.);
#18732=EDGE_CURVE('',#14505,#14506,#9470,.T.);
#18733=EDGE_CURVE('',#14505,#14503,#3100,.T.);
#18734=EDGE_CURVE('',#14506,#14504,#3101,.T.);
#18735=EDGE_CURVE('',#14507,#14508,#9471,.T.);
#18736=EDGE_CURVE('',#14507,#14505,#3102,.T.);
#18737=EDGE_CURVE('',#14508,#14506,#3103,.T.);
#18738=EDGE_CURVE('',#14509,#14510,#9472,.T.);
#18739=EDGE_CURVE('',#14509,#14507,#3104,.T.);
#18740=EDGE_CURVE('',#14510,#14508,#3105,.T.);
#18741=EDGE_CURVE('',#14511,#14512,#9473,.T.);
#18742=EDGE_CURVE('',#14511,#14509,#3106,.T.);
#18743=EDGE_CURVE('',#14512,#14510,#3107,.T.);
#18744=EDGE_CURVE('',#14513,#14514,#9474,.T.);
#18745=EDGE_CURVE('',#14513,#14511,#3108,.T.);
#18746=EDGE_CURVE('',#14514,#14512,#3109,.T.);
#18747=EDGE_CURVE('',#14515,#14516,#9475,.T.);
#18748=EDGE_CURVE('',#14515,#14513,#3110,.T.);
#18749=EDGE_CURVE('',#14516,#14514,#3111,.T.);
#18750=EDGE_CURVE('',#14517,#14518,#9476,.T.);
#18751=EDGE_CURVE('',#14517,#14515,#3112,.T.);
#18752=EDGE_CURVE('',#14518,#14516,#3113,.T.);
#18753=EDGE_CURVE('',#14519,#14520,#9477,.T.);
#18754=EDGE_CURVE('',#14519,#14517,#3114,.T.);
#18755=EDGE_CURVE('',#14520,#14518,#3115,.T.);
#18756=EDGE_CURVE('',#14521,#14522,#9478,.T.);
#18757=EDGE_CURVE('',#14521,#14519,#3116,.T.);
#18758=EDGE_CURVE('',#14522,#14520,#3117,.T.);
#18759=EDGE_CURVE('',#14523,#14524,#9479,.T.);
#18760=EDGE_CURVE('',#14523,#14521,#3118,.T.);
#18761=EDGE_CURVE('',#14524,#14522,#3119,.T.);
#18762=EDGE_CURVE('',#14525,#14526,#9480,.T.);
#18763=EDGE_CURVE('',#14525,#14523,#3120,.T.);
#18764=EDGE_CURVE('',#14526,#14524,#3121,.T.);
#18765=EDGE_CURVE('',#14527,#14528,#9481,.T.);
#18766=EDGE_CURVE('',#14527,#14525,#3122,.T.);
#18767=EDGE_CURVE('',#14528,#14526,#3123,.T.);
#18768=EDGE_CURVE('',#14529,#14530,#9482,.T.);
#18769=EDGE_CURVE('',#14529,#14527,#3124,.T.);
#18770=EDGE_CURVE('',#14530,#14528,#3125,.T.);
#18771=EDGE_CURVE('',#14531,#14532,#9483,.T.);
#18772=EDGE_CURVE('',#14531,#14529,#3126,.T.);
#18773=EDGE_CURVE('',#14532,#14530,#3127,.T.);
#18774=EDGE_CURVE('',#14533,#14534,#9484,.T.);
#18775=EDGE_CURVE('',#14533,#14531,#3128,.T.);
#18776=EDGE_CURVE('',#14534,#14532,#3129,.T.);
#18777=EDGE_CURVE('',#14535,#14536,#9485,.T.);
#18778=EDGE_CURVE('',#14535,#14533,#3130,.T.);
#18779=EDGE_CURVE('',#14536,#14534,#3131,.T.);
#18780=EDGE_CURVE('',#14537,#14538,#9486,.T.);
#18781=EDGE_CURVE('',#14537,#14535,#3132,.T.);
#18782=EDGE_CURVE('',#14538,#14536,#3133,.T.);
#18783=EDGE_CURVE('',#14539,#14540,#9487,.T.);
#18784=EDGE_CURVE('',#14539,#14537,#3134,.T.);
#18785=EDGE_CURVE('',#14540,#14538,#3135,.T.);
#18786=EDGE_CURVE('',#14541,#14542,#9488,.T.);
#18787=EDGE_CURVE('',#14541,#14539,#3136,.T.);
#18788=EDGE_CURVE('',#14542,#14540,#3137,.T.);
#18789=EDGE_CURVE('',#14543,#14544,#9489,.T.);
#18790=EDGE_CURVE('',#14543,#14541,#3138,.T.);
#18791=EDGE_CURVE('',#14544,#14542,#3139,.T.);
#18792=EDGE_CURVE('',#14545,#14546,#9490,.T.);
#18793=EDGE_CURVE('',#14545,#14543,#3140,.T.);
#18794=EDGE_CURVE('',#14546,#14544,#3141,.T.);
#18795=EDGE_CURVE('',#14547,#14548,#9491,.T.);
#18796=EDGE_CURVE('',#14547,#14545,#3142,.T.);
#18797=EDGE_CURVE('',#14548,#14546,#3143,.T.);
#18798=EDGE_CURVE('',#14549,#14550,#9492,.T.);
#18799=EDGE_CURVE('',#14549,#14547,#3144,.T.);
#18800=EDGE_CURVE('',#14550,#14548,#3145,.T.);
#18801=EDGE_CURVE('',#14551,#14552,#9493,.T.);
#18802=EDGE_CURVE('',#14551,#14549,#3146,.T.);
#18803=EDGE_CURVE('',#14552,#14550,#3147,.T.);
#18804=EDGE_CURVE('',#14553,#14554,#9494,.T.);
#18805=EDGE_CURVE('',#14553,#14551,#3148,.T.);
#18806=EDGE_CURVE('',#14554,#14552,#3149,.T.);
#18807=EDGE_CURVE('',#14555,#14556,#9495,.T.);
#18808=EDGE_CURVE('',#14555,#14553,#3150,.T.);
#18809=EDGE_CURVE('',#14556,#14554,#3151,.T.);
#18810=EDGE_CURVE('',#14557,#14558,#9496,.T.);
#18811=EDGE_CURVE('',#14557,#14555,#3152,.T.);
#18812=EDGE_CURVE('',#14558,#14556,#3153,.T.);
#18813=EDGE_CURVE('',#14559,#14560,#9497,.T.);
#18814=EDGE_CURVE('',#14559,#14557,#3154,.T.);
#18815=EDGE_CURVE('',#14560,#14558,#3155,.T.);
#18816=EDGE_CURVE('',#14561,#14562,#9498,.T.);
#18817=EDGE_CURVE('',#14561,#14559,#3156,.T.);
#18818=EDGE_CURVE('',#14562,#14560,#3157,.T.);
#18819=EDGE_CURVE('',#14563,#14564,#9499,.T.);
#18820=EDGE_CURVE('',#14563,#14561,#3158,.T.);
#18821=EDGE_CURVE('',#14564,#14562,#3159,.T.);
#18822=EDGE_CURVE('',#14565,#14566,#9500,.T.);
#18823=EDGE_CURVE('',#14565,#14563,#3160,.T.);
#18824=EDGE_CURVE('',#14566,#14564,#3161,.T.);
#18825=EDGE_CURVE('',#14567,#14568,#9501,.T.);
#18826=EDGE_CURVE('',#14567,#14565,#3162,.T.);
#18827=EDGE_CURVE('',#14568,#14566,#3163,.T.);
#18828=EDGE_CURVE('',#14569,#14570,#9502,.T.);
#18829=EDGE_CURVE('',#14569,#14567,#3164,.T.);
#18830=EDGE_CURVE('',#14570,#14568,#3165,.T.);
#18831=EDGE_CURVE('',#14571,#14572,#9503,.T.);
#18832=EDGE_CURVE('',#14571,#14569,#3166,.T.);
#18833=EDGE_CURVE('',#14572,#14570,#3167,.T.);
#18834=EDGE_CURVE('',#14573,#14574,#9504,.T.);
#18835=EDGE_CURVE('',#14573,#14571,#3168,.T.);
#18836=EDGE_CURVE('',#14574,#14572,#3169,.T.);
#18837=EDGE_CURVE('',#14575,#14576,#9505,.T.);
#18838=EDGE_CURVE('',#14575,#14573,#3170,.T.);
#18839=EDGE_CURVE('',#14576,#14574,#3171,.T.);
#18840=EDGE_CURVE('',#14577,#14578,#9506,.T.);
#18841=EDGE_CURVE('',#14577,#14575,#3172,.T.);
#18842=EDGE_CURVE('',#14578,#14576,#3173,.T.);
#18843=EDGE_CURVE('',#14579,#14580,#9507,.T.);
#18844=EDGE_CURVE('',#14579,#14577,#3174,.T.);
#18845=EDGE_CURVE('',#14580,#14578,#3175,.T.);
#18846=EDGE_CURVE('',#14581,#14582,#9508,.T.);
#18847=EDGE_CURVE('',#14581,#14579,#3176,.T.);
#18848=EDGE_CURVE('',#14582,#14580,#3177,.T.);
#18849=EDGE_CURVE('',#14583,#14584,#9509,.T.);
#18850=EDGE_CURVE('',#14583,#14581,#3178,.T.);
#18851=EDGE_CURVE('',#14584,#14582,#3179,.T.);
#18852=EDGE_CURVE('',#14585,#14586,#9510,.T.);
#18853=EDGE_CURVE('',#14585,#14583,#3180,.T.);
#18854=EDGE_CURVE('',#14586,#14584,#3181,.T.);
#18855=EDGE_CURVE('',#14587,#14588,#9511,.T.);
#18856=EDGE_CURVE('',#14587,#14585,#3182,.T.);
#18857=EDGE_CURVE('',#14588,#14586,#3183,.T.);
#18858=EDGE_CURVE('',#14589,#14590,#9512,.T.);
#18859=EDGE_CURVE('',#14589,#14587,#3184,.T.);
#18860=EDGE_CURVE('',#14590,#14588,#3185,.T.);
#18861=EDGE_CURVE('',#14591,#14592,#9513,.T.);
#18862=EDGE_CURVE('',#14591,#14589,#3186,.T.);
#18863=EDGE_CURVE('',#14592,#14590,#3187,.T.);
#18864=EDGE_CURVE('',#14593,#14594,#9514,.T.);
#18865=EDGE_CURVE('',#14593,#14591,#3188,.T.);
#18866=EDGE_CURVE('',#14594,#14592,#3189,.T.);
#18867=EDGE_CURVE('',#14595,#14596,#9515,.T.);
#18868=EDGE_CURVE('',#14595,#14593,#3190,.T.);
#18869=EDGE_CURVE('',#14596,#14594,#3191,.T.);
#18870=EDGE_CURVE('',#14597,#14598,#9516,.T.);
#18871=EDGE_CURVE('',#14597,#14595,#3192,.T.);
#18872=EDGE_CURVE('',#14598,#14596,#3193,.T.);
#18873=EDGE_CURVE('',#14599,#14600,#9517,.T.);
#18874=EDGE_CURVE('',#14599,#14597,#3194,.T.);
#18875=EDGE_CURVE('',#14600,#14598,#3195,.T.);
#18876=EDGE_CURVE('',#14601,#14602,#9518,.T.);
#18877=EDGE_CURVE('',#14601,#14599,#3196,.T.);
#18878=EDGE_CURVE('',#14602,#14600,#3197,.T.);
#18879=EDGE_CURVE('',#14603,#14604,#9519,.T.);
#18880=EDGE_CURVE('',#14603,#14601,#3198,.T.);
#18881=EDGE_CURVE('',#14604,#14602,#3199,.T.);
#18882=EDGE_CURVE('',#14605,#14606,#9520,.T.);
#18883=EDGE_CURVE('',#14605,#14603,#3200,.T.);
#18884=EDGE_CURVE('',#14606,#14604,#3201,.T.);
#18885=EDGE_CURVE('',#14607,#14608,#9521,.T.);
#18886=EDGE_CURVE('',#14607,#14605,#3202,.T.);
#18887=EDGE_CURVE('',#14608,#14606,#3203,.T.);
#18888=EDGE_CURVE('',#14609,#14610,#9522,.T.);
#18889=EDGE_CURVE('',#14609,#14607,#3204,.T.);
#18890=EDGE_CURVE('',#14610,#14608,#3205,.T.);
#18891=EDGE_CURVE('',#14611,#14612,#9523,.T.);
#18892=EDGE_CURVE('',#14611,#14609,#3206,.T.);
#18893=EDGE_CURVE('',#14612,#14610,#3207,.T.);
#18894=EDGE_CURVE('',#14613,#14614,#9524,.T.);
#18895=EDGE_CURVE('',#14613,#14611,#3208,.T.);
#18896=EDGE_CURVE('',#14614,#14612,#3209,.T.);
#18897=EDGE_CURVE('',#14615,#14616,#9525,.T.);
#18898=EDGE_CURVE('',#14615,#14613,#3210,.T.);
#18899=EDGE_CURVE('',#14616,#14614,#3211,.T.);
#18900=EDGE_CURVE('',#14467,#14617,#3212,.T.);
#18901=EDGE_CURVE('',#14618,#14617,#1767,.F.);
#18902=EDGE_CURVE('',#14619,#14618,#1768,.F.);
#18903=EDGE_CURVE('',#14619,#14468,#3213,.T.);
#18904=EDGE_CURVE('',#14464,#14619,#3214,.T.);
#18905=EDGE_CURVE('',#14620,#14316,#3215,.T.);
#18906=EDGE_CURVE('',#14620,#14616,#3216,.T.);
#18907=EDGE_CURVE('',#14316,#14621,#1769,.T.);
#18908=EDGE_CURVE('',#14621,#14315,#1770,.T.);
#18909=EDGE_CURVE('',#14315,#14622,#3217,.T.);
#18910=EDGE_CURVE('',#14622,#14620,#1771,.T.);
#18911=EDGE_CURVE('',#14622,#14615,#3218,.T.);
#18912=EDGE_CURVE('',#14617,#14463,#3219,.T.);
#18913=EDGE_CURVE('',#14623,#14623,#1772,.T.);
#18914=EDGE_CURVE('',#14623,#14624,#9526,.T.);
#18915=EDGE_CURVE('',#14624,#14624,#1773,.T.);
#18916=EDGE_CURVE('',#14621,#14623,#9527,.T.);
#18917=EDGE_CURVE('',#14617,#14619,#1774,.F.);
#18918=EDGE_CURVE('',#14625,#14625,#1775,.T.);
#18919=EDGE_CURVE('',#14625,#14618,#9528,.T.);
#18920=EDGE_CURVE('',#14626,#14627,#1776,.T.);
#26453=ORIENTED_EDGE('',*,*,#18448,.F.);
#26454=ORIENTED_EDGE('',*,*,#18449,.T.);
#26455=ORIENTED_EDGE('',*,*,#18450,.T.);
#26456=ORIENTED_EDGE('',*,*,#18451,.T.);
#26457=ORIENTED_EDGE('',*,*,#18452,.F.);
#26458=ORIENTED_EDGE('',*,*,#18453,.T.);
#26459=ORIENTED_EDGE('',*,*,#18448,.T.);
#26460=ORIENTED_EDGE('',*,*,#18454,.T.);
#26461=ORIENTED_EDGE('',*,*,#18455,.F.);
#26462=ORIENTED_EDGE('',*,*,#18456,.T.);
#26463=ORIENTED_EDGE('',*,*,#18452,.T.);
#26464=ORIENTED_EDGE('',*,*,#18457,.T.);
#26465=ORIENTED_EDGE('',*,*,#18458,.F.);
#26466=ORIENTED_EDGE('',*,*,#18459,.T.);
#26467=ORIENTED_EDGE('',*,*,#18455,.T.);
#26468=ORIENTED_EDGE('',*,*,#18460,.T.);
#26469=ORIENTED_EDGE('',*,*,#18461,.F.);
#26470=ORIENTED_EDGE('',*,*,#18462,.T.);
#26471=ORIENTED_EDGE('',*,*,#18458,.T.);
#26472=ORIENTED_EDGE('',*,*,#18463,.T.);
#26473=ORIENTED_EDGE('',*,*,#18464,.F.);
#26474=ORIENTED_EDGE('',*,*,#18465,.T.);
#26475=ORIENTED_EDGE('',*,*,#18461,.T.);
#26476=ORIENTED_EDGE('',*,*,#18466,.T.);
#26477=ORIENTED_EDGE('',*,*,#18467,.F.);
#26478=ORIENTED_EDGE('',*,*,#18468,.T.);
#26479=ORIENTED_EDGE('',*,*,#18464,.T.);
#26480=ORIENTED_EDGE('',*,*,#18469,.T.);
#26481=ORIENTED_EDGE('',*,*,#18470,.F.);
#26482=ORIENTED_EDGE('',*,*,#18471,.T.);
#26483=ORIENTED_EDGE('',*,*,#18467,.T.);
#26484=ORIENTED_EDGE('',*,*,#18472,.T.);
#26485=ORIENTED_EDGE('',*,*,#18473,.F.);
#26486=ORIENTED_EDGE('',*,*,#18474,.T.);
#26487=ORIENTED_EDGE('',*,*,#18470,.T.);
#26488=ORIENTED_EDGE('',*,*,#18475,.T.);
#26489=ORIENTED_EDGE('',*,*,#18476,.F.);
#26490=ORIENTED_EDGE('',*,*,#18477,.T.);
#26491=ORIENTED_EDGE('',*,*,#18473,.T.);
#26492=ORIENTED_EDGE('',*,*,#18478,.T.);
#26493=ORIENTED_EDGE('',*,*,#18479,.F.);
#26494=ORIENTED_EDGE('',*,*,#18480,.T.);
#26495=ORIENTED_EDGE('',*,*,#18476,.T.);
#26496=ORIENTED_EDGE('',*,*,#18481,.T.);
#26497=ORIENTED_EDGE('',*,*,#18482,.F.);
#26498=ORIENTED_EDGE('',*,*,#18483,.T.);
#26499=ORIENTED_EDGE('',*,*,#18479,.T.);
#26500=ORIENTED_EDGE('',*,*,#18484,.T.);
#26501=ORIENTED_EDGE('',*,*,#18485,.F.);
#26502=ORIENTED_EDGE('',*,*,#18486,.T.);
#26503=ORIENTED_EDGE('',*,*,#18482,.T.);
#26504=ORIENTED_EDGE('',*,*,#18487,.T.);
#26505=ORIENTED_EDGE('',*,*,#18488,.F.);
#26506=ORIENTED_EDGE('',*,*,#18489,.T.);
#26507=ORIENTED_EDGE('',*,*,#18485,.T.);
#26508=ORIENTED_EDGE('',*,*,#18490,.T.);
#26509=ORIENTED_EDGE('',*,*,#18491,.F.);
#26510=ORIENTED_EDGE('',*,*,#18492,.T.);
#26511=ORIENTED_EDGE('',*,*,#18488,.T.);
#26512=ORIENTED_EDGE('',*,*,#18493,.T.);
#26513=ORIENTED_EDGE('',*,*,#18494,.F.);
#26514=ORIENTED_EDGE('',*,*,#18495,.T.);
#26515=ORIENTED_EDGE('',*,*,#18491,.T.);
#26516=ORIENTED_EDGE('',*,*,#18496,.T.);
#26517=ORIENTED_EDGE('',*,*,#18497,.F.);
#26518=ORIENTED_EDGE('',*,*,#18498,.T.);
#26519=ORIENTED_EDGE('',*,*,#18494,.T.);
#26520=ORIENTED_EDGE('',*,*,#18499,.T.);
#26521=ORIENTED_EDGE('',*,*,#18500,.F.);
#26522=ORIENTED_EDGE('',*,*,#18501,.T.);
#26523=ORIENTED_EDGE('',*,*,#18497,.T.);
#26524=ORIENTED_EDGE('',*,*,#18502,.T.);
#26525=ORIENTED_EDGE('',*,*,#18503,.F.);
#26526=ORIENTED_EDGE('',*,*,#18504,.T.);
#26527=ORIENTED_EDGE('',*,*,#18500,.T.);
#26528=ORIENTED_EDGE('',*,*,#18505,.T.);
#26529=ORIENTED_EDGE('',*,*,#18506,.F.);
#26530=ORIENTED_EDGE('',*,*,#18507,.T.);
#26531=ORIENTED_EDGE('',*,*,#18503,.T.);
#26532=ORIENTED_EDGE('',*,*,#18508,.T.);
#26533=ORIENTED_EDGE('',*,*,#18509,.F.);
#26534=ORIENTED_EDGE('',*,*,#18510,.T.);
#26535=ORIENTED_EDGE('',*,*,#18506,.T.);
#26536=ORIENTED_EDGE('',*,*,#18511,.T.);
#26537=ORIENTED_EDGE('',*,*,#18512,.F.);
#26538=ORIENTED_EDGE('',*,*,#18513,.T.);
#26539=ORIENTED_EDGE('',*,*,#18509,.T.);
#26540=ORIENTED_EDGE('',*,*,#18514,.T.);
#26541=ORIENTED_EDGE('',*,*,#18515,.F.);
#26542=ORIENTED_EDGE('',*,*,#18516,.T.);
#26543=ORIENTED_EDGE('',*,*,#18512,.T.);
#26544=ORIENTED_EDGE('',*,*,#18517,.T.);
#26545=ORIENTED_EDGE('',*,*,#18518,.F.);
#26546=ORIENTED_EDGE('',*,*,#18519,.T.);
#26547=ORIENTED_EDGE('',*,*,#18515,.T.);
#26548=ORIENTED_EDGE('',*,*,#18520,.T.);
#26549=ORIENTED_EDGE('',*,*,#18521,.F.);
#26550=ORIENTED_EDGE('',*,*,#18522,.T.);
#26551=ORIENTED_EDGE('',*,*,#18518,.T.);
#26552=ORIENTED_EDGE('',*,*,#18523,.T.);
#26553=ORIENTED_EDGE('',*,*,#18524,.F.);
#26554=ORIENTED_EDGE('',*,*,#18525,.T.);
#26555=ORIENTED_EDGE('',*,*,#18521,.T.);
#26556=ORIENTED_EDGE('',*,*,#18526,.T.);
#26557=ORIENTED_EDGE('',*,*,#18527,.F.);
#26558=ORIENTED_EDGE('',*,*,#18528,.T.);
#26559=ORIENTED_EDGE('',*,*,#18524,.T.);
#26560=ORIENTED_EDGE('',*,*,#18529,.T.);
#26561=ORIENTED_EDGE('',*,*,#18530,.F.);
#26562=ORIENTED_EDGE('',*,*,#18531,.T.);
#26563=ORIENTED_EDGE('',*,*,#18527,.T.);
#26564=ORIENTED_EDGE('',*,*,#18532,.T.);
#26565=ORIENTED_EDGE('',*,*,#18533,.F.);
#26566=ORIENTED_EDGE('',*,*,#18534,.T.);
#26567=ORIENTED_EDGE('',*,*,#18530,.T.);
#26568=ORIENTED_EDGE('',*,*,#18535,.T.);
#26569=ORIENTED_EDGE('',*,*,#18536,.F.);
#26570=ORIENTED_EDGE('',*,*,#18537,.T.);
#26571=ORIENTED_EDGE('',*,*,#18533,.T.);
#26572=ORIENTED_EDGE('',*,*,#18538,.T.);
#26573=ORIENTED_EDGE('',*,*,#18539,.F.);
#26574=ORIENTED_EDGE('',*,*,#18540,.T.);
#26575=ORIENTED_EDGE('',*,*,#18536,.T.);
#26576=ORIENTED_EDGE('',*,*,#18541,.T.);
#26577=ORIENTED_EDGE('',*,*,#18542,.F.);
#26578=ORIENTED_EDGE('',*,*,#18543,.T.);
#26579=ORIENTED_EDGE('',*,*,#18539,.T.);
#26580=ORIENTED_EDGE('',*,*,#18544,.T.);
#26581=ORIENTED_EDGE('',*,*,#18545,.F.);
#26582=ORIENTED_EDGE('',*,*,#18546,.T.);
#26583=ORIENTED_EDGE('',*,*,#18542,.T.);
#26584=ORIENTED_EDGE('',*,*,#18547,.T.);
#26585=ORIENTED_EDGE('',*,*,#18548,.F.);
#26586=ORIENTED_EDGE('',*,*,#18549,.T.);
#26587=ORIENTED_EDGE('',*,*,#18545,.T.);
#26588=ORIENTED_EDGE('',*,*,#18550,.T.);
#26589=ORIENTED_EDGE('',*,*,#18551,.F.);
#26590=ORIENTED_EDGE('',*,*,#18552,.T.);
#26591=ORIENTED_EDGE('',*,*,#18548,.T.);
#26592=ORIENTED_EDGE('',*,*,#18553,.T.);
#26593=ORIENTED_EDGE('',*,*,#18554,.F.);
#26594=ORIENTED_EDGE('',*,*,#18555,.T.);
#26595=ORIENTED_EDGE('',*,*,#18551,.T.);
#26596=ORIENTED_EDGE('',*,*,#18556,.T.);
#26597=ORIENTED_EDGE('',*,*,#18557,.F.);
#26598=ORIENTED_EDGE('',*,*,#18558,.T.);
#26599=ORIENTED_EDGE('',*,*,#18554,.T.);
#26600=ORIENTED_EDGE('',*,*,#18559,.T.);
#26601=ORIENTED_EDGE('',*,*,#18560,.F.);
#26602=ORIENTED_EDGE('',*,*,#18561,.T.);
#26603=ORIENTED_EDGE('',*,*,#18557,.T.);
#26604=ORIENTED_EDGE('',*,*,#18562,.T.);
#26605=ORIENTED_EDGE('',*,*,#18563,.F.);
#26606=ORIENTED_EDGE('',*,*,#18564,.T.);
#26607=ORIENTED_EDGE('',*,*,#18560,.T.);
#26608=ORIENTED_EDGE('',*,*,#18565,.T.);
#26609=ORIENTED_EDGE('',*,*,#18566,.F.);
#26610=ORIENTED_EDGE('',*,*,#18567,.T.);
#26611=ORIENTED_EDGE('',*,*,#18563,.T.);
#26612=ORIENTED_EDGE('',*,*,#18568,.T.);
#26613=ORIENTED_EDGE('',*,*,#18569,.F.);
#26614=ORIENTED_EDGE('',*,*,#18570,.T.);
#26615=ORIENTED_EDGE('',*,*,#18566,.T.);
#26616=ORIENTED_EDGE('',*,*,#18571,.T.);
#26617=ORIENTED_EDGE('',*,*,#18572,.F.);
#26618=ORIENTED_EDGE('',*,*,#18573,.T.);
#26619=ORIENTED_EDGE('',*,*,#18569,.T.);
#26620=ORIENTED_EDGE('',*,*,#18574,.T.);
#26621=ORIENTED_EDGE('',*,*,#18575,.F.);
#26622=ORIENTED_EDGE('',*,*,#18576,.T.);
#26623=ORIENTED_EDGE('',*,*,#18572,.T.);
#26624=ORIENTED_EDGE('',*,*,#18577,.T.);
#26625=ORIENTED_EDGE('',*,*,#18578,.F.);
#26626=ORIENTED_EDGE('',*,*,#18579,.T.);
#26627=ORIENTED_EDGE('',*,*,#18575,.T.);
#26628=ORIENTED_EDGE('',*,*,#18580,.T.);
#26629=ORIENTED_EDGE('',*,*,#18581,.F.);
#26630=ORIENTED_EDGE('',*,*,#18582,.T.);
#26631=ORIENTED_EDGE('',*,*,#18578,.T.);
#26632=ORIENTED_EDGE('',*,*,#18583,.T.);
#26633=ORIENTED_EDGE('',*,*,#18584,.F.);
#26634=ORIENTED_EDGE('',*,*,#18585,.T.);
#26635=ORIENTED_EDGE('',*,*,#18581,.T.);
#26636=ORIENTED_EDGE('',*,*,#18586,.T.);
#26637=ORIENTED_EDGE('',*,*,#18587,.F.);
#26638=ORIENTED_EDGE('',*,*,#18588,.T.);
#26639=ORIENTED_EDGE('',*,*,#18584,.T.);
#26640=ORIENTED_EDGE('',*,*,#18589,.T.);
#26641=ORIENTED_EDGE('',*,*,#18590,.F.);
#26642=ORIENTED_EDGE('',*,*,#18591,.T.);
#26643=ORIENTED_EDGE('',*,*,#18587,.T.);
#26644=ORIENTED_EDGE('',*,*,#18592,.T.);
#26645=ORIENTED_EDGE('',*,*,#18593,.F.);
#26646=ORIENTED_EDGE('',*,*,#18594,.T.);
#26647=ORIENTED_EDGE('',*,*,#18590,.T.);
#26648=ORIENTED_EDGE('',*,*,#18595,.T.);
#26649=ORIENTED_EDGE('',*,*,#18596,.F.);
#26650=ORIENTED_EDGE('',*,*,#18597,.T.);
#26651=ORIENTED_EDGE('',*,*,#18593,.T.);
#26652=ORIENTED_EDGE('',*,*,#18598,.T.);
#26653=ORIENTED_EDGE('',*,*,#18599,.F.);
#26654=ORIENTED_EDGE('',*,*,#18600,.T.);
#26655=ORIENTED_EDGE('',*,*,#18596,.T.);
#26656=ORIENTED_EDGE('',*,*,#18601,.T.);
#26657=ORIENTED_EDGE('',*,*,#18602,.F.);
#26658=ORIENTED_EDGE('',*,*,#18603,.T.);
#26659=ORIENTED_EDGE('',*,*,#18599,.T.);
#26660=ORIENTED_EDGE('',*,*,#18604,.T.);
#26661=ORIENTED_EDGE('',*,*,#18605,.F.);
#26662=ORIENTED_EDGE('',*,*,#18606,.T.);
#26663=ORIENTED_EDGE('',*,*,#18602,.T.);
#26664=ORIENTED_EDGE('',*,*,#18607,.T.);
#26665=ORIENTED_EDGE('',*,*,#18608,.F.);
#26666=ORIENTED_EDGE('',*,*,#18609,.T.);
#26667=ORIENTED_EDGE('',*,*,#18605,.T.);
#26668=ORIENTED_EDGE('',*,*,#18610,.T.);
#26669=ORIENTED_EDGE('',*,*,#18611,.F.);
#26670=ORIENTED_EDGE('',*,*,#18612,.T.);
#26671=ORIENTED_EDGE('',*,*,#18608,.T.);
#26672=ORIENTED_EDGE('',*,*,#18613,.T.);
#26673=ORIENTED_EDGE('',*,*,#18614,.F.);
#26674=ORIENTED_EDGE('',*,*,#18615,.T.);
#26675=ORIENTED_EDGE('',*,*,#18611,.T.);
#26676=ORIENTED_EDGE('',*,*,#18616,.T.);
#26677=ORIENTED_EDGE('',*,*,#18617,.F.);
#26678=ORIENTED_EDGE('',*,*,#18618,.T.);
#26679=ORIENTED_EDGE('',*,*,#18614,.T.);
#26680=ORIENTED_EDGE('',*,*,#18619,.T.);
#26681=ORIENTED_EDGE('',*,*,#18620,.F.);
#26682=ORIENTED_EDGE('',*,*,#18621,.T.);
#26683=ORIENTED_EDGE('',*,*,#18617,.T.);
#26684=ORIENTED_EDGE('',*,*,#18622,.T.);
#26685=ORIENTED_EDGE('',*,*,#18623,.F.);
#26686=ORIENTED_EDGE('',*,*,#18624,.T.);
#26687=ORIENTED_EDGE('',*,*,#18620,.T.);
#26688=ORIENTED_EDGE('',*,*,#18625,.T.);
#26689=ORIENTED_EDGE('',*,*,#18626,.F.);
#26690=ORIENTED_EDGE('',*,*,#18627,.T.);
#26691=ORIENTED_EDGE('',*,*,#18623,.T.);
#26692=ORIENTED_EDGE('',*,*,#18628,.T.);
#26693=ORIENTED_EDGE('',*,*,#18629,.F.);
#26694=ORIENTED_EDGE('',*,*,#18630,.T.);
#26695=ORIENTED_EDGE('',*,*,#18626,.T.);
#26696=ORIENTED_EDGE('',*,*,#18631,.T.);
#26697=ORIENTED_EDGE('',*,*,#18632,.F.);
#26698=ORIENTED_EDGE('',*,*,#18633,.T.);
#26699=ORIENTED_EDGE('',*,*,#18629,.T.);
#26700=ORIENTED_EDGE('',*,*,#18634,.T.);
#26701=ORIENTED_EDGE('',*,*,#18635,.F.);
#26702=ORIENTED_EDGE('',*,*,#18636,.T.);
#26703=ORIENTED_EDGE('',*,*,#18632,.T.);
#26704=ORIENTED_EDGE('',*,*,#18637,.T.);
#26705=ORIENTED_EDGE('',*,*,#18638,.F.);
#26706=ORIENTED_EDGE('',*,*,#18639,.T.);
#26707=ORIENTED_EDGE('',*,*,#18635,.T.);
#26708=ORIENTED_EDGE('',*,*,#18640,.T.);
#26709=ORIENTED_EDGE('',*,*,#18641,.F.);
#26710=ORIENTED_EDGE('',*,*,#18642,.T.);
#26711=ORIENTED_EDGE('',*,*,#18638,.T.);
#26712=ORIENTED_EDGE('',*,*,#18643,.T.);
#26713=ORIENTED_EDGE('',*,*,#18644,.F.);
#26714=ORIENTED_EDGE('',*,*,#18645,.T.);
#26715=ORIENTED_EDGE('',*,*,#18641,.T.);
#26716=ORIENTED_EDGE('',*,*,#18646,.T.);
#26717=ORIENTED_EDGE('',*,*,#18647,.F.);
#26718=ORIENTED_EDGE('',*,*,#18648,.T.);
#26719=ORIENTED_EDGE('',*,*,#18644,.T.);
#26720=ORIENTED_EDGE('',*,*,#18649,.T.);
#26721=ORIENTED_EDGE('',*,*,#18650,.F.);
#26722=ORIENTED_EDGE('',*,*,#18651,.T.);
#26723=ORIENTED_EDGE('',*,*,#18647,.T.);
#26724=ORIENTED_EDGE('',*,*,#18652,.T.);
#26725=ORIENTED_EDGE('',*,*,#18653,.F.);
#26726=ORIENTED_EDGE('',*,*,#18654,.T.);
#26727=ORIENTED_EDGE('',*,*,#18650,.T.);
#26728=ORIENTED_EDGE('',*,*,#18655,.T.);
#26729=ORIENTED_EDGE('',*,*,#18656,.F.);
#26730=ORIENTED_EDGE('',*,*,#18657,.T.);
#26731=ORIENTED_EDGE('',*,*,#18653,.T.);
#26732=ORIENTED_EDGE('',*,*,#18658,.T.);
#26733=ORIENTED_EDGE('',*,*,#18659,.F.);
#26734=ORIENTED_EDGE('',*,*,#18660,.T.);
#26735=ORIENTED_EDGE('',*,*,#18656,.T.);
#26736=ORIENTED_EDGE('',*,*,#18661,.T.);
#26737=ORIENTED_EDGE('',*,*,#18662,.F.);
#26738=ORIENTED_EDGE('',*,*,#18663,.T.);
#26739=ORIENTED_EDGE('',*,*,#18659,.T.);
#26740=ORIENTED_EDGE('',*,*,#18664,.T.);
#26741=ORIENTED_EDGE('',*,*,#18665,.F.);
#26742=ORIENTED_EDGE('',*,*,#18666,.T.);
#26743=ORIENTED_EDGE('',*,*,#18662,.T.);
#26744=ORIENTED_EDGE('',*,*,#18667,.T.);
#26745=ORIENTED_EDGE('',*,*,#18668,.F.);
#26746=ORIENTED_EDGE('',*,*,#18669,.T.);
#26747=ORIENTED_EDGE('',*,*,#18665,.T.);
#26748=ORIENTED_EDGE('',*,*,#18670,.T.);
#26749=ORIENTED_EDGE('',*,*,#18671,.F.);
#26750=ORIENTED_EDGE('',*,*,#18672,.T.);
#26751=ORIENTED_EDGE('',*,*,#18668,.T.);
#26752=ORIENTED_EDGE('',*,*,#18673,.T.);
#26753=ORIENTED_EDGE('',*,*,#18674,.F.);
#26754=ORIENTED_EDGE('',*,*,#18675,.T.);
#26755=ORIENTED_EDGE('',*,*,#18676,.F.);
#26756=ORIENTED_EDGE('',*,*,#18677,.F.);
#26757=ORIENTED_EDGE('',*,*,#18678,.F.);
#26758=ORIENTED_EDGE('',*,*,#18679,.T.);
#26759=ORIENTED_EDGE('',*,*,#18674,.T.);
#26760=ORIENTED_EDGE('',*,*,#18680,.F.);
#26761=ORIENTED_EDGE('',*,*,#18681,.F.);
#26762=ORIENTED_EDGE('',*,*,#18682,.T.);
#26763=ORIENTED_EDGE('',*,*,#18678,.T.);
#26764=ORIENTED_EDGE('',*,*,#18683,.F.);
#26765=ORIENTED_EDGE('',*,*,#18684,.F.);
#26766=ORIENTED_EDGE('',*,*,#18685,.T.);
#26767=ORIENTED_EDGE('',*,*,#18681,.T.);
#26768=ORIENTED_EDGE('',*,*,#18686,.F.);
#26769=ORIENTED_EDGE('',*,*,#18687,.F.);
#26770=ORIENTED_EDGE('',*,*,#18688,.T.);
#26771=ORIENTED_EDGE('',*,*,#18684,.T.);
#26772=ORIENTED_EDGE('',*,*,#18689,.F.);
#26773=ORIENTED_EDGE('',*,*,#18690,.F.);
#26774=ORIENTED_EDGE('',*,*,#18691,.T.);
#26775=ORIENTED_EDGE('',*,*,#18687,.T.);
#26776=ORIENTED_EDGE('',*,*,#18692,.F.);
#26777=ORIENTED_EDGE('',*,*,#18693,.F.);
#26778=ORIENTED_EDGE('',*,*,#18694,.T.);
#26779=ORIENTED_EDGE('',*,*,#18690,.T.);
#26780=ORIENTED_EDGE('',*,*,#18695,.F.);
#26781=ORIENTED_EDGE('',*,*,#18696,.F.);
#26782=ORIENTED_EDGE('',*,*,#18697,.T.);
#26783=ORIENTED_EDGE('',*,*,#18693,.T.);
#26784=ORIENTED_EDGE('',*,*,#18698,.F.);
#26785=ORIENTED_EDGE('',*,*,#18699,.F.);
#26786=ORIENTED_EDGE('',*,*,#18700,.T.);
#26787=ORIENTED_EDGE('',*,*,#18696,.T.);
#26788=ORIENTED_EDGE('',*,*,#18701,.F.);
#26789=ORIENTED_EDGE('',*,*,#18702,.F.);
#26790=ORIENTED_EDGE('',*,*,#18703,.T.);
#26791=ORIENTED_EDGE('',*,*,#18699,.T.);
#26792=ORIENTED_EDGE('',*,*,#18704,.F.);
#26793=ORIENTED_EDGE('',*,*,#18705,.F.);
#26794=ORIENTED_EDGE('',*,*,#18706,.T.);
#26795=ORIENTED_EDGE('',*,*,#18702,.T.);
#26796=ORIENTED_EDGE('',*,*,#18707,.F.);
#26797=ORIENTED_EDGE('',*,*,#18708,.F.);
#26798=ORIENTED_EDGE('',*,*,#18709,.T.);
#26799=ORIENTED_EDGE('',*,*,#18705,.T.);
#26800=ORIENTED_EDGE('',*,*,#18710,.F.);
#26801=ORIENTED_EDGE('',*,*,#18711,.F.);
#26802=ORIENTED_EDGE('',*,*,#18712,.T.);
#26803=ORIENTED_EDGE('',*,*,#18708,.T.);
#26804=ORIENTED_EDGE('',*,*,#18713,.F.);
#26805=ORIENTED_EDGE('',*,*,#18714,.F.);
#26806=ORIENTED_EDGE('',*,*,#18715,.T.);
#26807=ORIENTED_EDGE('',*,*,#18711,.T.);
#26808=ORIENTED_EDGE('',*,*,#18716,.F.);
#26809=ORIENTED_EDGE('',*,*,#18717,.F.);
#26810=ORIENTED_EDGE('',*,*,#18718,.T.);
#26811=ORIENTED_EDGE('',*,*,#18714,.T.);
#26812=ORIENTED_EDGE('',*,*,#18719,.F.);
#26813=ORIENTED_EDGE('',*,*,#18720,.F.);
#26814=ORIENTED_EDGE('',*,*,#18721,.T.);
#26815=ORIENTED_EDGE('',*,*,#18717,.T.);
#26816=ORIENTED_EDGE('',*,*,#18722,.F.);
#26817=ORIENTED_EDGE('',*,*,#18723,.F.);
#26818=ORIENTED_EDGE('',*,*,#18724,.T.);
#26819=ORIENTED_EDGE('',*,*,#18720,.T.);
#26820=ORIENTED_EDGE('',*,*,#18725,.F.);
#26821=ORIENTED_EDGE('',*,*,#18726,.F.);
#26822=ORIENTED_EDGE('',*,*,#18727,.T.);
#26823=ORIENTED_EDGE('',*,*,#18723,.T.);
#26824=ORIENTED_EDGE('',*,*,#18728,.F.);
#26825=ORIENTED_EDGE('',*,*,#18729,.F.);
#26826=ORIENTED_EDGE('',*,*,#18730,.T.);
#26827=ORIENTED_EDGE('',*,*,#18726,.T.);
#26828=ORIENTED_EDGE('',*,*,#18731,.F.);
#26829=ORIENTED_EDGE('',*,*,#18732,.F.);
#26830=ORIENTED_EDGE('',*,*,#18733,.T.);
#26831=ORIENTED_EDGE('',*,*,#18729,.T.);
#26832=ORIENTED_EDGE('',*,*,#18734,.F.);
#26833=ORIENTED_EDGE('',*,*,#18735,.F.);
#26834=ORIENTED_EDGE('',*,*,#18736,.T.);
#26835=ORIENTED_EDGE('',*,*,#18732,.T.);
#26836=ORIENTED_EDGE('',*,*,#18737,.F.);
#26837=ORIENTED_EDGE('',*,*,#18738,.F.);
#26838=ORIENTED_EDGE('',*,*,#18739,.T.);
#26839=ORIENTED_EDGE('',*,*,#18735,.T.);
#26840=ORIENTED_EDGE('',*,*,#18740,.F.);
#26841=ORIENTED_EDGE('',*,*,#18741,.F.);
#26842=ORIENTED_EDGE('',*,*,#18742,.T.);
#26843=ORIENTED_EDGE('',*,*,#18738,.T.);
#26844=ORIENTED_EDGE('',*,*,#18743,.F.);
#26845=ORIENTED_EDGE('',*,*,#18744,.F.);
#26846=ORIENTED_EDGE('',*,*,#18745,.T.);
#26847=ORIENTED_EDGE('',*,*,#18741,.T.);
#26848=ORIENTED_EDGE('',*,*,#18746,.F.);
#26849=ORIENTED_EDGE('',*,*,#18747,.F.);
#26850=ORIENTED_EDGE('',*,*,#18748,.T.);
#26851=ORIENTED_EDGE('',*,*,#18744,.T.);
#26852=ORIENTED_EDGE('',*,*,#18749,.F.);
#26853=ORIENTED_EDGE('',*,*,#18750,.F.);
#26854=ORIENTED_EDGE('',*,*,#18751,.T.);
#26855=ORIENTED_EDGE('',*,*,#18747,.T.);
#26856=ORIENTED_EDGE('',*,*,#18752,.F.);
#26857=ORIENTED_EDGE('',*,*,#18753,.F.);
#26858=ORIENTED_EDGE('',*,*,#18754,.T.);
#26859=ORIENTED_EDGE('',*,*,#18750,.T.);
#26860=ORIENTED_EDGE('',*,*,#18755,.F.);
#26861=ORIENTED_EDGE('',*,*,#18756,.F.);
#26862=ORIENTED_EDGE('',*,*,#18757,.T.);
#26863=ORIENTED_EDGE('',*,*,#18753,.T.);
#26864=ORIENTED_EDGE('',*,*,#18758,.F.);
#26865=ORIENTED_EDGE('',*,*,#18759,.F.);
#26866=ORIENTED_EDGE('',*,*,#18760,.T.);
#26867=ORIENTED_EDGE('',*,*,#18756,.T.);
#26868=ORIENTED_EDGE('',*,*,#18761,.F.);
#26869=ORIENTED_EDGE('',*,*,#18762,.F.);
#26870=ORIENTED_EDGE('',*,*,#18763,.T.);
#26871=ORIENTED_EDGE('',*,*,#18759,.T.);
#26872=ORIENTED_EDGE('',*,*,#18764,.F.);
#26873=ORIENTED_EDGE('',*,*,#18765,.F.);
#26874=ORIENTED_EDGE('',*,*,#18766,.T.);
#26875=ORIENTED_EDGE('',*,*,#18762,.T.);
#26876=ORIENTED_EDGE('',*,*,#18767,.F.);
#26877=ORIENTED_EDGE('',*,*,#18768,.F.);
#26878=ORIENTED_EDGE('',*,*,#18769,.T.);
#26879=ORIENTED_EDGE('',*,*,#18765,.T.);
#26880=ORIENTED_EDGE('',*,*,#18770,.F.);
#26881=ORIENTED_EDGE('',*,*,#18771,.F.);
#26882=ORIENTED_EDGE('',*,*,#18772,.T.);
#26883=ORIENTED_EDGE('',*,*,#18768,.T.);
#26884=ORIENTED_EDGE('',*,*,#18773,.F.);
#26885=ORIENTED_EDGE('',*,*,#18774,.F.);
#26886=ORIENTED_EDGE('',*,*,#18775,.T.);
#26887=ORIENTED_EDGE('',*,*,#18771,.T.);
#26888=ORIENTED_EDGE('',*,*,#18776,.F.);
#26889=ORIENTED_EDGE('',*,*,#18777,.F.);
#26890=ORIENTED_EDGE('',*,*,#18778,.T.);
#26891=ORIENTED_EDGE('',*,*,#18774,.T.);
#26892=ORIENTED_EDGE('',*,*,#18779,.F.);
#26893=ORIENTED_EDGE('',*,*,#18780,.F.);
#26894=ORIENTED_EDGE('',*,*,#18781,.T.);
#26895=ORIENTED_EDGE('',*,*,#18777,.T.);
#26896=ORIENTED_EDGE('',*,*,#18782,.F.);
#26897=ORIENTED_EDGE('',*,*,#18783,.F.);
#26898=ORIENTED_EDGE('',*,*,#18784,.T.);
#26899=ORIENTED_EDGE('',*,*,#18780,.T.);
#26900=ORIENTED_EDGE('',*,*,#18785,.F.);
#26901=ORIENTED_EDGE('',*,*,#18786,.F.);
#26902=ORIENTED_EDGE('',*,*,#18787,.T.);
#26903=ORIENTED_EDGE('',*,*,#18783,.T.);
#26904=ORIENTED_EDGE('',*,*,#18788,.F.);
#26905=ORIENTED_EDGE('',*,*,#18789,.F.);
#26906=ORIENTED_EDGE('',*,*,#18790,.T.);
#26907=ORIENTED_EDGE('',*,*,#18786,.T.);
#26908=ORIENTED_EDGE('',*,*,#18791,.F.);
#26909=ORIENTED_EDGE('',*,*,#18792,.F.);
#26910=ORIENTED_EDGE('',*,*,#18793,.T.);
#26911=ORIENTED_EDGE('',*,*,#18789,.T.);
#26912=ORIENTED_EDGE('',*,*,#18794,.F.);
#26913=ORIENTED_EDGE('',*,*,#18795,.F.);
#26914=ORIENTED_EDGE('',*,*,#18796,.T.);
#26915=ORIENTED_EDGE('',*,*,#18792,.T.);
#26916=ORIENTED_EDGE('',*,*,#18797,.F.);
#26917=ORIENTED_EDGE('',*,*,#18798,.F.);
#26918=ORIENTED_EDGE('',*,*,#18799,.T.);
#26919=ORIENTED_EDGE('',*,*,#18795,.T.);
#26920=ORIENTED_EDGE('',*,*,#18800,.F.);
#26921=ORIENTED_EDGE('',*,*,#18801,.F.);
#26922=ORIENTED_EDGE('',*,*,#18802,.T.);
#26923=ORIENTED_EDGE('',*,*,#18798,.T.);
#26924=ORIENTED_EDGE('',*,*,#18803,.F.);
#26925=ORIENTED_EDGE('',*,*,#18804,.F.);
#26926=ORIENTED_EDGE('',*,*,#18805,.T.);
#26927=ORIENTED_EDGE('',*,*,#18801,.T.);
#26928=ORIENTED_EDGE('',*,*,#18806,.F.);
#26929=ORIENTED_EDGE('',*,*,#18807,.F.);
#26930=ORIENTED_EDGE('',*,*,#18808,.T.);
#26931=ORIENTED_EDGE('',*,*,#18804,.T.);
#26932=ORIENTED_EDGE('',*,*,#18809,.F.);
#26933=ORIENTED_EDGE('',*,*,#18810,.F.);
#26934=ORIENTED_EDGE('',*,*,#18811,.T.);
#26935=ORIENTED_EDGE('',*,*,#18807,.T.);
#26936=ORIENTED_EDGE('',*,*,#18812,.F.);
#26937=ORIENTED_EDGE('',*,*,#18813,.F.);
#26938=ORIENTED_EDGE('',*,*,#18814,.T.);
#26939=ORIENTED_EDGE('',*,*,#18810,.T.);
#26940=ORIENTED_EDGE('',*,*,#18815,.F.);
#26941=ORIENTED_EDGE('',*,*,#18816,.F.);
#26942=ORIENTED_EDGE('',*,*,#18817,.T.);
#26943=ORIENTED_EDGE('',*,*,#18813,.T.);
#26944=ORIENTED_EDGE('',*,*,#18818,.F.);
#26945=ORIENTED_EDGE('',*,*,#18819,.F.);
#26946=ORIENTED_EDGE('',*,*,#18820,.T.);
#26947=ORIENTED_EDGE('',*,*,#18816,.T.);
#26948=ORIENTED_EDGE('',*,*,#18821,.F.);
#26949=ORIENTED_EDGE('',*,*,#18822,.F.);
#26950=ORIENTED_EDGE('',*,*,#18823,.T.);
#26951=ORIENTED_EDGE('',*,*,#18819,.T.);
#26952=ORIENTED_EDGE('',*,*,#18824,.F.);
#26953=ORIENTED_EDGE('',*,*,#18825,.F.);
#26954=ORIENTED_EDGE('',*,*,#18826,.T.);
#26955=ORIENTED_EDGE('',*,*,#18822,.T.);
#26956=ORIENTED_EDGE('',*,*,#18827,.F.);
#26957=ORIENTED_EDGE('',*,*,#18828,.F.);
#26958=ORIENTED_EDGE('',*,*,#18829,.T.);
#26959=ORIENTED_EDGE('',*,*,#18825,.T.);
#26960=ORIENTED_EDGE('',*,*,#18830,.F.);
#26961=ORIENTED_EDGE('',*,*,#18831,.F.);
#26962=ORIENTED_EDGE('',*,*,#18832,.T.);
#26963=ORIENTED_EDGE('',*,*,#18828,.T.);
#26964=ORIENTED_EDGE('',*,*,#18833,.F.);
#26965=ORIENTED_EDGE('',*,*,#18834,.F.);
#26966=ORIENTED_EDGE('',*,*,#18835,.T.);
#26967=ORIENTED_EDGE('',*,*,#18831,.T.);
#26968=ORIENTED_EDGE('',*,*,#18836,.F.);
#26969=ORIENTED_EDGE('',*,*,#18837,.F.);
#26970=ORIENTED_EDGE('',*,*,#18838,.T.);
#26971=ORIENTED_EDGE('',*,*,#18834,.T.);
#26972=ORIENTED_EDGE('',*,*,#18839,.F.);
#26973=ORIENTED_EDGE('',*,*,#18840,.F.);
#26974=ORIENTED_EDGE('',*,*,#18841,.T.);
#26975=ORIENTED_EDGE('',*,*,#18837,.T.);
#26976=ORIENTED_EDGE('',*,*,#18842,.F.);
#26977=ORIENTED_EDGE('',*,*,#18843,.F.);
#26978=ORIENTED_EDGE('',*,*,#18844,.T.);
#26979=ORIENTED_EDGE('',*,*,#18840,.T.);
#26980=ORIENTED_EDGE('',*,*,#18845,.F.);
#26981=ORIENTED_EDGE('',*,*,#18846,.F.);
#26982=ORIENTED_EDGE('',*,*,#18847,.T.);
#26983=ORIENTED_EDGE('',*,*,#18843,.T.);
#26984=ORIENTED_EDGE('',*,*,#18848,.F.);
#26985=ORIENTED_EDGE('',*,*,#18849,.F.);
#26986=ORIENTED_EDGE('',*,*,#18850,.T.);
#26987=ORIENTED_EDGE('',*,*,#18846,.T.);
#26988=ORIENTED_EDGE('',*,*,#18851,.F.);
#26989=ORIENTED_EDGE('',*,*,#18852,.F.);
#26990=ORIENTED_EDGE('',*,*,#18853,.T.);
#26991=ORIENTED_EDGE('',*,*,#18849,.T.);
#26992=ORIENTED_EDGE('',*,*,#18854,.F.);
#26993=ORIENTED_EDGE('',*,*,#18855,.F.);
#26994=ORIENTED_EDGE('',*,*,#18856,.T.);
#26995=ORIENTED_EDGE('',*,*,#18852,.T.);
#26996=ORIENTED_EDGE('',*,*,#18857,.F.);
#26997=ORIENTED_EDGE('',*,*,#18858,.F.);
#26998=ORIENTED_EDGE('',*,*,#18859,.T.);
#26999=ORIENTED_EDGE('',*,*,#18855,.T.);
#27000=ORIENTED_EDGE('',*,*,#18860,.F.);
#27001=ORIENTED_EDGE('',*,*,#18861,.F.);
#27002=ORIENTED_EDGE('',*,*,#18862,.T.);
#27003=ORIENTED_EDGE('',*,*,#18858,.T.);
#27004=ORIENTED_EDGE('',*,*,#18863,.F.);
#27005=ORIENTED_EDGE('',*,*,#18864,.F.);
#27006=ORIENTED_EDGE('',*,*,#18865,.T.);
#27007=ORIENTED_EDGE('',*,*,#18861,.T.);
#27008=ORIENTED_EDGE('',*,*,#18866,.F.);
#27009=ORIENTED_EDGE('',*,*,#18867,.F.);
#27010=ORIENTED_EDGE('',*,*,#18868,.T.);
#27011=ORIENTED_EDGE('',*,*,#18864,.T.);
#27012=ORIENTED_EDGE('',*,*,#18869,.F.);
#27013=ORIENTED_EDGE('',*,*,#18870,.F.);
#27014=ORIENTED_EDGE('',*,*,#18871,.T.);
#27015=ORIENTED_EDGE('',*,*,#18867,.T.);
#27016=ORIENTED_EDGE('',*,*,#18872,.F.);
#27017=ORIENTED_EDGE('',*,*,#18873,.F.);
#27018=ORIENTED_EDGE('',*,*,#18874,.T.);
#27019=ORIENTED_EDGE('',*,*,#18870,.T.);
#27020=ORIENTED_EDGE('',*,*,#18875,.F.);
#27021=ORIENTED_EDGE('',*,*,#18876,.F.);
#27022=ORIENTED_EDGE('',*,*,#18877,.T.);
#27023=ORIENTED_EDGE('',*,*,#18873,.T.);
#27024=ORIENTED_EDGE('',*,*,#18878,.F.);
#27025=ORIENTED_EDGE('',*,*,#18879,.F.);
#27026=ORIENTED_EDGE('',*,*,#18880,.T.);
#27027=ORIENTED_EDGE('',*,*,#18876,.T.);
#27028=ORIENTED_EDGE('',*,*,#18881,.F.);
#27029=ORIENTED_EDGE('',*,*,#18882,.F.);
#27030=ORIENTED_EDGE('',*,*,#18883,.T.);
#27031=ORIENTED_EDGE('',*,*,#18879,.T.);
#27032=ORIENTED_EDGE('',*,*,#18884,.F.);
#27033=ORIENTED_EDGE('',*,*,#18885,.F.);
#27034=ORIENTED_EDGE('',*,*,#18886,.T.);
#27035=ORIENTED_EDGE('',*,*,#18882,.T.);
#27036=ORIENTED_EDGE('',*,*,#18887,.F.);
#27037=ORIENTED_EDGE('',*,*,#18888,.F.);
#27038=ORIENTED_EDGE('',*,*,#18889,.T.);
#27039=ORIENTED_EDGE('',*,*,#18885,.T.);
#27040=ORIENTED_EDGE('',*,*,#18890,.F.);
#27041=ORIENTED_EDGE('',*,*,#18891,.F.);
#27042=ORIENTED_EDGE('',*,*,#18892,.T.);
#27043=ORIENTED_EDGE('',*,*,#18888,.T.);
#27044=ORIENTED_EDGE('',*,*,#18893,.F.);
#27045=ORIENTED_EDGE('',*,*,#18894,.F.);
#27046=ORIENTED_EDGE('',*,*,#18895,.T.);
#27047=ORIENTED_EDGE('',*,*,#18891,.T.);
#27048=ORIENTED_EDGE('',*,*,#18896,.F.);
#27049=ORIENTED_EDGE('',*,*,#18897,.F.);
#27050=ORIENTED_EDGE('',*,*,#18898,.T.);
#27051=ORIENTED_EDGE('',*,*,#18894,.T.);
#27052=ORIENTED_EDGE('',*,*,#18899,.F.);
#27053=ORIENTED_EDGE('',*,*,#18676,.T.);
#27054=ORIENTED_EDGE('',*,*,#18900,.T.);
#27055=ORIENTED_EDGE('',*,*,#18901,.F.);
#27056=ORIENTED_EDGE('',*,*,#18902,.F.);
#27057=ORIENTED_EDGE('',*,*,#18903,.T.);
#27058=ORIENTED_EDGE('',*,*,#18903,.F.);
#27059=ORIENTED_EDGE('',*,*,#18904,.F.);
#27060=ORIENTED_EDGE('',*,*,#18673,.F.);
#27061=ORIENTED_EDGE('',*,*,#18670,.F.);
#27062=ORIENTED_EDGE('',*,*,#18667,.F.);
#27063=ORIENTED_EDGE('',*,*,#18664,.F.);
#27064=ORIENTED_EDGE('',*,*,#18661,.F.);
#27065=ORIENTED_EDGE('',*,*,#18658,.F.);
#27066=ORIENTED_EDGE('',*,*,#18655,.F.);
#27067=ORIENTED_EDGE('',*,*,#18652,.F.);
#27068=ORIENTED_EDGE('',*,*,#18649,.F.);
#27069=ORIENTED_EDGE('',*,*,#18646,.F.);
#27070=ORIENTED_EDGE('',*,*,#18643,.F.);
#27071=ORIENTED_EDGE('',*,*,#18640,.F.);
#27072=ORIENTED_EDGE('',*,*,#18637,.F.);
#27073=ORIENTED_EDGE('',*,*,#18634,.F.);
#27074=ORIENTED_EDGE('',*,*,#18631,.F.);
#27075=ORIENTED_EDGE('',*,*,#18628,.F.);
#27076=ORIENTED_EDGE('',*,*,#18625,.F.);
#27077=ORIENTED_EDGE('',*,*,#18622,.F.);
#27078=ORIENTED_EDGE('',*,*,#18619,.F.);
#27079=ORIENTED_EDGE('',*,*,#18616,.F.);
#27080=ORIENTED_EDGE('',*,*,#18613,.F.);
#27081=ORIENTED_EDGE('',*,*,#18610,.F.);
#27082=ORIENTED_EDGE('',*,*,#18607,.F.);
#27083=ORIENTED_EDGE('',*,*,#18604,.F.);
#27084=ORIENTED_EDGE('',*,*,#18601,.F.);
#27085=ORIENTED_EDGE('',*,*,#18598,.F.);
#27086=ORIENTED_EDGE('',*,*,#18595,.F.);
#27087=ORIENTED_EDGE('',*,*,#18592,.F.);
#27088=ORIENTED_EDGE('',*,*,#18589,.F.);
#27089=ORIENTED_EDGE('',*,*,#18586,.F.);
#27090=ORIENTED_EDGE('',*,*,#18583,.F.);
#27091=ORIENTED_EDGE('',*,*,#18580,.F.);
#27092=ORIENTED_EDGE('',*,*,#18577,.F.);
#27093=ORIENTED_EDGE('',*,*,#18574,.F.);
#27094=ORIENTED_EDGE('',*,*,#18571,.F.);
#27095=ORIENTED_EDGE('',*,*,#18568,.F.);
#27096=ORIENTED_EDGE('',*,*,#18565,.F.);
#27097=ORIENTED_EDGE('',*,*,#18562,.F.);
#27098=ORIENTED_EDGE('',*,*,#18559,.F.);
#27099=ORIENTED_EDGE('',*,*,#18556,.F.);
#27100=ORIENTED_EDGE('',*,*,#18553,.F.);
#27101=ORIENTED_EDGE('',*,*,#18550,.F.);
#27102=ORIENTED_EDGE('',*,*,#18547,.F.);
#27103=ORIENTED_EDGE('',*,*,#18544,.F.);
#27104=ORIENTED_EDGE('',*,*,#18541,.F.);
#27105=ORIENTED_EDGE('',*,*,#18538,.F.);
#27106=ORIENTED_EDGE('',*,*,#18535,.F.);
#27107=ORIENTED_EDGE('',*,*,#18532,.F.);
#27108=ORIENTED_EDGE('',*,*,#18529,.F.);
#27109=ORIENTED_EDGE('',*,*,#18526,.F.);
#27110=ORIENTED_EDGE('',*,*,#18523,.F.);
#27111=ORIENTED_EDGE('',*,*,#18520,.F.);
#27112=ORIENTED_EDGE('',*,*,#18517,.F.);
#27113=ORIENTED_EDGE('',*,*,#18514,.F.);
#27114=ORIENTED_EDGE('',*,*,#18511,.F.);
#27115=ORIENTED_EDGE('',*,*,#18508,.F.);
#27116=ORIENTED_EDGE('',*,*,#18505,.F.);
#27117=ORIENTED_EDGE('',*,*,#18502,.F.);
#27118=ORIENTED_EDGE('',*,*,#18499,.F.);
#27119=ORIENTED_EDGE('',*,*,#18496,.F.);
#27120=ORIENTED_EDGE('',*,*,#18493,.F.);
#27121=ORIENTED_EDGE('',*,*,#18490,.F.);
#27122=ORIENTED_EDGE('',*,*,#18487,.F.);
#27123=ORIENTED_EDGE('',*,*,#18484,.F.);
#27124=ORIENTED_EDGE('',*,*,#18481,.F.);
#27125=ORIENTED_EDGE('',*,*,#18478,.F.);
#27126=ORIENTED_EDGE('',*,*,#18475,.F.);
#27127=ORIENTED_EDGE('',*,*,#18472,.F.);
#27128=ORIENTED_EDGE('',*,*,#18469,.F.);
#27129=ORIENTED_EDGE('',*,*,#18466,.F.);
#27130=ORIENTED_EDGE('',*,*,#18463,.F.);
#27131=ORIENTED_EDGE('',*,*,#18460,.F.);
#27132=ORIENTED_EDGE('',*,*,#18457,.F.);
#27133=ORIENTED_EDGE('',*,*,#18454,.F.);
#27134=ORIENTED_EDGE('',*,*,#18451,.F.);
#27135=ORIENTED_EDGE('',*,*,#18905,.F.);
#27136=ORIENTED_EDGE('',*,*,#18906,.T.);
#27137=ORIENTED_EDGE('',*,*,#18899,.T.);
#27138=ORIENTED_EDGE('',*,*,#18896,.T.);
#27139=ORIENTED_EDGE('',*,*,#18893,.T.);
#27140=ORIENTED_EDGE('',*,*,#18890,.T.);
#27141=ORIENTED_EDGE('',*,*,#18887,.T.);
#27142=ORIENTED_EDGE('',*,*,#18884,.T.);
#27143=ORIENTED_EDGE('',*,*,#18881,.T.);
#27144=ORIENTED_EDGE('',*,*,#18878,.T.);
#27145=ORIENTED_EDGE('',*,*,#18875,.T.);
#27146=ORIENTED_EDGE('',*,*,#18872,.T.);
#27147=ORIENTED_EDGE('',*,*,#18869,.T.);
#27148=ORIENTED_EDGE('',*,*,#18866,.T.);
#27149=ORIENTED_EDGE('',*,*,#18863,.T.);
#27150=ORIENTED_EDGE('',*,*,#18860,.T.);
#27151=ORIENTED_EDGE('',*,*,#18857,.T.);
#27152=ORIENTED_EDGE('',*,*,#18854,.T.);
#27153=ORIENTED_EDGE('',*,*,#18851,.T.);
#27154=ORIENTED_EDGE('',*,*,#18848,.T.);
#27155=ORIENTED_EDGE('',*,*,#18845,.T.);
#27156=ORIENTED_EDGE('',*,*,#18842,.T.);
#27157=ORIENTED_EDGE('',*,*,#18839,.T.);
#27158=ORIENTED_EDGE('',*,*,#18836,.T.);
#27159=ORIENTED_EDGE('',*,*,#18833,.T.);
#27160=ORIENTED_EDGE('',*,*,#18830,.T.);
#27161=ORIENTED_EDGE('',*,*,#18827,.T.);
#27162=ORIENTED_EDGE('',*,*,#18824,.T.);
#27163=ORIENTED_EDGE('',*,*,#18821,.T.);
#27164=ORIENTED_EDGE('',*,*,#18818,.T.);
#27165=ORIENTED_EDGE('',*,*,#18815,.T.);
#27166=ORIENTED_EDGE('',*,*,#18812,.T.);
#27167=ORIENTED_EDGE('',*,*,#18809,.T.);
#27168=ORIENTED_EDGE('',*,*,#18806,.T.);
#27169=ORIENTED_EDGE('',*,*,#18803,.T.);
#27170=ORIENTED_EDGE('',*,*,#18800,.T.);
#27171=ORIENTED_EDGE('',*,*,#18797,.T.);
#27172=ORIENTED_EDGE('',*,*,#18794,.T.);
#27173=ORIENTED_EDGE('',*,*,#18791,.T.);
#27174=ORIENTED_EDGE('',*,*,#18788,.T.);
#27175=ORIENTED_EDGE('',*,*,#18785,.T.);
#27176=ORIENTED_EDGE('',*,*,#18782,.T.);
#27177=ORIENTED_EDGE('',*,*,#18779,.T.);
#27178=ORIENTED_EDGE('',*,*,#18776,.T.);
#27179=ORIENTED_EDGE('',*,*,#18773,.T.);
#27180=ORIENTED_EDGE('',*,*,#18770,.T.);
#27181=ORIENTED_EDGE('',*,*,#18767,.T.);
#27182=ORIENTED_EDGE('',*,*,#18764,.T.);
#27183=ORIENTED_EDGE('',*,*,#18761,.T.);
#27184=ORIENTED_EDGE('',*,*,#18758,.T.);
#27185=ORIENTED_EDGE('',*,*,#18755,.T.);
#27186=ORIENTED_EDGE('',*,*,#18752,.T.);
#27187=ORIENTED_EDGE('',*,*,#18749,.T.);
#27188=ORIENTED_EDGE('',*,*,#18746,.T.);
#27189=ORIENTED_EDGE('',*,*,#18743,.T.);
#27190=ORIENTED_EDGE('',*,*,#18740,.T.);
#27191=ORIENTED_EDGE('',*,*,#18737,.T.);
#27192=ORIENTED_EDGE('',*,*,#18734,.T.);
#27193=ORIENTED_EDGE('',*,*,#18731,.T.);
#27194=ORIENTED_EDGE('',*,*,#18728,.T.);
#27195=ORIENTED_EDGE('',*,*,#18725,.T.);
#27196=ORIENTED_EDGE('',*,*,#18722,.T.);
#27197=ORIENTED_EDGE('',*,*,#18719,.T.);
#27198=ORIENTED_EDGE('',*,*,#18716,.T.);
#27199=ORIENTED_EDGE('',*,*,#18713,.T.);
#27200=ORIENTED_EDGE('',*,*,#18710,.T.);
#27201=ORIENTED_EDGE('',*,*,#18707,.T.);
#27202=ORIENTED_EDGE('',*,*,#18704,.T.);
#27203=ORIENTED_EDGE('',*,*,#18701,.T.);
#27204=ORIENTED_EDGE('',*,*,#18698,.T.);
#27205=ORIENTED_EDGE('',*,*,#18695,.T.);
#27206=ORIENTED_EDGE('',*,*,#18692,.T.);
#27207=ORIENTED_EDGE('',*,*,#18689,.T.);
#27208=ORIENTED_EDGE('',*,*,#18686,.T.);
#27209=ORIENTED_EDGE('',*,*,#18683,.T.);
#27210=ORIENTED_EDGE('',*,*,#18680,.T.);
#27211=ORIENTED_EDGE('',*,*,#18677,.T.);
#27212=ORIENTED_EDGE('',*,*,#18907,.T.);
#27213=ORIENTED_EDGE('',*,*,#18908,.T.);
#27214=ORIENTED_EDGE('',*,*,#18909,.T.);
#27215=ORIENTED_EDGE('',*,*,#18910,.T.);
#27216=ORIENTED_EDGE('',*,*,#18905,.T.);
#27217=ORIENTED_EDGE('',*,*,#18897,.T.);
#27218=ORIENTED_EDGE('',*,*,#18906,.F.);
#27219=ORIENTED_EDGE('',*,*,#18910,.F.);
#27220=ORIENTED_EDGE('',*,*,#18911,.T.);
#27221=ORIENTED_EDGE('',*,*,#18900,.F.);
#27222=ORIENTED_EDGE('',*,*,#18675,.F.);
#27223=ORIENTED_EDGE('',*,*,#18679,.F.);
#27224=ORIENTED_EDGE('',*,*,#18682,.F.);
#27225=ORIENTED_EDGE('',*,*,#18685,.F.);
#27226=ORIENTED_EDGE('',*,*,#18688,.F.);
#27227=ORIENTED_EDGE('',*,*,#18691,.F.);
#27228=ORIENTED_EDGE('',*,*,#18694,.F.);
#27229=ORIENTED_EDGE('',*,*,#18697,.F.);
#27230=ORIENTED_EDGE('',*,*,#18700,.F.);
#27231=ORIENTED_EDGE('',*,*,#18703,.F.);
#27232=ORIENTED_EDGE('',*,*,#18706,.F.);
#27233=ORIENTED_EDGE('',*,*,#18709,.F.);
#27234=ORIENTED_EDGE('',*,*,#18712,.F.);
#27235=ORIENTED_EDGE('',*,*,#18715,.F.);
#27236=ORIENTED_EDGE('',*,*,#18718,.F.);
#27237=ORIENTED_EDGE('',*,*,#18721,.F.);
#27238=ORIENTED_EDGE('',*,*,#18724,.F.);
#27239=ORIENTED_EDGE('',*,*,#18727,.F.);
#27240=ORIENTED_EDGE('',*,*,#18730,.F.);
#27241=ORIENTED_EDGE('',*,*,#18733,.F.);
#27242=ORIENTED_EDGE('',*,*,#18736,.F.);
#27243=ORIENTED_EDGE('',*,*,#18739,.F.);
#27244=ORIENTED_EDGE('',*,*,#18742,.F.);
#27245=ORIENTED_EDGE('',*,*,#18745,.F.);
#27246=ORIENTED_EDGE('',*,*,#18748,.F.);
#27247=ORIENTED_EDGE('',*,*,#18751,.F.);
#27248=ORIENTED_EDGE('',*,*,#18754,.F.);
#27249=ORIENTED_EDGE('',*,*,#18757,.F.);
#27250=ORIENTED_EDGE('',*,*,#18760,.F.);
#27251=ORIENTED_EDGE('',*,*,#18763,.F.);
#27252=ORIENTED_EDGE('',*,*,#18766,.F.);
#27253=ORIENTED_EDGE('',*,*,#18769,.F.);
#27254=ORIENTED_EDGE('',*,*,#18772,.F.);
#27255=ORIENTED_EDGE('',*,*,#18775,.F.);
#27256=ORIENTED_EDGE('',*,*,#18778,.F.);
#27257=ORIENTED_EDGE('',*,*,#18781,.F.);
#27258=ORIENTED_EDGE('',*,*,#18784,.F.);
#27259=ORIENTED_EDGE('',*,*,#18787,.F.);
#27260=ORIENTED_EDGE('',*,*,#18790,.F.);
#27261=ORIENTED_EDGE('',*,*,#18793,.F.);
#27262=ORIENTED_EDGE('',*,*,#18796,.F.);
#27263=ORIENTED_EDGE('',*,*,#18799,.F.);
#27264=ORIENTED_EDGE('',*,*,#18802,.F.);
#27265=ORIENTED_EDGE('',*,*,#18805,.F.);
#27266=ORIENTED_EDGE('',*,*,#18808,.F.);
#27267=ORIENTED_EDGE('',*,*,#18811,.F.);
#27268=ORIENTED_EDGE('',*,*,#18814,.F.);
#27269=ORIENTED_EDGE('',*,*,#18817,.F.);
#27270=ORIENTED_EDGE('',*,*,#18820,.F.);
#27271=ORIENTED_EDGE('',*,*,#18823,.F.);
#27272=ORIENTED_EDGE('',*,*,#18826,.F.);
#27273=ORIENTED_EDGE('',*,*,#18829,.F.);
#27274=ORIENTED_EDGE('',*,*,#18832,.F.);
#27275=ORIENTED_EDGE('',*,*,#18835,.F.);
#27276=ORIENTED_EDGE('',*,*,#18838,.F.);
#27277=ORIENTED_EDGE('',*,*,#18841,.F.);
#27278=ORIENTED_EDGE('',*,*,#18844,.F.);
#27279=ORIENTED_EDGE('',*,*,#18847,.F.);
#27280=ORIENTED_EDGE('',*,*,#18850,.F.);
#27281=ORIENTED_EDGE('',*,*,#18853,.F.);
#27282=ORIENTED_EDGE('',*,*,#18856,.F.);
#27283=ORIENTED_EDGE('',*,*,#18859,.F.);
#27284=ORIENTED_EDGE('',*,*,#18862,.F.);
#27285=ORIENTED_EDGE('',*,*,#18865,.F.);
#27286=ORIENTED_EDGE('',*,*,#18868,.F.);
#27287=ORIENTED_EDGE('',*,*,#18871,.F.);
#27288=ORIENTED_EDGE('',*,*,#18874,.F.);
#27289=ORIENTED_EDGE('',*,*,#18877,.F.);
#27290=ORIENTED_EDGE('',*,*,#18880,.F.);
#27291=ORIENTED_EDGE('',*,*,#18883,.F.);
#27292=ORIENTED_EDGE('',*,*,#18886,.F.);
#27293=ORIENTED_EDGE('',*,*,#18889,.F.);
#27294=ORIENTED_EDGE('',*,*,#18892,.F.);
#27295=ORIENTED_EDGE('',*,*,#18895,.F.);
#27296=ORIENTED_EDGE('',*,*,#18898,.F.);
#27297=ORIENTED_EDGE('',*,*,#18911,.F.);
#27298=ORIENTED_EDGE('',*,*,#18909,.F.);
#27299=ORIENTED_EDGE('',*,*,#18449,.F.);
#27300=ORIENTED_EDGE('',*,*,#18453,.F.);
#27301=ORIENTED_EDGE('',*,*,#18456,.F.);
#27302=ORIENTED_EDGE('',*,*,#18459,.F.);
#27303=ORIENTED_EDGE('',*,*,#18462,.F.);
#27304=ORIENTED_EDGE('',*,*,#18465,.F.);
#27305=ORIENTED_EDGE('',*,*,#18468,.F.);
#27306=ORIENTED_EDGE('',*,*,#18471,.F.);
#27307=ORIENTED_EDGE('',*,*,#18474,.F.);
#27308=ORIENTED_EDGE('',*,*,#18477,.F.);
#27309=ORIENTED_EDGE('',*,*,#18480,.F.);
#27310=ORIENTED_EDGE('',*,*,#18483,.F.);
#27311=ORIENTED_EDGE('',*,*,#18486,.F.);
#27312=ORIENTED_EDGE('',*,*,#18489,.F.);
#27313=ORIENTED_EDGE('',*,*,#18492,.F.);
#27314=ORIENTED_EDGE('',*,*,#18495,.F.);
#27315=ORIENTED_EDGE('',*,*,#18498,.F.);
#27316=ORIENTED_EDGE('',*,*,#18501,.F.);
#27317=ORIENTED_EDGE('',*,*,#18504,.F.);
#27318=ORIENTED_EDGE('',*,*,#18507,.F.);
#27319=ORIENTED_EDGE('',*,*,#18510,.F.);
#27320=ORIENTED_EDGE('',*,*,#18513,.F.);
#27321=ORIENTED_EDGE('',*,*,#18516,.F.);
#27322=ORIENTED_EDGE('',*,*,#18519,.F.);
#27323=ORIENTED_EDGE('',*,*,#18522,.F.);
#27324=ORIENTED_EDGE('',*,*,#18525,.F.);
#27325=ORIENTED_EDGE('',*,*,#18528,.F.);
#27326=ORIENTED_EDGE('',*,*,#18531,.F.);
#27327=ORIENTED_EDGE('',*,*,#18534,.F.);
#27328=ORIENTED_EDGE('',*,*,#18537,.F.);
#27329=ORIENTED_EDGE('',*,*,#18540,.F.);
#27330=ORIENTED_EDGE('',*,*,#18543,.F.);
#27331=ORIENTED_EDGE('',*,*,#18546,.F.);
#27332=ORIENTED_EDGE('',*,*,#18549,.F.);
#27333=ORIENTED_EDGE('',*,*,#18552,.F.);
#27334=ORIENTED_EDGE('',*,*,#18555,.F.);
#27335=ORIENTED_EDGE('',*,*,#18558,.F.);
#27336=ORIENTED_EDGE('',*,*,#18561,.F.);
#27337=ORIENTED_EDGE('',*,*,#18564,.F.);
#27338=ORIENTED_EDGE('',*,*,#18567,.F.);
#27339=ORIENTED_EDGE('',*,*,#18570,.F.);
#27340=ORIENTED_EDGE('',*,*,#18573,.F.);
#27341=ORIENTED_EDGE('',*,*,#18576,.F.);
#27342=ORIENTED_EDGE('',*,*,#18579,.F.);
#27343=ORIENTED_EDGE('',*,*,#18582,.F.);
#27344=ORIENTED_EDGE('',*,*,#18585,.F.);
#27345=ORIENTED_EDGE('',*,*,#18588,.F.);
#27346=ORIENTED_EDGE('',*,*,#18591,.F.);
#27347=ORIENTED_EDGE('',*,*,#18594,.F.);
#27348=ORIENTED_EDGE('',*,*,#18597,.F.);
#27349=ORIENTED_EDGE('',*,*,#18600,.F.);
#27350=ORIENTED_EDGE('',*,*,#18603,.F.);
#27351=ORIENTED_EDGE('',*,*,#18606,.F.);
#27352=ORIENTED_EDGE('',*,*,#18609,.F.);
#27353=ORIENTED_EDGE('',*,*,#18612,.F.);
#27354=ORIENTED_EDGE('',*,*,#18615,.F.);
#27355=ORIENTED_EDGE('',*,*,#18618,.F.);
#27356=ORIENTED_EDGE('',*,*,#18621,.F.);
#27357=ORIENTED_EDGE('',*,*,#18624,.F.);
#27358=ORIENTED_EDGE('',*,*,#18627,.F.);
#27359=ORIENTED_EDGE('',*,*,#18630,.F.);
#27360=ORIENTED_EDGE('',*,*,#18633,.F.);
#27361=ORIENTED_EDGE('',*,*,#18636,.F.);
#27362=ORIENTED_EDGE('',*,*,#18639,.F.);
#27363=ORIENTED_EDGE('',*,*,#18642,.F.);
#27364=ORIENTED_EDGE('',*,*,#18645,.F.);
#27365=ORIENTED_EDGE('',*,*,#18648,.F.);
#27366=ORIENTED_EDGE('',*,*,#18651,.F.);
#27367=ORIENTED_EDGE('',*,*,#18654,.F.);
#27368=ORIENTED_EDGE('',*,*,#18657,.F.);
#27369=ORIENTED_EDGE('',*,*,#18660,.F.);
#27370=ORIENTED_EDGE('',*,*,#18663,.F.);
#27371=ORIENTED_EDGE('',*,*,#18666,.F.);
#27372=ORIENTED_EDGE('',*,*,#18669,.F.);
#27373=ORIENTED_EDGE('',*,*,#18672,.F.);
#27374=ORIENTED_EDGE('',*,*,#18912,.F.);
#27375=ORIENTED_EDGE('',*,*,#18913,.F.);
#27376=ORIENTED_EDGE('',*,*,#18914,.T.);
#27377=ORIENTED_EDGE('',*,*,#18915,.T.);
#27378=ORIENTED_EDGE('',*,*,#18914,.F.);
#27379=ORIENTED_EDGE('',*,*,#18907,.F.);
#27380=ORIENTED_EDGE('',*,*,#18450,.F.);
#27381=ORIENTED_EDGE('',*,*,#18908,.F.);
#27382=ORIENTED_EDGE('',*,*,#18916,.T.);
#27383=ORIENTED_EDGE('',*,*,#18913,.T.);
#27384=ORIENTED_EDGE('',*,*,#18916,.F.);
#27385=ORIENTED_EDGE('',*,*,#18671,.T.);
#27386=ORIENTED_EDGE('',*,*,#18904,.T.);
#27387=ORIENTED_EDGE('',*,*,#18917,.F.);
#27388=ORIENTED_EDGE('',*,*,#18912,.T.);
#27389=ORIENTED_EDGE('',*,*,#18918,.F.);
#27390=ORIENTED_EDGE('',*,*,#18919,.T.);
#27391=ORIENTED_EDGE('',*,*,#18901,.T.);
#27392=ORIENTED_EDGE('',*,*,#18917,.T.);
#27393=ORIENTED_EDGE('',*,*,#18902,.T.);
#27394=ORIENTED_EDGE('',*,*,#18919,.F.);
#27395=ORIENTED_EDGE('',*,*,#18918,.T.);
#27396=ORIENTED_EDGE('',*,*,#18920,.T.);
#27397=ORIENTED_EDGE('',*,*,#18920,.F.);
#27398=ORIENTED_EDGE('',*,*,#18915,.F.);
#28829=PLANE('',#33135);
#28830=PLANE('',#33138);
#28831=PLANE('',#33151);
#30372=ADVANCED_FACE('',(#5044),#850,.T.);
#30373=ADVANCED_FACE('',(#5045),#851,.T.);
#30374=ADVANCED_FACE('',(#5046),#852,.T.);
#30375=ADVANCED_FACE('',(#5047),#853,.T.);
#30376=ADVANCED_FACE('',(#5048),#854,.T.);
#30377=ADVANCED_FACE('',(#5049),#855,.T.);
#30378=ADVANCED_FACE('',(#5050),#856,.T.);
#30379=ADVANCED_FACE('',(#5051),#857,.T.);
#30380=ADVANCED_FACE('',(#5052),#858,.T.);
#30381=ADVANCED_FACE('',(#5053),#859,.T.);
#30382=ADVANCED_FACE('',(#5054),#860,.T.);
#30383=ADVANCED_FACE('',(#5055),#861,.T.);
#30384=ADVANCED_FACE('',(#5056),#862,.T.);
#30385=ADVANCED_FACE('',(#5057),#863,.T.);
#30386=ADVANCED_FACE('',(#5058),#864,.T.);
#30387=ADVANCED_FACE('',(#5059),#865,.T.);
#30388=ADVANCED_FACE('',(#5060),#866,.T.);
#30389=ADVANCED_FACE('',(#5061),#867,.T.);
#30390=ADVANCED_FACE('',(#5062),#868,.T.);
#30391=ADVANCED_FACE('',(#5063),#869,.T.);
#30392=ADVANCED_FACE('',(#5064),#870,.T.);
#30393=ADVANCED_FACE('',(#5065),#871,.T.);
#30394=ADVANCED_FACE('',(#5066),#872,.T.);
#30395=ADVANCED_FACE('',(#5067),#873,.T.);
#30396=ADVANCED_FACE('',(#5068),#874,.T.);
#30397=ADVANCED_FACE('',(#5069),#875,.T.);
#30398=ADVANCED_FACE('',(#5070),#876,.T.);
#30399=ADVANCED_FACE('',(#5071),#877,.T.);
#30400=ADVANCED_FACE('',(#5072),#878,.T.);
#30401=ADVANCED_FACE('',(#5073),#879,.T.);
#30402=ADVANCED_FACE('',(#5074),#880,.T.);
#30403=ADVANCED_FACE('',(#5075),#881,.T.);
#30404=ADVANCED_FACE('',(#5076),#882,.T.);
#30405=ADVANCED_FACE('',(#5077),#883,.T.);
#30406=ADVANCED_FACE('',(#5078),#884,.T.);
#30407=ADVANCED_FACE('',(#5079),#885,.T.);
#30408=ADVANCED_FACE('',(#5080),#886,.T.);
#30409=ADVANCED_FACE('',(#5081),#887,.T.);
#30410=ADVANCED_FACE('',(#5082),#888,.T.);
#30411=ADVANCED_FACE('',(#5083),#889,.T.);
#30412=ADVANCED_FACE('',(#5084),#890,.T.);
#30413=ADVANCED_FACE('',(#5085),#891,.T.);
#30414=ADVANCED_FACE('',(#5086),#892,.T.);
#30415=ADVANCED_FACE('',(#5087),#893,.T.);
#30416=ADVANCED_FACE('',(#5088),#894,.T.);
#30417=ADVANCED_FACE('',(#5089),#895,.T.);
#30418=ADVANCED_FACE('',(#5090),#896,.T.);
#30419=ADVANCED_FACE('',(#5091),#897,.T.);
#30420=ADVANCED_FACE('',(#5092),#898,.T.);
#30421=ADVANCED_FACE('',(#5093),#899,.T.);
#30422=ADVANCED_FACE('',(#5094),#900,.T.);
#30423=ADVANCED_FACE('',(#5095),#901,.T.);
#30424=ADVANCED_FACE('',(#5096),#902,.T.);
#30425=ADVANCED_FACE('',(#5097),#903,.T.);
#30426=ADVANCED_FACE('',(#5098),#904,.T.);
#30427=ADVANCED_FACE('',(#5099),#905,.T.);
#30428=ADVANCED_FACE('',(#5100),#906,.T.);
#30429=ADVANCED_FACE('',(#5101),#907,.T.);
#30430=ADVANCED_FACE('',(#5102),#908,.T.);
#30431=ADVANCED_FACE('',(#5103),#909,.T.);
#30432=ADVANCED_FACE('',(#5104),#910,.T.);
#30433=ADVANCED_FACE('',(#5105),#911,.T.);
#30434=ADVANCED_FACE('',(#5106),#912,.T.);
#30435=ADVANCED_FACE('',(#5107),#913,.T.);
#30436=ADVANCED_FACE('',(#5108),#914,.T.);
#30437=ADVANCED_FACE('',(#5109),#915,.T.);
#30438=ADVANCED_FACE('',(#5110),#916,.T.);
#30439=ADVANCED_FACE('',(#5111),#917,.T.);
#30440=ADVANCED_FACE('',(#5112),#918,.T.);
#30441=ADVANCED_FACE('',(#5113),#919,.T.);
#30442=ADVANCED_FACE('',(#5114),#920,.T.);
#30443=ADVANCED_FACE('',(#5115),#921,.T.);
#30444=ADVANCED_FACE('',(#5116),#922,.T.);
#30445=ADVANCED_FACE('',(#5117),#923,.T.);
#30446=ADVANCED_FACE('',(#5118),#924,.T.);
#30447=ADVANCED_FACE('',(#5119),#925,.T.);
#30448=ADVANCED_FACE('',(#5120),#926,.T.);
#30449=ADVANCED_FACE('',(#5121),#927,.T.);
#30450=ADVANCED_FACE('',(#5122),#928,.T.);
#30451=ADVANCED_FACE('',(#5123),#929,.T.);
#30452=ADVANCED_FACE('',(#5124),#930,.T.);
#30453=ADVANCED_FACE('',(#5125),#931,.T.);
#30454=ADVANCED_FACE('',(#5126),#932,.T.);
#30455=ADVANCED_FACE('',(#5127),#933,.T.);
#30456=ADVANCED_FACE('',(#5128),#934,.T.);
#30457=ADVANCED_FACE('',(#5129),#935,.T.);
#30458=ADVANCED_FACE('',(#5130),#936,.T.);
#30459=ADVANCED_FACE('',(#5131),#937,.T.);
#30460=ADVANCED_FACE('',(#5132),#938,.T.);
#30461=ADVANCED_FACE('',(#5133),#939,.T.);
#30462=ADVANCED_FACE('',(#5134),#940,.T.);
#30463=ADVANCED_FACE('',(#5135),#941,.T.);
#30464=ADVANCED_FACE('',(#5136),#942,.T.);
#30465=ADVANCED_FACE('',(#5137),#943,.T.);
#30466=ADVANCED_FACE('',(#5138),#944,.T.);
#30467=ADVANCED_FACE('',(#5139),#945,.T.);
#30468=ADVANCED_FACE('',(#5140),#946,.T.);
#30469=ADVANCED_FACE('',(#5141),#947,.T.);
#30470=ADVANCED_FACE('',(#5142),#948,.T.);
#30471=ADVANCED_FACE('',(#5143),#949,.T.);
#30472=ADVANCED_FACE('',(#5144),#950,.T.);
#30473=ADVANCED_FACE('',(#5145),#951,.T.);
#30474=ADVANCED_FACE('',(#5146),#952,.T.);
#30475=ADVANCED_FACE('',(#5147),#953,.T.);
#30476=ADVANCED_FACE('',(#5148),#954,.T.);
#30477=ADVANCED_FACE('',(#5149),#955,.T.);
#30478=ADVANCED_FACE('',(#5150),#956,.T.);
#30479=ADVANCED_FACE('',(#5151),#957,.T.);
#30480=ADVANCED_FACE('',(#5152),#958,.T.);
#30481=ADVANCED_FACE('',(#5153),#959,.T.);
#30482=ADVANCED_FACE('',(#5154),#960,.T.);
#30483=ADVANCED_FACE('',(#5155),#961,.T.);
#30484=ADVANCED_FACE('',(#5156),#962,.T.);
#30485=ADVANCED_FACE('',(#5157),#963,.T.);
#30486=ADVANCED_FACE('',(#5158),#964,.T.);
#30487=ADVANCED_FACE('',(#5159),#965,.T.);
#30488=ADVANCED_FACE('',(#5160),#966,.T.);
#30489=ADVANCED_FACE('',(#5161),#967,.T.);
#30490=ADVANCED_FACE('',(#5162),#968,.T.);
#30491=ADVANCED_FACE('',(#5163),#969,.T.);
#30492=ADVANCED_FACE('',(#5164),#970,.T.);
#30493=ADVANCED_FACE('',(#5165),#971,.T.);
#30494=ADVANCED_FACE('',(#5166),#972,.T.);
#30495=ADVANCED_FACE('',(#5167),#973,.T.);
#30496=ADVANCED_FACE('',(#5168),#974,.T.);
#30497=ADVANCED_FACE('',(#5169),#975,.T.);
#30498=ADVANCED_FACE('',(#5170),#976,.T.);
#30499=ADVANCED_FACE('',(#5171),#977,.T.);
#30500=ADVANCED_FACE('',(#5172),#978,.T.);
#30501=ADVANCED_FACE('',(#5173),#979,.T.);
#30502=ADVANCED_FACE('',(#5174),#980,.T.);
#30503=ADVANCED_FACE('',(#5175),#981,.T.);
#30504=ADVANCED_FACE('',(#5176),#982,.T.);
#30505=ADVANCED_FACE('',(#5177),#983,.T.);
#30506=ADVANCED_FACE('',(#5178),#984,.T.);
#30507=ADVANCED_FACE('',(#5179),#985,.T.);
#30508=ADVANCED_FACE('',(#5180),#986,.T.);
#30509=ADVANCED_FACE('',(#5181),#987,.T.);
#30510=ADVANCED_FACE('',(#5182),#988,.T.);
#30511=ADVANCED_FACE('',(#5183),#989,.T.);
#30512=ADVANCED_FACE('',(#5184),#990,.T.);
#30513=ADVANCED_FACE('',(#5185),#991,.T.);
#30514=ADVANCED_FACE('',(#5186),#992,.T.);
#30515=ADVANCED_FACE('',(#5187),#993,.T.);
#30516=ADVANCED_FACE('',(#5188),#994,.T.);
#30517=ADVANCED_FACE('',(#5189),#995,.T.);
#30518=ADVANCED_FACE('',(#5190),#996,.T.);
#30519=ADVANCED_FACE('',(#5191),#997,.T.);
#30520=ADVANCED_FACE('',(#5192),#998,.T.);
#30521=ADVANCED_FACE('',(#5193),#999,.T.);
#30522=ADVANCED_FACE('',(#5194),#28829,.F.);
#30523=ADVANCED_FACE('',(#5195),#429,.F.);
#30524=ADVANCED_FACE('',(#5196),#28830,.T.);
#30525=ADVANCED_FACE('',(#5197),#1000,.T.);
#30526=ADVANCED_FACE('',(#5198),#430,.F.);
#30527=ADVANCED_FACE('',(#5199),#1001,.T.);
#30528=ADVANCED_FACE('',(#5200),#2061,.T.);
#30529=ADVANCED_FACE('',(#5201),#1002,.T.);
#30530=ADVANCED_FACE('',(#5202),#2062,.T.);
#30531=ADVANCED_FACE('',(#5203),#28831,.T.);
#30532=ADVANCED_FACE('',(#5204,#3572),#156,.T.);
#30677=CLOSED_SHELL('',(#30372,#30373,#30374,#30375,#30376,#30377,#30378,
#30379,#30380,#30381,#30382,#30383,#30384,#30385,#30386,#30387,#30388,#30389,
#30390,#30391,#30392,#30393,#30394,#30395,#30396,#30397,#30398,#30399,#30400,
#30401,#30402,#30403,#30404,#30405,#30406,#30407,#30408,#30409,#30410,#30411,
#30412,#30413,#30414,#30415,#30416,#30417,#30418,#30419,#30420,#30421,#30422,
#30423,#30424,#30425,#30426,#30427,#30428,#30429,#30430,#30431,#30432,#30433,
#30434,#30435,#30436,#30437,#30438,#30439,#30440,#30441,#30442,#30443,#30444,
#30445,#30446,#30447,#30448,#30449,#30450,#30451,#30452,#30453,#30454,#30455,
#30456,#30457,#30458,#30459,#30460,#30461,#30462,#30463,#30464,#30465,#30466,
#30467,#30468,#30469,#30470,#30471,#30472,#30473,#30474,#30475,#30476,#30477,
#30478,#30479,#30480,#30481,#30482,#30483,#30484,#30485,#30486,#30487,#30488,
#30489,#30490,#30491,#30492,#30493,#30494,#30495,#30496,#30497,#30498,#30499,
#30500,#30501,#30502,#30503,#30504,#30505,#30506,#30507,#30508,#30509,#30510,
#30511,#30512,#30513,#30514,#30515,#30516,#30517,#30518,#30519,#30520,#30521,
#30522,#30523,#30524,#30525,#30526,#30527,#30528,#30529,#30530,#30531,#30532));
#32982=AXIS2_PLACEMENT_3D('',#70391,#39591,#39592);
#32983=AXIS2_PLACEMENT_3D('',#70392,#39593,#39594);
#32984=AXIS2_PLACEMENT_3D('',#70408,#39596,#39597);
#32985=AXIS2_PLACEMENT_3D('',#70419,#39598,#39599);
#32986=AXIS2_PLACEMENT_3D('',#70467,#39601,#39602);
#32987=AXIS2_PLACEMENT_3D('',#70515,#39604,#39605);
#32988=AXIS2_PLACEMENT_3D('',#70563,#39607,#39608);
#32989=AXIS2_PLACEMENT_3D('',#70617,#39610,#39611);
#32990=AXIS2_PLACEMENT_3D('',#70665,#39613,#39614);
#32991=AXIS2_PLACEMENT_3D('',#70713,#39616,#39617);
#32992=AXIS2_PLACEMENT_3D('',#70767,#39619,#39620);
#32993=AXIS2_PLACEMENT_3D('',#70815,#39622,#39623);
#32994=AXIS2_PLACEMENT_3D('',#70863,#39625,#39626);
#32995=AXIS2_PLACEMENT_3D('',#70914,#39628,#39629);
#32996=AXIS2_PLACEMENT_3D('',#70965,#39631,#39632);
#32997=AXIS2_PLACEMENT_3D('',#71013,#39634,#39635);
#32998=AXIS2_PLACEMENT_3D('',#71061,#39637,#39638);
#32999=AXIS2_PLACEMENT_3D('',#71115,#39640,#39641);
#33000=AXIS2_PLACEMENT_3D('',#71163,#39643,#39644);
#33001=AXIS2_PLACEMENT_3D('',#71211,#39646,#39647);
#33002=AXIS2_PLACEMENT_3D('',#71262,#39649,#39650);
#33003=AXIS2_PLACEMENT_3D('',#71310,#39652,#39653);
#33004=AXIS2_PLACEMENT_3D('',#71358,#39655,#39656);
#33005=AXIS2_PLACEMENT_3D('',#71406,#39658,#39659);
#33006=AXIS2_PLACEMENT_3D('',#71460,#39661,#39662);
#33007=AXIS2_PLACEMENT_3D('',#71508,#39664,#39665);
#33008=AXIS2_PLACEMENT_3D('',#71556,#39667,#39668);
#33009=AXIS2_PLACEMENT_3D('',#71610,#39670,#39671);
#33010=AXIS2_PLACEMENT_3D('',#71658,#39673,#39674);
#33011=AXIS2_PLACEMENT_3D('',#71706,#39676,#39677);
#33012=AXIS2_PLACEMENT_3D('',#71754,#39679,#39680);
#33013=AXIS2_PLACEMENT_3D('',#71808,#39682,#39683);
#33014=AXIS2_PLACEMENT_3D('',#71856,#39685,#39686);
#33015=AXIS2_PLACEMENT_3D('',#71904,#39688,#39689);
#33016=AXIS2_PLACEMENT_3D('',#71958,#39691,#39692);
#33017=AXIS2_PLACEMENT_3D('',#72006,#39694,#39695);
#33018=AXIS2_PLACEMENT_3D('',#72054,#39697,#39698);
#33019=AXIS2_PLACEMENT_3D('',#72102,#39700,#39701);
#33020=AXIS2_PLACEMENT_3D('',#72156,#39703,#39704);
#33021=AXIS2_PLACEMENT_3D('',#72204,#39706,#39707);
#33022=AXIS2_PLACEMENT_3D('',#72252,#39709,#39710);
#33023=AXIS2_PLACEMENT_3D('',#72306,#39712,#39713);
#33024=AXIS2_PLACEMENT_3D('',#72354,#39715,#39716);
#33025=AXIS2_PLACEMENT_3D('',#72402,#39718,#39719);
#33026=AXIS2_PLACEMENT_3D('',#72450,#39721,#39722);
#33027=AXIS2_PLACEMENT_3D('',#72504,#39724,#39725);
#33028=AXIS2_PLACEMENT_3D('',#72552,#39727,#39728);
#33029=AXIS2_PLACEMENT_3D('',#72600,#39730,#39731);
#33030=AXIS2_PLACEMENT_3D('',#72654,#39733,#39734);
#33031=AXIS2_PLACEMENT_3D('',#72702,#39736,#39737);
#33032=AXIS2_PLACEMENT_3D('',#72750,#39739,#39740);
#33033=AXIS2_PLACEMENT_3D('',#72798,#39742,#39743);
#33034=AXIS2_PLACEMENT_3D('',#72852,#39745,#39746);
#33035=AXIS2_PLACEMENT_3D('',#72900,#39748,#39749);
#33036=AXIS2_PLACEMENT_3D('',#72948,#39751,#39752);
#33037=AXIS2_PLACEMENT_3D('',#73002,#39754,#39755);
#33038=AXIS2_PLACEMENT_3D('',#73050,#39757,#39758);
#33039=AXIS2_PLACEMENT_3D('',#73098,#39760,#39761);
#33040=AXIS2_PLACEMENT_3D('',#73146,#39763,#39764);
#33041=AXIS2_PLACEMENT_3D('',#73200,#39766,#39767);
#33042=AXIS2_PLACEMENT_3D('',#73248,#39769,#39770);
#33043=AXIS2_PLACEMENT_3D('',#73296,#39772,#39773);
#33044=AXIS2_PLACEMENT_3D('',#73350,#39775,#39776);
#33045=AXIS2_PLACEMENT_3D('',#73398,#39778,#39779);
#33046=AXIS2_PLACEMENT_3D('',#73446,#39781,#39782);
#33047=AXIS2_PLACEMENT_3D('',#73497,#39784,#39785);
#33048=AXIS2_PLACEMENT_3D('',#73548,#39787,#39788);
#33049=AXIS2_PLACEMENT_3D('',#73596,#39790,#39791);
#33050=AXIS2_PLACEMENT_3D('',#73644,#39793,#39794);
#33051=AXIS2_PLACEMENT_3D('',#73698,#39796,#39797);
#33052=AXIS2_PLACEMENT_3D('',#73746,#39799,#39800);
#33053=AXIS2_PLACEMENT_3D('',#73794,#39802,#39803);
#33054=AXIS2_PLACEMENT_3D('',#73845,#39805,#39806);
#33055=AXIS2_PLACEMENT_3D('',#73893,#39808,#39809);
#33056=AXIS2_PLACEMENT_3D('',#73941,#39811,#39812);
#33057=AXIS2_PLACEMENT_3D('',#73989,#39814,#39815);
#33058=AXIS2_PLACEMENT_3D('',#74043,#39817,#39818);
#33059=AXIS2_PLACEMENT_3D('',#74091,#39820,#39821);
#33060=AXIS2_PLACEMENT_3D('',#74102,#39823,#39824);
#33061=AXIS2_PLACEMENT_3D('',#74107,#39825,#39826);
#33062=AXIS2_PLACEMENT_3D('',#74132,#39828,#39829);
#33063=AXIS2_PLACEMENT_3D('',#74157,#39831,#39832);
#33064=AXIS2_PLACEMENT_3D('',#74182,#39834,#39835);
#33065=AXIS2_PLACEMENT_3D('',#74206,#39837,#39838);
#33066=AXIS2_PLACEMENT_3D('',#74230,#39840,#39841);
#33067=AXIS2_PLACEMENT_3D('',#74255,#39843,#39844);
#33068=AXIS2_PLACEMENT_3D('',#74280,#39846,#39847);
#33069=AXIS2_PLACEMENT_3D('',#74304,#39849,#39850);
#33070=AXIS2_PLACEMENT_3D('',#74329,#39852,#39853);
#33071=AXIS2_PLACEMENT_3D('',#74354,#39855,#39856);
#33072=AXIS2_PLACEMENT_3D('',#74378,#39858,#39859);
#33073=AXIS2_PLACEMENT_3D('',#74403,#39861,#39862);
#33074=AXIS2_PLACEMENT_3D('',#74427,#39864,#39865);
#33075=AXIS2_PLACEMENT_3D('',#74452,#39867,#39868);
#33076=AXIS2_PLACEMENT_3D('',#74476,#39870,#39871);
#33077=AXIS2_PLACEMENT_3D('',#74501,#39873,#39874);
#33078=AXIS2_PLACEMENT_3D('',#74526,#39876,#39877);
#33079=AXIS2_PLACEMENT_3D('',#74550,#39879,#39880);
#33080=AXIS2_PLACEMENT_3D('',#74575,#39882,#39883);
#33081=AXIS2_PLACEMENT_3D('',#74600,#39885,#39886);
#33082=AXIS2_PLACEMENT_3D('',#74624,#39888,#39889);
#33083=AXIS2_PLACEMENT_3D('',#74648,#39891,#39892);
#33084=AXIS2_PLACEMENT_3D('',#74673,#39894,#39895);
#33085=AXIS2_PLACEMENT_3D('',#74698,#39897,#39898);
#33086=AXIS2_PLACEMENT_3D('',#74722,#39900,#39901);
#33087=AXIS2_PLACEMENT_3D('',#74747,#39903,#39904);
#33088=AXIS2_PLACEMENT_3D('',#74772,#39906,#39907);
#33089=AXIS2_PLACEMENT_3D('',#74796,#39909,#39910);
#33090=AXIS2_PLACEMENT_3D('',#74820,#39912,#39913);
#33091=AXIS2_PLACEMENT_3D('',#74845,#39915,#39916);
#33092=AXIS2_PLACEMENT_3D('',#74870,#39918,#39919);
#33093=AXIS2_PLACEMENT_3D('',#74894,#39921,#39922);
#33094=AXIS2_PLACEMENT_3D('',#74919,#39924,#39925);
#33095=AXIS2_PLACEMENT_3D('',#74944,#39927,#39928);
#33096=AXIS2_PLACEMENT_3D('',#74968,#39930,#39931);
#33097=AXIS2_PLACEMENT_3D('',#74992,#39933,#39934);
#33098=AXIS2_PLACEMENT_3D('',#75017,#39936,#39937);
#33099=AXIS2_PLACEMENT_3D('',#75042,#39939,#39940);
#33100=AXIS2_PLACEMENT_3D('',#75066,#39942,#39943);
#33101=AXIS2_PLACEMENT_3D('',#75091,#39945,#39946);
#33102=AXIS2_PLACEMENT_3D('',#75116,#39948,#39949);
#33103=AXIS2_PLACEMENT_3D('',#75140,#39951,#39952);
#33104=AXIS2_PLACEMENT_3D('',#75164,#39954,#39955);
#33105=AXIS2_PLACEMENT_3D('',#75189,#39957,#39958);
#33106=AXIS2_PLACEMENT_3D('',#75214,#39960,#39961);
#33107=AXIS2_PLACEMENT_3D('',#75238,#39963,#39964);
#33108=AXIS2_PLACEMENT_3D('',#75263,#39966,#39967);
#33109=AXIS2_PLACEMENT_3D('',#75288,#39969,#39970);
#33110=AXIS2_PLACEMENT_3D('',#75312,#39972,#39973);
#33111=AXIS2_PLACEMENT_3D('',#75336,#39975,#39976);
#33112=AXIS2_PLACEMENT_3D('',#75361,#39978,#39979);
#33113=AXIS2_PLACEMENT_3D('',#75386,#39981,#39982);
#33114=AXIS2_PLACEMENT_3D('',#75410,#39984,#39985);
#33115=AXIS2_PLACEMENT_3D('',#75435,#39987,#39988);
#33116=AXIS2_PLACEMENT_3D('',#75460,#39990,#39991);
#33117=AXIS2_PLACEMENT_3D('',#75484,#39993,#39994);
#33118=AXIS2_PLACEMENT_3D('',#75508,#39996,#39997);
#33119=AXIS2_PLACEMENT_3D('',#75533,#39999,#40000);
#33120=AXIS2_PLACEMENT_3D('',#75558,#40002,#40003);
#33121=AXIS2_PLACEMENT_3D('',#75582,#40005,#40006);
#33122=AXIS2_PLACEMENT_3D('',#75607,#40008,#40009);
#33123=AXIS2_PLACEMENT_3D('',#75632,#40011,#40012);
#33124=AXIS2_PLACEMENT_3D('',#75656,#40014,#40015);
#33125=AXIS2_PLACEMENT_3D('',#75681,#40017,#40018);
#33126=AXIS2_PLACEMENT_3D('',#75705,#40020,#40021);
#33127=AXIS2_PLACEMENT_3D('',#75730,#40023,#40024);
#33128=AXIS2_PLACEMENT_3D('',#75754,#40026,#40027);
#33129=AXIS2_PLACEMENT_3D('',#75779,#40029,#40030);
#33130=AXIS2_PLACEMENT_3D('',#75804,#40032,#40033);
#33131=AXIS2_PLACEMENT_3D('',#75828,#40035,#40036);
#33132=AXIS2_PLACEMENT_3D('',#75853,#40038,#40039);
#33133=AXIS2_PLACEMENT_3D('',#75878,#40041,#40042);
#33134=AXIS2_PLACEMENT_3D('',#75902,#40044,#40045);
#33135=AXIS2_PLACEMENT_3D('',#75926,#40047,#40048);
#33136=AXIS2_PLACEMENT_3D('',#76035,#40049,#40050);
#33137=AXIS2_PLACEMENT_3D('',#76037,#40051,#40052);
#33138=AXIS2_PLACEMENT_3D('',#78191,#40053,#40054);
#33139=AXIS2_PLACEMENT_3D('',#78193,#40055,#40056);
#33140=AXIS2_PLACEMENT_3D('',#78194,#40057,#40058);
#33141=AXIS2_PLACEMENT_3D('',#78305,#40059,#40060);
#33142=AXIS2_PLACEMENT_3D('',#78306,#40061,#40062);
#33143=AXIS2_PLACEMENT_3D('',#80244,#40063,#40064);
#33144=AXIS2_PLACEMENT_3D('',#80246,#40065,#40066);
#33145=AXIS2_PLACEMENT_3D('',#80249,#40068,#40069);
#33146=AXIS2_PLACEMENT_3D('',#80250,#40070,#40071);
#33147=AXIS2_PLACEMENT_3D('',#80252,#40073,#40074);
#33148=AXIS2_PLACEMENT_3D('',#80253,#40075,#40076);
#33149=AXIS2_PLACEMENT_3D('',#80254,#40077,#40078);
#33150=AXIS2_PLACEMENT_3D('',#80256,#40079,#40080);
#33151=AXIS2_PLACEMENT_3D('',#80258,#40082,#40083);
#33152=AXIS2_PLACEMENT_3D('',#80259,#40084,#40085);
#33153=AXIS2_PLACEMENT_3D('',#80262,#40086,#40087);
#39591=DIRECTION('axis',(0.,0.,1.));
#39592=DIRECTION('refdir',(1.,0.,0.));
#39593=DIRECTION('center_axis',(1.,0.,0.));
#39594=DIRECTION('ref_axis',(0.,1.,0.));
#39595=DIRECTION('',(-1.,0.,0.));
#39596=DIRECTION('center_axis',(1.,0.,0.));
#39597=DIRECTION('ref_axis',(0.,1.,0.));
#39598=DIRECTION('center_axis',(1.,0.,0.));
#39599=DIRECTION('ref_axis',(0.,1.,0.));
#39600=DIRECTION('',(-1.,0.,0.));
#39601=DIRECTION('center_axis',(1.,0.,0.));
#39602=DIRECTION('ref_axis',(0.,1.,0.));
#39603=DIRECTION('',(-1.,0.,0.));
#39604=DIRECTION('center_axis',(1.,0.,0.));
#39605=DIRECTION('ref_axis',(0.,1.,0.));
#39606=DIRECTION('',(-1.,0.,0.));
#39607=DIRECTION('center_axis',(1.,0.,0.));
#39608=DIRECTION('ref_axis',(0.,1.,0.));
#39609=DIRECTION('',(-1.,0.,0.));
#39610=DIRECTION('center_axis',(1.,0.,0.));
#39611=DIRECTION('ref_axis',(0.,1.,0.));
#39612=DIRECTION('',(-1.,0.,0.));
#39613=DIRECTION('center_axis',(1.,0.,0.));
#39614=DIRECTION('ref_axis',(0.,1.,0.));
#39615=DIRECTION('',(-1.,0.,0.));
#39616=DIRECTION('center_axis',(1.,0.,0.));
#39617=DIRECTION('ref_axis',(0.,1.,0.));
#39618=DIRECTION('',(-1.,0.,0.));
#39619=DIRECTION('center_axis',(1.,0.,0.));
#39620=DIRECTION('ref_axis',(0.,1.,0.));
#39621=DIRECTION('',(-1.,0.,0.));
#39622=DIRECTION('center_axis',(1.,0.,0.));
#39623=DIRECTION('ref_axis',(0.,1.,0.));
#39624=DIRECTION('',(-1.,0.,0.));
#39625=DIRECTION('center_axis',(1.,0.,0.));
#39626=DIRECTION('ref_axis',(0.,1.,0.));
#39627=DIRECTION('',(-1.,0.,0.));
#39628=DIRECTION('center_axis',(1.,0.,0.));
#39629=DIRECTION('ref_axis',(0.,1.,0.));
#39630=DIRECTION('',(-1.,0.,0.));
#39631=DIRECTION('center_axis',(1.,0.,0.));
#39632=DIRECTION('ref_axis',(0.,1.,0.));
#39633=DIRECTION('',(-1.,0.,0.));
#39634=DIRECTION('center_axis',(1.,0.,0.));
#39635=DIRECTION('ref_axis',(0.,1.,0.));
#39636=DIRECTION('',(-1.,0.,0.));
#39637=DIRECTION('center_axis',(1.,0.,0.));
#39638=DIRECTION('ref_axis',(0.,1.,0.));
#39639=DIRECTION('',(-1.,0.,0.));
#39640=DIRECTION('center_axis',(1.,0.,0.));
#39641=DIRECTION('ref_axis',(0.,1.,0.));
#39642=DIRECTION('',(-1.,0.,0.));
#39643=DIRECTION('center_axis',(1.,0.,0.));
#39644=DIRECTION('ref_axis',(0.,1.,0.));
#39645=DIRECTION('',(-1.,0.,0.));
#39646=DIRECTION('center_axis',(1.,0.,0.));
#39647=DIRECTION('ref_axis',(0.,1.,0.));
#39648=DIRECTION('',(-1.,0.,0.));
#39649=DIRECTION('center_axis',(1.,0.,0.));
#39650=DIRECTION('ref_axis',(0.,1.,0.));
#39651=DIRECTION('',(-1.,0.,0.));
#39652=DIRECTION('center_axis',(1.,0.,0.));
#39653=DIRECTION('ref_axis',(0.,1.,0.));
#39654=DIRECTION('',(-1.,0.,0.));
#39655=DIRECTION('center_axis',(1.,0.,0.));
#39656=DIRECTION('ref_axis',(0.,1.,0.));
#39657=DIRECTION('',(-1.,0.,0.));
#39658=DIRECTION('center_axis',(1.,0.,0.));
#39659=DIRECTION('ref_axis',(0.,1.,0.));
#39660=DIRECTION('',(-1.,0.,0.));
#39661=DIRECTION('center_axis',(1.,0.,0.));
#39662=DIRECTION('ref_axis',(0.,1.,0.));
#39663=DIRECTION('',(-1.,0.,0.));
#39664=DIRECTION('center_axis',(1.,0.,0.));
#39665=DIRECTION('ref_axis',(0.,1.,0.));
#39666=DIRECTION('',(-1.,0.,0.));
#39667=DIRECTION('center_axis',(1.,0.,0.));
#39668=DIRECTION('ref_axis',(0.,1.,0.));
#39669=DIRECTION('',(-1.,0.,0.));
#39670=DIRECTION('center_axis',(1.,0.,0.));
#39671=DIRECTION('ref_axis',(0.,1.,0.));
#39672=DIRECTION('',(-1.,0.,0.));
#39673=DIRECTION('center_axis',(1.,0.,0.));
#39674=DIRECTION('ref_axis',(0.,1.,0.));
#39675=DIRECTION('',(-1.,0.,0.));
#39676=DIRECTION('center_axis',(1.,0.,0.));
#39677=DIRECTION('ref_axis',(0.,1.,0.));
#39678=DIRECTION('',(-1.,0.,0.));
#39679=DIRECTION('center_axis',(1.,0.,0.));
#39680=DIRECTION('ref_axis',(0.,1.,0.));
#39681=DIRECTION('',(-1.,0.,0.));
#39682=DIRECTION('center_axis',(1.,0.,0.));
#39683=DIRECTION('ref_axis',(0.,1.,0.));
#39684=DIRECTION('',(-1.,0.,0.));
#39685=DIRECTION('center_axis',(1.,0.,0.));
#39686=DIRECTION('ref_axis',(0.,1.,0.));
#39687=DIRECTION('',(-1.,0.,0.));
#39688=DIRECTION('center_axis',(1.,0.,0.));
#39689=DIRECTION('ref_axis',(0.,1.,0.));
#39690=DIRECTION('',(-1.,0.,0.));
#39691=DIRECTION('center_axis',(1.,0.,0.));
#39692=DIRECTION('ref_axis',(0.,1.,0.));
#39693=DIRECTION('',(-1.,0.,0.));
#39694=DIRECTION('center_axis',(1.,0.,0.));
#39695=DIRECTION('ref_axis',(0.,1.,0.));
#39696=DIRECTION('',(-1.,0.,0.));
#39697=DIRECTION('center_axis',(1.,0.,0.));
#39698=DIRECTION('ref_axis',(0.,1.,0.));
#39699=DIRECTION('',(-1.,0.,0.));
#39700=DIRECTION('center_axis',(1.,0.,0.));
#39701=DIRECTION('ref_axis',(0.,1.,0.));
#39702=DIRECTION('',(-1.,0.,0.));
#39703=DIRECTION('center_axis',(1.,0.,0.));
#39704=DIRECTION('ref_axis',(0.,1.,0.));
#39705=DIRECTION('',(-1.,0.,0.));
#39706=DIRECTION('center_axis',(1.,0.,0.));
#39707=DIRECTION('ref_axis',(0.,1.,0.));
#39708=DIRECTION('',(-1.,0.,0.));
#39709=DIRECTION('center_axis',(1.,0.,0.));
#39710=DIRECTION('ref_axis',(0.,1.,0.));
#39711=DIRECTION('',(-1.,0.,0.));
#39712=DIRECTION('center_axis',(1.,0.,0.));
#39713=DIRECTION('ref_axis',(0.,1.,0.));
#39714=DIRECTION('',(-1.,0.,0.));
#39715=DIRECTION('center_axis',(1.,0.,0.));
#39716=DIRECTION('ref_axis',(0.,1.,0.));
#39717=DIRECTION('',(-1.,0.,0.));
#39718=DIRECTION('center_axis',(1.,0.,0.));
#39719=DIRECTION('ref_axis',(0.,1.,0.));
#39720=DIRECTION('',(-1.,0.,0.));
#39721=DIRECTION('center_axis',(1.,0.,0.));
#39722=DIRECTION('ref_axis',(0.,1.,0.));
#39723=DIRECTION('',(-1.,0.,0.));
#39724=DIRECTION('center_axis',(1.,0.,0.));
#39725=DIRECTION('ref_axis',(0.,1.,0.));
#39726=DIRECTION('',(-1.,0.,0.));
#39727=DIRECTION('center_axis',(1.,0.,0.));
#39728=DIRECTION('ref_axis',(0.,1.,0.));
#39729=DIRECTION('',(-1.,0.,0.));
#39730=DIRECTION('center_axis',(1.,0.,0.));
#39731=DIRECTION('ref_axis',(0.,1.,0.));
#39732=DIRECTION('',(-1.,0.,0.));
#39733=DIRECTION('center_axis',(1.,0.,0.));
#39734=DIRECTION('ref_axis',(0.,1.,0.));
#39735=DIRECTION('',(-1.,0.,0.));
#39736=DIRECTION('center_axis',(1.,0.,0.));
#39737=DIRECTION('ref_axis',(0.,1.,0.));
#39738=DIRECTION('',(-1.,0.,0.));
#39739=DIRECTION('center_axis',(1.,0.,0.));
#39740=DIRECTION('ref_axis',(0.,1.,0.));
#39741=DIRECTION('',(-1.,0.,0.));
#39742=DIRECTION('center_axis',(1.,0.,0.));
#39743=DIRECTION('ref_axis',(0.,1.,0.));
#39744=DIRECTION('',(-1.,0.,0.));
#39745=DIRECTION('center_axis',(1.,0.,0.));
#39746=DIRECTION('ref_axis',(0.,1.,0.));
#39747=DIRECTION('',(-1.,0.,0.));
#39748=DIRECTION('center_axis',(1.,0.,0.));
#39749=DIRECTION('ref_axis',(0.,1.,0.));
#39750=DIRECTION('',(-1.,0.,0.));
#39751=DIRECTION('center_axis',(1.,0.,0.));
#39752=DIRECTION('ref_axis',(0.,1.,0.));
#39753=DIRECTION('',(-1.,0.,0.));
#39754=DIRECTION('center_axis',(1.,0.,0.));
#39755=DIRECTION('ref_axis',(0.,1.,0.));
#39756=DIRECTION('',(-1.,0.,0.));
#39757=DIRECTION('center_axis',(1.,0.,0.));
#39758=DIRECTION('ref_axis',(0.,1.,0.));
#39759=DIRECTION('',(-1.,0.,0.));
#39760=DIRECTION('center_axis',(1.,0.,0.));
#39761=DIRECTION('ref_axis',(0.,1.,0.));
#39762=DIRECTION('',(-1.,0.,0.));
#39763=DIRECTION('center_axis',(1.,0.,0.));
#39764=DIRECTION('ref_axis',(0.,1.,0.));
#39765=DIRECTION('',(-1.,0.,0.));
#39766=DIRECTION('center_axis',(1.,0.,0.));
#39767=DIRECTION('ref_axis',(0.,1.,0.));
#39768=DIRECTION('',(-1.,0.,0.));
#39769=DIRECTION('center_axis',(1.,0.,0.));
#39770=DIRECTION('ref_axis',(0.,1.,0.));
#39771=DIRECTION('',(-1.,0.,0.));
#39772=DIRECTION('center_axis',(1.,0.,0.));
#39773=DIRECTION('ref_axis',(0.,1.,0.));
#39774=DIRECTION('',(-1.,0.,0.));
#39775=DIRECTION('center_axis',(1.,0.,0.));
#39776=DIRECTION('ref_axis',(0.,1.,0.));
#39777=DIRECTION('',(-1.,0.,0.));
#39778=DIRECTION('center_axis',(1.,0.,0.));
#39779=DIRECTION('ref_axis',(0.,1.,0.));
#39780=DIRECTION('',(-1.,0.,0.));
#39781=DIRECTION('center_axis',(1.,0.,0.));
#39782=DIRECTION('ref_axis',(0.,1.,0.));
#39783=DIRECTION('',(-1.,0.,0.));
#39784=DIRECTION('center_axis',(1.,0.,0.));
#39785=DIRECTION('ref_axis',(0.,1.,0.));
#39786=DIRECTION('',(-1.,0.,0.));
#39787=DIRECTION('center_axis',(1.,0.,0.));
#39788=DIRECTION('ref_axis',(0.,1.,0.));
#39789=DIRECTION('',(-1.,0.,0.));
#39790=DIRECTION('center_axis',(1.,0.,0.));
#39791=DIRECTION('ref_axis',(0.,1.,0.));
#39792=DIRECTION('',(-1.,0.,0.));
#39793=DIRECTION('center_axis',(1.,0.,0.));
#39794=DIRECTION('ref_axis',(0.,1.,0.));
#39795=DIRECTION('',(-1.,0.,0.));
#39796=DIRECTION('center_axis',(1.,0.,0.));
#39797=DIRECTION('ref_axis',(0.,1.,0.));
#39798=DIRECTION('',(-1.,0.,0.));
#39799=DIRECTION('center_axis',(1.,0.,0.));
#39800=DIRECTION('ref_axis',(0.,1.,0.));
#39801=DIRECTION('',(-1.,0.,0.));
#39802=DIRECTION('center_axis',(1.,0.,0.));
#39803=DIRECTION('ref_axis',(0.,1.,0.));
#39804=DIRECTION('',(-1.,0.,0.));
#39805=DIRECTION('center_axis',(1.,0.,0.));
#39806=DIRECTION('ref_axis',(0.,1.,0.));
#39807=DIRECTION('',(-1.,0.,0.));
#39808=DIRECTION('center_axis',(1.,0.,0.));
#39809=DIRECTION('ref_axis',(0.,1.,0.));
#39810=DIRECTION('',(-1.,0.,0.));
#39811=DIRECTION('center_axis',(1.,0.,0.));
#39812=DIRECTION('ref_axis',(0.,1.,0.));
#39813=DIRECTION('',(-1.,0.,0.));
#39814=DIRECTION('center_axis',(1.,0.,0.));
#39815=DIRECTION('ref_axis',(0.,1.,0.));
#39816=DIRECTION('',(-1.,0.,0.));
#39817=DIRECTION('center_axis',(1.,0.,0.));
#39818=DIRECTION('ref_axis',(0.,1.,0.));
#39819=DIRECTION('',(-1.,0.,0.));
#39820=DIRECTION('center_axis',(1.,0.,0.));
#39821=DIRECTION('ref_axis',(0.,-0.740693059652024,-0.671843576573687));
#39822=DIRECTION('',(1.,0.,0.));
#39823=DIRECTION('center_axis',(1.,0.,0.));
#39824=DIRECTION('ref_axis',(0.,1.,-1.13773497930895E-12));
#39825=DIRECTION('center_axis',(1.,0.,0.));
#39826=DIRECTION('ref_axis',(0.,1.,-1.13773497930895E-12));
#39827=DIRECTION('',(1.,0.,0.));
#39828=DIRECTION('center_axis',(1.,0.,0.));
#39829=DIRECTION('ref_axis',(0.,1.,-1.13773497930895E-12));
#39830=DIRECTION('',(1.,0.,0.));
#39831=DIRECTION('center_axis',(1.,0.,0.));
#39832=DIRECTION('ref_axis',(0.,1.,-1.13773497930895E-12));
#39833=DIRECTION('',(1.,0.,0.));
#39834=DIRECTION('center_axis',(1.,0.,0.));
#39835=DIRECTION('ref_axis',(0.,1.,-1.13773497930895E-12));
#39836=DIRECTION('',(1.,0.,0.));
#39837=DIRECTION('center_axis',(1.,0.,0.));
#39838=DIRECTION('ref_axis',(0.,1.,-1.13773497930895E-12));
#39839=DIRECTION('',(1.,0.,0.));
#39840=DIRECTION('center_axis',(1.,0.,0.));
#39841=DIRECTION('ref_axis',(0.,1.,-1.13773497930895E-12));
#39842=DIRECTION('',(1.,0.,0.));
#39843=DIRECTION('center_axis',(1.,0.,0.));
#39844=DIRECTION('ref_axis',(0.,1.,-1.13773497930895E-12));
#39845=DIRECTION('',(1.,0.,0.));
#39846=DIRECTION('center_axis',(1.,0.,0.));
#39847=DIRECTION('ref_axis',(0.,1.,-1.13773497930895E-12));
#39848=DIRECTION('',(1.,0.,0.));
#39849=DIRECTION('center_axis',(1.,0.,0.));
#39850=DIRECTION('ref_axis',(0.,1.,-1.13773497930895E-12));
#39851=DIRECTION('',(1.,0.,0.));
#39852=DIRECTION('center_axis',(1.,0.,0.));
#39853=DIRECTION('ref_axis',(0.,1.,-1.13773497930895E-12));
#39854=DIRECTION('',(1.,0.,0.));
#39855=DIRECTION('center_axis',(1.,0.,0.));
#39856=DIRECTION('ref_axis',(0.,1.,-1.13773497930895E-12));
#39857=DIRECTION('',(1.,0.,0.));
#39858=DIRECTION('center_axis',(1.,0.,0.));
#39859=DIRECTION('ref_axis',(0.,1.,-1.13773497930895E-12));
#39860=DIRECTION('',(1.,0.,0.));
#39861=DIRECTION('center_axis',(1.,0.,0.));
#39862=DIRECTION('ref_axis',(0.,1.,-1.13773497930895E-12));
#39863=DIRECTION('',(1.,0.,0.));
#39864=DIRECTION('center_axis',(1.,0.,0.));
#39865=DIRECTION('ref_axis',(0.,1.,-1.13773497930895E-12));
#39866=DIRECTION('',(1.,0.,0.));
#39867=DIRECTION('center_axis',(1.,0.,0.));
#39868=DIRECTION('ref_axis',(0.,1.,-1.13773497930895E-12));
#39869=DIRECTION('',(1.,0.,0.));
#39870=DIRECTION('center_axis',(1.,0.,0.));
#39871=DIRECTION('ref_axis',(0.,1.,-1.13773497930895E-12));
#39872=DIRECTION('',(1.,0.,0.));
#39873=DIRECTION('center_axis',(1.,0.,0.));
#39874=DIRECTION('ref_axis',(0.,1.,-1.13773497930895E-12));
#39875=DIRECTION('',(1.,0.,0.));
#39876=DIRECTION('center_axis',(1.,0.,0.));
#39877=DIRECTION('ref_axis',(0.,1.,-1.13773497930895E-12));
#39878=DIRECTION('',(1.,0.,0.));
#39879=DIRECTION('center_axis',(1.,0.,0.));
#39880=DIRECTION('ref_axis',(0.,1.,-1.13773497930895E-12));
#39881=DIRECTION('',(1.,0.,0.));
#39882=DIRECTION('center_axis',(1.,0.,0.));
#39883=DIRECTION('ref_axis',(0.,1.,-1.13773497930895E-12));
#39884=DIRECTION('',(1.,0.,0.));
#39885=DIRECTION('center_axis',(1.,0.,0.));
#39886=DIRECTION('ref_axis',(0.,1.,-1.13773497930895E-12));
#39887=DIRECTION('',(1.,0.,0.));
#39888=DIRECTION('center_axis',(1.,0.,0.));
#39889=DIRECTION('ref_axis',(0.,1.,-1.13773497930895E-12));
#39890=DIRECTION('',(1.,0.,0.));
#39891=DIRECTION('center_axis',(1.,0.,0.));
#39892=DIRECTION('ref_axis',(0.,1.,-1.13773497930895E-12));
#39893=DIRECTION('',(1.,0.,0.));
#39894=DIRECTION('center_axis',(1.,0.,0.));
#39895=DIRECTION('ref_axis',(0.,1.,-1.13773497930895E-12));
#39896=DIRECTION('',(1.,0.,0.));
#39897=DIRECTION('center_axis',(1.,0.,0.));
#39898=DIRECTION('ref_axis',(0.,1.,-1.13773497930895E-12));
#39899=DIRECTION('',(1.,0.,0.));
#39900=DIRECTION('center_axis',(1.,0.,0.));
#39901=DIRECTION('ref_axis',(0.,1.,-1.13773497930895E-12));
#39902=DIRECTION('',(1.,0.,0.));
#39903=DIRECTION('center_axis',(1.,0.,0.));
#39904=DIRECTION('ref_axis',(0.,1.,-1.13773497930895E-12));
#39905=DIRECTION('',(1.,0.,0.));
#39906=DIRECTION('center_axis',(1.,0.,0.));
#39907=DIRECTION('ref_axis',(0.,1.,-1.13773497930895E-12));
#39908=DIRECTION('',(1.,0.,0.));
#39909=DIRECTION('center_axis',(1.,0.,0.));
#39910=DIRECTION('ref_axis',(0.,1.,-1.13773497930895E-12));
#39911=DIRECTION('',(1.,0.,0.));
#39912=DIRECTION('center_axis',(1.,0.,0.));
#39913=DIRECTION('ref_axis',(0.,1.,-1.13773497930895E-12));
#39914=DIRECTION('',(1.,0.,0.));
#39915=DIRECTION('center_axis',(1.,0.,0.));
#39916=DIRECTION('ref_axis',(0.,1.,-1.13773497930895E-12));
#39917=DIRECTION('',(1.,0.,0.));
#39918=DIRECTION('center_axis',(1.,0.,0.));
#39919=DIRECTION('ref_axis',(0.,1.,-1.13773497930895E-12));
#39920=DIRECTION('',(1.,0.,0.));
#39921=DIRECTION('center_axis',(1.,0.,0.));
#39922=DIRECTION('ref_axis',(0.,1.,-1.13773497930895E-12));
#39923=DIRECTION('',(1.,0.,0.));
#39924=DIRECTION('center_axis',(1.,0.,0.));
#39925=DIRECTION('ref_axis',(0.,1.,-1.13773497930895E-12));
#39926=DIRECTION('',(1.,0.,0.));
#39927=DIRECTION('center_axis',(1.,0.,0.));
#39928=DIRECTION('ref_axis',(0.,1.,-1.13773497930895E-12));
#39929=DIRECTION('',(1.,0.,0.));
#39930=DIRECTION('center_axis',(1.,0.,0.));
#39931=DIRECTION('ref_axis',(0.,1.,-1.13773497930895E-12));
#39932=DIRECTION('',(1.,0.,0.));
#39933=DIRECTION('center_axis',(1.,0.,0.));
#39934=DIRECTION('ref_axis',(0.,1.,-1.13773497930895E-12));
#39935=DIRECTION('',(1.,0.,0.));
#39936=DIRECTION('center_axis',(1.,0.,0.));
#39937=DIRECTION('ref_axis',(0.,1.,-1.13773497930895E-12));
#39938=DIRECTION('',(1.,0.,0.));
#39939=DIRECTION('center_axis',(1.,0.,0.));
#39940=DIRECTION('ref_axis',(0.,1.,-1.13773497930895E-12));
#39941=DIRECTION('',(1.,0.,0.));
#39942=DIRECTION('center_axis',(1.,0.,0.));
#39943=DIRECTION('ref_axis',(0.,1.,-1.13773497930895E-12));
#39944=DIRECTION('',(1.,0.,0.));
#39945=DIRECTION('center_axis',(1.,0.,0.));
#39946=DIRECTION('ref_axis',(0.,1.,-1.13773497930895E-12));
#39947=DIRECTION('',(1.,0.,0.));
#39948=DIRECTION('center_axis',(1.,0.,0.));
#39949=DIRECTION('ref_axis',(0.,1.,-1.13773497930895E-12));
#39950=DIRECTION('',(1.,0.,0.));
#39951=DIRECTION('center_axis',(1.,0.,0.));
#39952=DIRECTION('ref_axis',(0.,1.,-1.13773497930895E-12));
#39953=DIRECTION('',(1.,0.,0.));
#39954=DIRECTION('center_axis',(1.,0.,0.));
#39955=DIRECTION('ref_axis',(0.,1.,-1.13773497930895E-12));
#39956=DIRECTION('',(1.,0.,0.));
#39957=DIRECTION('center_axis',(1.,0.,0.));
#39958=DIRECTION('ref_axis',(0.,1.,-1.13773497930895E-12));
#39959=DIRECTION('',(1.,0.,0.));
#39960=DIRECTION('center_axis',(1.,0.,0.));
#39961=DIRECTION('ref_axis',(0.,1.,-1.13773497930895E-12));
#39962=DIRECTION('',(1.,0.,0.));
#39963=DIRECTION('center_axis',(1.,0.,0.));
#39964=DIRECTION('ref_axis',(0.,1.,-1.13773497930895E-12));
#39965=DIRECTION('',(1.,0.,0.));
#39966=DIRECTION('center_axis',(1.,0.,0.));
#39967=DIRECTION('ref_axis',(0.,1.,-1.13773497930895E-12));
#39968=DIRECTION('',(1.,0.,0.));
#39969=DIRECTION('center_axis',(1.,0.,0.));
#39970=DIRECTION('ref_axis',(0.,1.,-1.13773497930895E-12));
#39971=DIRECTION('',(1.,0.,0.));
#39972=DIRECTION('center_axis',(1.,0.,0.));
#39973=DIRECTION('ref_axis',(0.,1.,-1.13773497930895E-12));
#39974=DIRECTION('',(1.,0.,0.));
#39975=DIRECTION('center_axis',(1.,0.,0.));
#39976=DIRECTION('ref_axis',(0.,1.,-1.13773497930895E-12));
#39977=DIRECTION('',(1.,0.,0.));
#39978=DIRECTION('center_axis',(1.,0.,0.));
#39979=DIRECTION('ref_axis',(0.,1.,-1.13773497930895E-12));
#39980=DIRECTION('',(1.,0.,0.));
#39981=DIRECTION('center_axis',(1.,0.,0.));
#39982=DIRECTION('ref_axis',(0.,1.,-1.13773497930895E-12));
#39983=DIRECTION('',(1.,0.,0.));
#39984=DIRECTION('center_axis',(1.,0.,0.));
#39985=DIRECTION('ref_axis',(0.,1.,-1.13773497930895E-12));
#39986=DIRECTION('',(1.,0.,0.));
#39987=DIRECTION('center_axis',(1.,0.,0.));
#39988=DIRECTION('ref_axis',(0.,1.,-1.13773497930895E-12));
#39989=DIRECTION('',(1.,0.,0.));
#39990=DIRECTION('center_axis',(1.,0.,0.));
#39991=DIRECTION('ref_axis',(0.,1.,-1.13773497930895E-12));
#39992=DIRECTION('',(1.,0.,0.));
#39993=DIRECTION('center_axis',(1.,0.,0.));
#39994=DIRECTION('ref_axis',(0.,1.,-1.13773497930895E-12));
#39995=DIRECTION('',(1.,0.,0.));
#39996=DIRECTION('center_axis',(1.,0.,0.));
#39997=DIRECTION('ref_axis',(0.,1.,-1.13773497930895E-12));
#39998=DIRECTION('',(1.,0.,0.));
#39999=DIRECTION('center_axis',(1.,0.,0.));
#40000=DIRECTION('ref_axis',(0.,1.,-1.13773497930895E-12));
#40001=DIRECTION('',(1.,0.,0.));
#40002=DIRECTION('center_axis',(1.,0.,0.));
#40003=DIRECTION('ref_axis',(0.,1.,-1.13773497930895E-12));
#40004=DIRECTION('',(1.,0.,0.));
#40005=DIRECTION('center_axis',(1.,0.,0.));
#40006=DIRECTION('ref_axis',(0.,1.,-1.13773497930895E-12));
#40007=DIRECTION('',(1.,0.,0.));
#40008=DIRECTION('center_axis',(1.,0.,0.));
#40009=DIRECTION('ref_axis',(0.,1.,-1.13773497930895E-12));
#40010=DIRECTION('',(1.,0.,0.));
#40011=DIRECTION('center_axis',(1.,0.,0.));
#40012=DIRECTION('ref_axis',(0.,1.,-1.13773497930895E-12));
#40013=DIRECTION('',(1.,0.,0.));
#40014=DIRECTION('center_axis',(1.,0.,0.));
#40015=DIRECTION('ref_axis',(0.,1.,-1.13773497930895E-12));
#40016=DIRECTION('',(1.,0.,0.));
#40017=DIRECTION('center_axis',(1.,0.,0.));
#40018=DIRECTION('ref_axis',(0.,1.,-1.13773497930895E-12));
#40019=DIRECTION('',(1.,0.,0.));
#40020=DIRECTION('center_axis',(1.,0.,0.));
#40021=DIRECTION('ref_axis',(0.,1.,-1.13773497930895E-12));
#40022=DIRECTION('',(1.,0.,0.));
#40023=DIRECTION('center_axis',(1.,0.,0.));
#40024=DIRECTION('ref_axis',(0.,1.,-1.13773497930895E-12));
#40025=DIRECTION('',(1.,0.,0.));
#40026=DIRECTION('center_axis',(1.,0.,0.));
#40027=DIRECTION('ref_axis',(0.,1.,-1.13773497930895E-12));
#40028=DIRECTION('',(1.,0.,0.));
#40029=DIRECTION('center_axis',(1.,0.,0.));
#40030=DIRECTION('ref_axis',(0.,1.,-1.13773497930895E-12));
#40031=DIRECTION('',(1.,0.,0.));
#40032=DIRECTION('center_axis',(1.,0.,0.));
#40033=DIRECTION('ref_axis',(0.,1.,-1.13773497930895E-12));
#40034=DIRECTION('',(1.,0.,0.));
#40035=DIRECTION('center_axis',(1.,0.,0.));
#40036=DIRECTION('ref_axis',(0.,1.,-1.13773497930895E-12));
#40037=DIRECTION('',(1.,0.,0.));
#40038=DIRECTION('center_axis',(1.,0.,0.));
#40039=DIRECTION('ref_axis',(0.,1.,-1.13773497930895E-12));
#40040=DIRECTION('',(1.,0.,0.));
#40041=DIRECTION('center_axis',(1.,0.,0.));
#40042=DIRECTION('ref_axis',(0.,1.,-1.13773497930895E-12));
#40043=DIRECTION('',(1.,0.,0.));
#40044=DIRECTION('center_axis',(1.,0.,0.));
#40045=DIRECTION('ref_axis',(0.,1.,-1.13773497930895E-12));
#40046=DIRECTION('',(1.,0.,0.));
#40047=DIRECTION('center_axis',(1.,0.,0.));
#40048=DIRECTION('ref_axis',(0.,0.,-1.));
#40049=DIRECTION('center_axis',(-1.,0.,0.));
#40050=DIRECTION('ref_axis',(0.,1.,0.));
#40051=DIRECTION('center_axis',(-1.,0.,0.));
#40052=DIRECTION('ref_axis',(0.,1.,0.));
#40053=DIRECTION('center_axis',(1.,0.,0.));
#40054=DIRECTION('ref_axis',(0.,0.,-1.));
#40055=DIRECTION('center_axis',(1.,0.,0.));
#40056=DIRECTION('ref_axis',(0.,1.,0.));
#40057=DIRECTION('center_axis',(1.,0.,0.));
#40058=DIRECTION('ref_axis',(0.,1.,0.));
#40059=DIRECTION('center_axis',(-1.,0.,0.));
#40060=DIRECTION('ref_axis',(0.,1.,-1.13773497930895E-12));
#40061=DIRECTION('center_axis',(1.,0.,0.));
#40062=DIRECTION('ref_axis',(0.,1.,-1.13773497930895E-12));
#40063=DIRECTION('center_axis',(1.,0.,0.));
#40064=DIRECTION('ref_axis',(0.,1.,0.));
#40065=DIRECTION('center_axis',(1.,0.,0.));
#40066=DIRECTION('ref_axis',(0.,0.,-1.));
#40067=DIRECTION('',(-1.,0.,0.));
#40068=DIRECTION('center_axis',(1.,0.,0.));
#40069=DIRECTION('ref_axis',(0.,0.,-1.));
#40070=DIRECTION('center_axis',(1.,0.,0.));
#40071=DIRECTION('ref_axis',(0.,1.,0.));
#40072=DIRECTION('',(-0.371390676354103,0.92847669088526,1.13705600757556E-16));
#40073=DIRECTION('center_axis',(1.,0.,0.));
#40074=DIRECTION('ref_axis',(0.,0.603448580913459,-0.797401912584571));
#40075=DIRECTION('center_axis',(-1.,0.,0.));
#40076=DIRECTION('ref_axis',(0.,1.,0.));
#40077=DIRECTION('center_axis',(-1.,0.,0.));
#40078=DIRECTION('ref_axis',(0.,1.,0.));
#40079=DIRECTION('center_axis',(1.,0.,0.));
#40080=DIRECTION('ref_axis',(0.,0.,-1.));
#40081=DIRECTION('',(-0.707106781186546,-0.707106781186549,-8.65956056235495E-17));
#40082=DIRECTION('center_axis',(1.,0.,0.));
#40083=DIRECTION('ref_axis',(0.,0.,-1.));
#40084=DIRECTION('center_axis',(0.,0.,1.));
#40085=DIRECTION('ref_axis',(1.,0.,0.));
#40086=DIRECTION('center_axis',(1.22464679914735E-16,-1.,0.));
#40087=DIRECTION('ref_axis',(-1.,-1.22464679914735E-16,0.));
#70391=CARTESIAN_POINT('',(0.,0.,0.));
#70392=CARTESIAN_POINT('Origin',(10.45,0.,0.));
#70393=CARTESIAN_POINT('',(-17.3782112878558,-4.95980655637472,0.00244053657197804));
#70394=CARTESIAN_POINT('',(-17.4835887121441,-4.95607622547182,0.00160660521679311));
#70395=CARTESIAN_POINT('',(10.45,-4.954,-6.06690024297599E-16));
#70396=CARTESIAN_POINT('',(-17.6184,2.11971615148618,4.48120317648902));
#70397=CARTESIAN_POINT('Ctrl Pts',(-17.3782112878558,-4.95980655637472,
0.00244053657197804));
#70398=CARTESIAN_POINT('Ctrl Pts',(-17.3820545464539,-4.96088006034128,
0.161384750450865));
#70399=CARTESIAN_POINT('Ctrl Pts',(-17.385897805052,-4.95392904526419,0.320240835458518));
#70400=CARTESIAN_POINT('Ctrl Pts',(-17.3897410636502,-4.93865078209299,
0.478296092362431));
#70401=CARTESIAN_POINT('Ctrl Pts',(-17.4294963877892,-4.78060981525614,
2.11324669733806));
#70402=CARTESIAN_POINT('Ctrl Pts',(-17.4692517119283,-3.73153769965044,
3.66250719470835));
#70403=CARTESIAN_POINT('Ctrl Pts',(-17.5090070360673,-2.27033074934917,
4.41321306777073));
#70404=CARTESIAN_POINT('Ctrl Pts',(-17.5454713573782,-0.93008460895497,
5.10177443050972));
#70405=CARTESIAN_POINT('Ctrl Pts',(-17.5819356786891,0.756886402755601,
5.11851985816336));
#70406=CARTESIAN_POINT('Ctrl Pts',(-17.6184,2.1230376970401,4.48323345254421));
#70407=CARTESIAN_POINT('',(-17.6184,-2.11639460593172,4.47917290043409));
#70408=CARTESIAN_POINT('Origin',(-17.6184,0.,0.));
#70409=CARTESIAN_POINT('Ctrl Pts',(-17.6184,-2.11639460593172,4.47917290043409));
#70410=CARTESIAN_POINT('Ctrl Pts',(-17.5985223379305,-2.8622965430514,4.1267366646904));
#70411=CARTESIAN_POINT('Ctrl Pts',(-17.578644675861,-3.51256081769737,3.58433682878205));
#70412=CARTESIAN_POINT('Ctrl Pts',(-17.5587670137914,-4.00026620400954,
2.91790966066576));
#70413=CARTESIAN_POINT('Ctrl Pts',(-17.5388893517219,-4.48797159032172,
2.25148249254946));
#70414=CARTESIAN_POINT('Ctrl Pts',(-17.5190116896524,-4.81311808830011,
1.46102799222521));
#70415=CARTESIAN_POINT('Ctrl Pts',(-17.4991340275828,-4.91815019368021,
0.644120288275306));
#70416=CARTESIAN_POINT('Ctrl Pts',(-17.4939522557699,-4.94553029508281,
0.431166204476148));
#70417=CARTESIAN_POINT('Ctrl Pts',(-17.488770483957,-4.95795236637979,0.216414474409738));
#70418=CARTESIAN_POINT('Ctrl Pts',(-17.4835887121441,-4.95607622547182,
0.00160660521679311));
#70419=CARTESIAN_POINT('Origin',(10.45,0.,0.));
#70420=CARTESIAN_POINT('',(-16.6282112878558,-4.94754111804637,0.00290217464796599));
#70421=CARTESIAN_POINT('',(-16.7335887121441,-4.9466458171129,0.00209310800741799));
#70422=CARTESIAN_POINT('',(10.45,-4.954,-6.06690024297599E-16));
#70423=CARTESIAN_POINT('Ctrl Pts',(-16.6282112878558,-4.94754111804637,
0.00290217464796599));
#70424=CARTESIAN_POINT('Ctrl Pts',(-16.6435226016196,-4.95093641568814,
0.640262719595125));
#70425=CARTESIAN_POINT('Ctrl Pts',(-16.6588339153834,-4.83671955758367,
1.27645309649682));
#70426=CARTESIAN_POINT('Ctrl Pts',(-16.6741452291472,-4.59927446317422,
1.86273610510442));
#70427=CARTESIAN_POINT('Ctrl Pts',(-16.7139005532862,-3.9827560612203,3.38500071309082));
#70428=CARTESIAN_POINT('Ctrl Pts',(-16.7536558774253,-2.53547700879338,
4.57080771208592));
#70429=CARTESIAN_POINT('Ctrl Pts',(-16.7934112015644,-0.921670863964594,
4.87584539304171));
#70430=CARTESIAN_POINT('Ctrl Pts',(-16.8331665257034,0.692135280864182,
5.18088307399749));
#70431=CARTESIAN_POINT('Ctrl Pts',(-16.8729218498425,2.47246851809482,4.60515143691398));
#70432=CARTESIAN_POINT('Ctrl Pts',(-16.9126771739815,3.6020671352805,3.41297586664233));
#70433=CARTESIAN_POINT('Ctrl Pts',(-16.9524324981206,4.73166575246619,2.22080029637068));
#70434=CARTESIAN_POINT('Ctrl Pts',(-16.9921878222596,5.21052974960693,0.412180792910897));
#70435=CARTESIAN_POINT('Ctrl Pts',(-17.0319431463987,4.81906279122762,-1.18287422808977));
#70436=CARTESIAN_POINT('Ctrl Pts',(-17.0716984705377,4.4275958328483,-2.77792924909044));
#70437=CARTESIAN_POINT('Ctrl Pts',(-17.1114537946768,3.16579791894893,-4.15941978763199));
#70438=CARTESIAN_POINT('Ctrl Pts',(-17.1512091188158,1.61244706364669,-4.69300265883637));
#70439=CARTESIAN_POINT('Ctrl Pts',(-17.1909644429549,0.0590962083444407,
-5.22658553004074));
#70440=CARTESIAN_POINT('Ctrl Pts',(-17.230719767094,-1.78580758836068,-4.91226073390795));
#70441=CARTESIAN_POINT('Ctrl Pts',(-17.270475091233,-3.07475457767925,-3.89477797955106));
#70442=CARTESIAN_POINT('Ctrl Pts',(-17.3063871567739,-4.23909544928865,
-2.97565813453576));
#70443=CARTESIAN_POINT('Ctrl Pts',(-17.3422992223148,-4.94977555174121,
-1.48276137748618));
#70444=CARTESIAN_POINT('Ctrl Pts',(-17.3782112878558,-4.95980655637472,
0.00244053657197804));
#70445=CARTESIAN_POINT('Ctrl Pts',(-17.4835887121441,-4.95607622547182,
0.00160660521679311));
#70446=CARTESIAN_POINT('Ctrl Pts',(-17.449015159818,-4.94355833425728,-1.43162345078241));
#70447=CARTESIAN_POINT('Ctrl Pts',(-17.4144416074918,-4.29451879539502,
-2.86735268421774));
#70448=CARTESIAN_POINT('Ctrl Pts',(-17.3798680551657,-3.2049418960497,-3.78830498722671));
#70449=CARTESIAN_POINT('Ctrl Pts',(-17.3401127310266,-1.95206274729191,
-4.8472866324265));
#70450=CARTESIAN_POINT('Ctrl Pts',(-17.3003574068876,-0.116697809409273,
-5.22562170042369));
#70451=CARTESIAN_POINT('Ctrl Pts',(-17.2606020827485,1.45422416551184,-4.74511164472302));
#70452=CARTESIAN_POINT('Ctrl Pts',(-17.2208467586095,3.02514614043297,-4.26460158902235));
#70453=CARTESIAN_POINT('Ctrl Pts',(-17.1810914344704,4.33162515239257,-2.92524640962383));
#70454=CARTESIAN_POINT('Ctrl Pts',(-17.1413361103314,4.77626420482008,-1.34400114385843));
#70455=CARTESIAN_POINT('Ctrl Pts',(-17.1015807861923,5.22090325724759,0.237244121906955));
#70456=CARTESIAN_POINT('Ctrl Pts',(-17.0618254620532,4.80370235014301,2.06037947403921));
#70457=CARTESIAN_POINT('Ctrl Pts',(-17.0220701379142,3.71497358052998,3.28973911961942));
#70458=CARTESIAN_POINT('Ctrl Pts',(-16.9823148137751,2.62624481091696,4.51909876519962));
#70459=CARTESIAN_POINT('Ctrl Pts',(-16.9425594896361,0.865988178795493,
5.15468270422777));
#70460=CARTESIAN_POINT('Ctrl Pts',(-16.902804165497,-0.757234442789558,
4.90416721199705));
#70461=CARTESIAN_POINT('Ctrl Pts',(-16.863048841358,-2.38045706437461,4.65365171976634));
#70462=CARTESIAN_POINT('Ctrl Pts',(-16.8232935172189,-3.86664567542324,
3.51703679627675));
#70463=CARTESIAN_POINT('Ctrl Pts',(-16.7835381930799,-4.53397860724609,
2.01633239046266));
#70464=CARTESIAN_POINT('Ctrl Pts',(-16.7668883661013,-4.81346262838259,
1.38782616534876));
#70465=CARTESIAN_POINT('Ctrl Pts',(-16.7502385391227,-4.9493196071233,0.695458753409945));
#70466=CARTESIAN_POINT('Ctrl Pts',(-16.7335887121441,-4.9466458171129,0.00209310800741799));
#70467=CARTESIAN_POINT('Origin',(10.45,0.,0.));
#70468=CARTESIAN_POINT('',(-15.8782112878558,-4.94963099410875,-0.0039542947945842));
#70469=CARTESIAN_POINT('',(-15.9835887121441,-4.95109393512768,-0.00433887822852018));
#70470=CARTESIAN_POINT('',(10.45,-4.954,-6.06690024297599E-16));
#70471=CARTESIAN_POINT('Ctrl Pts',(-15.8782112878558,-4.94963099410875,
-0.0039542947945842));
#70472=CARTESIAN_POINT('Ctrl Pts',(-15.9049906567853,-4.94133152292927,
1.10960955975419));
#70473=CARTESIAN_POINT('Ctrl Pts',(-15.9317700257147,-4.56971376715886,
2.22819216688661));
#70474=CARTESIAN_POINT('Ctrl Pts',(-15.9585493946442,-3.88008016453715,
3.09324852781628));
#70475=CARTESIAN_POINT('Ctrl Pts',(-15.9983047187833,-2.85628429086991,
4.37746833590356));
#70476=CARTESIAN_POINT('Ctrl Pts',(-16.0380600429223,-1.13161646218319,
5.10294417703389));
#70477=CARTESIAN_POINT('Ctrl Pts',(-16.0778153670614,0.502316997631763,
4.93668818591454));
#70478=CARTESIAN_POINT('Ctrl Pts',(-16.1175706912004,2.13625045744672,4.77043219479518));
#70479=CARTESIAN_POINT('Ctrl Pts',(-16.1573260153395,3.67944954838991,3.71244437142615));
#70480=CARTESIAN_POINT('Ctrl Pts',(-16.1970813394785,4.4235971230862,2.24833338328714));
#70481=CARTESIAN_POINT('Ctrl Pts',(-16.2368366636176,5.16774469778249,0.784222395148121));
#70482=CARTESIAN_POINT('Ctrl Pts',(-16.2765919877566,5.11284075623187,-1.08601175776088));
#70483=CARTESIAN_POINT('Ctrl Pts',(-16.3163473118957,4.28408994860642,-2.50395072399457));
#70484=CARTESIAN_POINT('Ctrl Pts',(-16.3561026360347,3.45533914098097,-3.92188969022827));
#70485=CARTESIAN_POINT('Ctrl Pts',(-16.3958579601738,1.85274146728066,-4.88753346978664));
#70486=CARTESIAN_POINT('Ctrl Pts',(-16.4356132843129,0.211867270152115,
-4.95765464081455));
#70487=CARTESIAN_POINT('Ctrl Pts',(-16.4753686084519,-1.42900692697643,
-5.02777581184246));
#70488=CARTESIAN_POINT('Ctrl Pts',(-16.515123932591,-3.10815764753321,-4.2023743743399));
#70489=CARTESIAN_POINT('Ctrl Pts',(-16.55487925673,-4.05485413207113,-2.86031254709977));
#70490=CARTESIAN_POINT('Ctrl Pts',(-16.5793232671053,-4.63694116547867,
-2.03513066417666));
#70491=CARTESIAN_POINT('Ctrl Pts',(-16.6037672774805,-4.94212063669103,
-1.01462303669556));
#70492=CARTESIAN_POINT('Ctrl Pts',(-16.6282112878558,-4.94754111804637,
0.00290217464796599));
#70493=CARTESIAN_POINT('Ctrl Pts',(-16.7335887121441,-4.9466458171129,0.00209310800741799));
#70494=CARTESIAN_POINT('Ctrl Pts',(-16.7104832149836,-4.94293531323964,
-0.960112563655588));
#70495=CARTESIAN_POINT('Ctrl Pts',(-16.6873777178232,-4.67244225281239,
-1.9242406333381));
#70496=CARTESIAN_POINT('Ctrl Pts',(-16.6642722206627,-4.14878639781746,
-2.72229021995792));
#70497=CARTESIAN_POINT('Ctrl Pts',(-16.6245168965236,-3.24778400396889,
-4.0954145364258));
#70498=CARTESIAN_POINT('Ctrl Pts',(-16.5847615723846,-1.59730196367469,
-4.97686928122295));
#70499=CARTESIAN_POINT('Ctrl Pts',(-16.5450062482455,0.0450125217207269,
-4.96198750357192));
#70500=CARTESIAN_POINT('Ctrl Pts',(-16.5052509241065,1.68732700711615,-4.9471057259209));
#70501=CARTESIAN_POINT('Ctrl Pts',(-16.4654955999674,3.32147393761279,-4.03588742582169));
#70502=CARTESIAN_POINT('Ctrl Pts',(-16.4257402758284,4.1974416845951,-2.64661961403913));
#70503=CARTESIAN_POINT('Ctrl Pts',(-16.3859849516893,5.07340943157741,-1.25735180225659));
#70504=CARTESIAN_POINT('Ctrl Pts',(-16.3462296275503,5.1911979950454,0.609965521209312));
#70505=CARTESIAN_POINT('Ctrl Pts',(-16.3064743034112,4.49671841016726,2.09827407943552));
#70506=CARTESIAN_POINT('Ctrl Pts',(-16.2667189792721,3.80223882528911,3.58658263766173));
#70507=CARTESIAN_POINT('Ctrl Pts',(-16.2269636551331,2.29549109206482,4.69588243064825));
#70508=CARTESIAN_POINT('Ctrl Pts',(-16.187208330994,0.668072464940804,4.91700184303135));
#70509=CARTESIAN_POINT('Ctrl Pts',(-16.147453006855,-0.95934616218321,5.13812125541445));
#70510=CARTESIAN_POINT('Ctrl Pts',(-16.1076976827159,-2.70743568320695,
4.47106028719414));
#70511=CARTESIAN_POINT('Ctrl Pts',(-16.0679423585769,-3.77384519331976,
3.22200078380499));
#70512=CARTESIAN_POINT('Ctrl Pts',(-16.0398244764326,-4.52808824308058,
2.33857425747055));
#70513=CARTESIAN_POINT('Ctrl Pts',(-16.0117065942884,-4.94133066842602,
1.16401133176273));
#70514=CARTESIAN_POINT('Ctrl Pts',(-15.9835887121441,-4.95109393512768,
-0.00433887822852018));
#70515=CARTESIAN_POINT('Origin',(10.45,0.,0.));
#70516=CARTESIAN_POINT('',(-15.1282112878558,-4.96185087269624,-0.00115664513161418));
#70517=CARTESIAN_POINT('',(-15.2335887121441,-4.9621737197389,-0.000131629710198743));
#70518=CARTESIAN_POINT('',(10.45,-4.954,-6.06690024297599E-16));
#70519=CARTESIAN_POINT('Ctrl Pts',(-15.1282112878558,-4.96185087269624,
-0.00115664513161418));
#70520=CARTESIAN_POINT('Ctrl Pts',(-15.1664587119509,-4.9568780428024,1.57919865857407));
#70521=CARTESIAN_POINT('Ctrl Pts',(-15.2047061360461,-4.13630119926,3.16399456753119));
#70522=CARTESIAN_POINT('Ctrl Pts',(-15.2429535601412,-2.8407735100365,4.06856442895952));
#70523=CARTESIAN_POINT('Ctrl Pts',(-15.2827088842803,-1.4941697992068,5.00879684717528));
#70524=CARTESIAN_POINT('Ctrl Pts',(-15.3224642084193,0.365572742064798,
5.21411026979585));
#70525=CARTESIAN_POINT('Ctrl Pts',(-15.3622195325584,1.88484852979504,4.59026760960427));
#70526=CARTESIAN_POINT('Ctrl Pts',(-15.4019748566974,3.40412431752528,3.9664249494127));
#70527=CARTESIAN_POINT('Ctrl Pts',(-15.4417301808365,4.58293335171415,2.513426206409));
#70528=CARTESIAN_POINT('Ctrl Pts',(-15.4814855049755,4.88021251791395,0.898185164615993));
#70529=CARTESIAN_POINT('Ctrl Pts',(-15.5212408291146,5.17749168411375,-0.717055877177018));
#70530=CARTESIAN_POINT('Ctrl Pts',(-15.5609961532537,4.59324098232445,-2.49453921775932));
#70531=CARTESIAN_POINT('Ctrl Pts',(-15.6007514773927,3.39562647972561,-3.61841556400534));
#70532=CARTESIAN_POINT('Ctrl Pts',(-15.6405068015318,2.19801197712677,-4.74229191025135));
#70533=CARTESIAN_POINT('Ctrl Pts',(-15.6802621256708,0.387033673718383,
-5.21256126216107));
#70534=CARTESIAN_POINT('Ctrl Pts',(-15.7200174498099,-1.20608535228746,
-4.81337397416404));
#70535=CARTESIAN_POINT('Ctrl Pts',(-15.7597727739489,-2.7992043782933,-4.41418668616701));
#70536=CARTESIAN_POINT('Ctrl Pts',(-15.799528098088,-4.1744641268966,-3.14554275826323));
#70537=CARTESIAN_POINT('Ctrl Pts',(-15.839283422227,-4.70063204187437,-1.58973890678923));
#70538=CARTESIAN_POINT('Ctrl Pts',(-15.8522593774366,-4.87237083272382,
-1.08193167520928));
#70539=CARTESIAN_POINT('Ctrl Pts',(-15.8652353326462,-4.9536525065862,-0.543532159294824));
#70540=CARTESIAN_POINT('Ctrl Pts',(-15.8782112878558,-4.94963099410875,
-0.0039542947945842));
#70541=CARTESIAN_POINT('Ctrl Pts',(-15.9835887121441,-4.95109393512768,
-0.00433887822852018));
#70542=CARTESIAN_POINT('Ctrl Pts',(-15.9719512701493,-4.95513476044081,
-0.487896200526849));
#70543=CARTESIAN_POINT('Ctrl Pts',(-15.9603138281545,-4.89006080214088,
-0.970389303042811));
#70544=CARTESIAN_POINT('Ctrl Pts',(-15.9486763861597,-4.75144255109529,
-1.43073717552031));
#70545=CARTESIAN_POINT('Ctrl Pts',(-15.9089210620207,-4.27790089955613,
-3.00335759289846));
#70546=CARTESIAN_POINT('Ctrl Pts',(-15.8691657378816,-2.94608809727594,
-4.31754038909679));
#70547=CARTESIAN_POINT('Ctrl Pts',(-15.8294104137426,-1.36729653084616,
-4.77008526960488));
#70548=CARTESIAN_POINT('Ctrl Pts',(-15.7896550896035,0.211495035583636,
-5.22263015011297));
#70549=CARTESIAN_POINT('Ctrl Pts',(-15.7498997654644,2.03726536616302,-4.81353711493081));
#70550=CARTESIAN_POINT('Ctrl Pts',(-15.7101444413254,3.27200281351365,-3.73057727440859));
#70551=CARTESIAN_POINT('Ctrl Pts',(-15.6703891171863,4.50674026086427,-2.64761743388638));
#70552=CARTESIAN_POINT('Ctrl Pts',(-15.6306337930473,5.15044482498614,-0.890790788024123));
#70553=CARTESIAN_POINT('Ctrl Pts',(-15.5908784689082,4.90766119087328,0.733535065939904));
#70554=CARTESIAN_POINT('Ctrl Pts',(-15.5511231447692,4.66487755676042,2.35786091990394));
#70555=CARTESIAN_POINT('Ctrl Pts',(-15.5113678206301,3.53560572441281,3.84968598196975));
#70556=CARTESIAN_POINT('Ctrl Pts',(-15.471612496491,2.0381718980976,4.52427528766509));
#70557=CARTESIAN_POINT('Ctrl Pts',(-15.431857172352,0.54073807178239,5.19886459336044));
#70558=CARTESIAN_POINT('Ctrl Pts',(-15.3921018482129,-1.32485774850043,
5.05621814268532));
#70559=CARTESIAN_POINT('Ctrl Pts',(-15.3523465240739,-2.70232349767177,
4.16180955481897));
#70560=CARTESIAN_POINT('Ctrl Pts',(-15.312760586764,-4.07392023280467,3.27121180331023));
#70561=CARTESIAN_POINT('Ctrl Pts',(-15.273174649454,-4.96153761937937,1.63524438301617));
#70562=CARTESIAN_POINT('Ctrl Pts',(-15.2335887121441,-4.9621737197389,-0.000131629710198743));
#70563=CARTESIAN_POINT('Origin',(10.45,0.,0.));
#70564=CARTESIAN_POINT('',(-14.3782112878558,-4.95311312927936,0.00456086744855991));
#70565=CARTESIAN_POINT('',(-14.4835887121441,-4.95148814634774,0.00440770772639709));
#70566=CARTESIAN_POINT('',(10.45,-4.954,-6.06690024297599E-16));
#70567=CARTESIAN_POINT('Ctrl Pts',(-14.3782112878558,-4.95311312927936,
0.00456086744855991));
#70568=CARTESIAN_POINT('Ctrl Pts',(-14.3881714429775,-4.95686762720455,
0.417995751918769));
#70569=CARTESIAN_POINT('Ctrl Pts',(-14.3981315980993,-4.90944555725122,
0.830581339778542));
#70570=CARTESIAN_POINT('Ctrl Pts',(-14.4080917532211,-4.80751544623729,
1.22922980986666));
#70571=CARTESIAN_POINT('Ctrl Pts',(-14.4478470773601,-4.40066790688175,
2.82040976159881));
#70572=CARTESIAN_POINT('Ctrl Pts',(-14.4876024014992,-3.12542206198846,
4.18954963958238));
#70573=CARTESIAN_POINT('Ctrl Pts',(-14.5273577256382,-1.56710463410095,
4.70822617933687));
#70574=CARTESIAN_POINT('Ctrl Pts',(-14.5671130497773,-0.00878720621342921,
5.22690271909136));
#70575=CARTESIAN_POINT('Ctrl Pts',(-14.6068683739163,1.83260180466831,4.89511592061677));
#70576=CARTESIAN_POINT('Ctrl Pts',(-14.6466236980554,3.11188090056794,3.86515303077406));
#70577=CARTESIAN_POINT('Ctrl Pts',(-14.6863790221945,4.39115999646756,2.83519014093136));
#70578=CARTESIAN_POINT('Ctrl Pts',(-14.7261343463335,5.10832917738507,1.10705115972054));
#70579=CARTESIAN_POINT('Ctrl Pts',(-14.7658896704726,4.93421404221,-0.52606318972133));
#70580=CARTESIAN_POINT('Ctrl Pts',(-14.8056449946116,4.76009890703493,-2.15917753916319));
#70581=CARTESIAN_POINT('Ctrl Pts',(-14.8454003187507,3.6946994557673,-3.69726725683611));
#70582=CARTESIAN_POINT('Ctrl Pts',(-14.8851556428897,2.22702474783851,-4.43436257622917));
#70583=CARTESIAN_POINT('Ctrl Pts',(-14.9249109670288,0.759350039909706,
-5.17145789562223));
#70584=CARTESIAN_POINT('Ctrl Pts',(-14.9646662911678,-1.11059992468025,
-5.10755881673543));
#70585=CARTESIAN_POINT('Ctrl Pts',(-15.0044216153069,-2.52453442237049,
-4.27199445713027));
#70586=CARTESIAN_POINT('Ctrl Pts',(-15.0441769394459,-3.93846892006073,
-3.43643009752511));
#70587=CARTESIAN_POINT('Ctrl Pts',(-15.083932263585,-4.89638795085125,-1.8292004572016));
#70588=CARTESIAN_POINT('Ctrl Pts',(-15.1236875877241,-4.95861502605261,
-0.188009930134371));
#70589=CARTESIAN_POINT('Ctrl Pts',(-15.125195487768,-4.96097526864804,-0.125760374347325));
#70590=CARTESIAN_POINT('Ctrl Pts',(-15.1267033878119,-4.96204692591009,
-0.0634619608025481));
#70591=CARTESIAN_POINT('Ctrl Pts',(-15.1282112878558,-4.96185087269624,
-0.00115664513161418));
#70592=CARTESIAN_POINT('Ctrl Pts',(-15.2335887121441,-4.9621737197389,-0.000131629710198743));
#70593=CARTESIAN_POINT('Ctrl Pts',(-15.233419325315,-4.9621764415899,-0.00712934597106935));
#70594=CARTESIAN_POINT('Ctrl Pts',(-15.2332499384858,-4.96216292322238,
-0.0141270514035398));
#70595=CARTESIAN_POINT('Ctrl Pts',(-15.2330805516567,-4.96213313306282,
-0.0211246875646397));
#70596=CARTESIAN_POINT('Ctrl Pts',(-15.1933252275177,-4.95514134122268,
-1.66347961702442));
#70597=CARTESIAN_POINT('Ctrl Pts',(-15.1535699033786,-4.05182207948253,
-3.30201875088644));
#70598=CARTESIAN_POINT('Ctrl Pts',(-15.1138145792396,-2.66679105273963,
-4.18466687585192));
#70599=CARTESIAN_POINT('Ctrl Pts',(-15.0740592551005,-1.28176002599674,
-5.0673150008174));
#70600=CARTESIAN_POINT('Ctrl Pts',(-15.0343039309615,0.584982765748895,
-5.19407211688634));
#70601=CARTESIAN_POINT('Ctrl Pts',(-14.9945486068224,2.07661868124458,-4.5067578339041));
#70602=CARTESIAN_POINT('Ctrl Pts',(-14.9547932826833,3.56825459674025,-3.81944355092187));
#70603=CARTESIAN_POINT('Ctrl Pts',(-14.9150379585443,4.68478363598596,-2.31805786888846));
#70604=CARTESIAN_POINT('Ctrl Pts',(-14.8752826344052,4.91372869508898,-0.691723712375354));
#70605=CARTESIAN_POINT('Ctrl Pts',(-14.8355273102662,5.142673754192,0.934610444137763));
#70606=CARTESIAN_POINT('Ctrl Pts',(-14.7957719861271,4.48403483315231,2.68589307513059));
#70607=CARTESIAN_POINT('Ctrl Pts',(-14.7560166619881,3.24012145917152,3.75830071895447));
#70608=CARTESIAN_POINT('Ctrl Pts',(-14.716261337849,1.99620808519072,4.83070836277836));
#70609=CARTESIAN_POINT('Ctrl Pts',(-14.6765060137099,0.167020258268824,
5.22424101943332));
#70610=CARTESIAN_POINT('Ctrl Pts',(-14.6367506895709,-1.40786076327547,
4.75827063427213));
#70611=CARTESIAN_POINT('Ctrl Pts',(-14.5969953654318,-2.98274178481976,
4.29230024911094));
#70612=CARTESIAN_POINT('Ctrl Pts',(-14.5572400412928,-4.30331600098644,
2.96682682213362));
#70613=CARTESIAN_POINT('Ctrl Pts',(-14.5174847171537,-4.76345136071661,
1.3902310961853));
#70614=CARTESIAN_POINT('Ctrl Pts',(-14.5061860488172,-4.89422420516193,
0.942154452513536));
#70615=CARTESIAN_POINT('Ctrl Pts',(-14.4948873804806,-4.95549718832007,
0.473794014340802));
#70616=CARTESIAN_POINT('Ctrl Pts',(-14.4835887121441,-4.95148814634774,
0.00440770772639709));
#70617=CARTESIAN_POINT('Origin',(10.45,0.,0.));
#70618=CARTESIAN_POINT('',(-13.6282112878558,-4.94601675291934,-0.00105820789737976));
#70619=CARTESIAN_POINT('',(-13.7335887121441,-4.94651950398206,-0.00192876730649404));
#70620=CARTESIAN_POINT('',(10.45,-4.954,-6.06690024297599E-16));
#70621=CARTESIAN_POINT('Ctrl Pts',(-13.6282112878558,-4.94601675291934,
-0.00105820789737976));
#70622=CARTESIAN_POINT('Ctrl Pts',(-13.6496394981432,-4.944317184649,0.891622090528033));
#70623=CARTESIAN_POINT('Ctrl Pts',(-13.6710677084306,-4.71383143873792,
1.78512061197043));
#70624=CARTESIAN_POINT('Ctrl Pts',(-13.6924959187181,-4.25979883424053,
2.54505885641213));
#70625=CARTESIAN_POINT('Ctrl Pts',(-13.7322512428571,-3.41744134757363,
3.95495687534098));
#70626=CARTESIAN_POINT('Ctrl Pts',(-13.7720065669962,-1.80562152001957,
4.90513202435166));
#70627=CARTESIAN_POINT('Ctrl Pts',(-13.8117618911352,-0.164150596859296,
4.95946219587632));
#70628=CARTESIAN_POINT('Ctrl Pts',(-13.8515172152743,1.47732032630098,5.01379236740099));
#70629=CARTESIAN_POINT('Ctrl Pts',(-13.8912725394134,3.14844234506749,4.17227756143964));
#70630=CARTESIAN_POINT('Ctrl Pts',(-13.9310278635524,4.08218502554369,2.82116573564903));
#70631=CARTESIAN_POINT('Ctrl Pts',(-13.9707831876915,5.01592770601988,1.47005390985843));
#70632=CARTESIAN_POINT('Ctrl Pts',(-14.0105385118305,5.21229104820577,-0.390654935761419));
#70633=CARTESIAN_POINT('Ctrl Pts',(-14.0502938359696,4.58114599036622,-1.90691166701902));
#70634=CARTESIAN_POINT('Ctrl Pts',(-14.0900491601086,3.95000093252669,-3.42316839827661));
#70635=CARTESIAN_POINT('Ctrl Pts',(-14.1298044842477,2.49134747466172,-4.59497301517194));
#70636=CARTESIAN_POINT('Ctrl Pts',(-14.1695598083867,0.874694834058384,
-4.88447741707956));
#70637=CARTESIAN_POINT('Ctrl Pts',(-14.2093151325258,-0.741957806544973,
-5.17398181898719));
#70638=CARTESIAN_POINT('Ctrl Pts',(-14.2490704566648,-2.51660962988671,
-4.58118600590708));
#70639=CARTESIAN_POINT('Ctrl Pts',(-14.2888257808039,-3.63471092464868,
-3.37817808662665));
#70640=CARTESIAN_POINT('Ctrl Pts',(-14.3186209498212,-4.47268716499728,
-2.47656742037406));
#70641=CARTESIAN_POINT('Ctrl Pts',(-14.3484161188385,-4.94188178811161,
-1.2322032300823));
#70642=CARTESIAN_POINT('Ctrl Pts',(-14.3782112878558,-4.95311312927936,
0.00456086744855991));
#70643=CARTESIAN_POINT('Ctrl Pts',(-14.4835887121441,-4.95148814634774,
0.00440770772639709));
#70644=CARTESIAN_POINT('Ctrl Pts',(-14.4551320563416,-4.94139103365212,
-1.17778157050275));
#70645=CARTESIAN_POINT('Ctrl Pts',(-14.4266754005391,-4.51719240613835,
-2.3664782092933));
#70646=CARTESIAN_POINT('Ctrl Pts',(-14.3982187447366,-3.74627668568719,
-3.25401634256688));
#70647=CARTESIAN_POINT('Ctrl Pts',(-14.3584634205975,-2.66927014763396,
-4.49395003045146));
#70648=CARTESIAN_POINT('Ctrl Pts',(-14.3187080964585,-0.915560568233825,
-5.14609938130129));
#70649=CARTESIAN_POINT('Ctrl Pts',(-14.2789527723194,0.709914648923431,
-4.91113353046451));
#70650=CARTESIAN_POINT('Ctrl Pts',(-14.2391974481804,2.33538986608067,-4.67616767962773));
#70651=CARTESIAN_POINT('Ctrl Pts',(-14.1994421240413,3.83263072099504,-3.55408662710436));
#70652=CARTESIAN_POINT('Ctrl Pts',(-14.1596867999022,4.51441671742681,-2.05991579087256));
#70653=CARTESIAN_POINT('Ctrl Pts',(-14.1199314757632,5.19620271385857,-0.565744954640754));
#70654=CARTESIAN_POINT('Ctrl Pts',(-14.0801761516241,5.06253385180771,1.30051566529948));
#70655=CARTESIAN_POINT('Ctrl Pts',(-14.0404208274851,4.17476297344876,2.68226871864855));
#70656=CARTESIAN_POINT('Ctrl Pts',(-14.000665503346,3.28699209508979,4.06402177199765));
#70657=CARTESIAN_POINT('Ctrl Pts',(-13.960910179207,1.64511920042269,4.96126725875556));
#70658=CARTESIAN_POINT('Ctrl Pts',(-13.9211548550679,0.00274963038812914,
4.96217732482585));
#70659=CARTESIAN_POINT('Ctrl Pts',(-13.8813995309289,-1.63961993964642,
4.96308739089613));
#70660=CARTESIAN_POINT('Ctrl Pts',(-13.8416442067898,-3.28248618504843,
4.06766203627881));
#70661=CARTESIAN_POINT('Ctrl Pts',(-13.8018888826508,-4.17178782544991,
2.68689369032047));
#70662=CARTESIAN_POINT('Ctrl Pts',(-13.7791221591485,-4.68106513598758,
1.89616762195546));
#70663=CARTESIAN_POINT('Ctrl Pts',(-13.7563554356463,-4.94320932191155,
0.946272281090748));
#70664=CARTESIAN_POINT('Ctrl Pts',(-13.7335887121441,-4.94651950398206,
-0.00192876730649404));
#70665=CARTESIAN_POINT('Origin',(10.45,0.,0.));
#70666=CARTESIAN_POINT('',(-12.8782112878558,-4.9570073981747,-0.00414712514969162));
#70667=CARTESIAN_POINT('',(-12.9835887121441,-4.95857558632536,-0.00363955744209949));
#70668=CARTESIAN_POINT('',(10.45,-4.954,-6.06690024297599E-16));
#70669=CARTESIAN_POINT('Ctrl Pts',(-12.8782112878558,-4.9570073981747,-0.00414712514969162));
#70670=CARTESIAN_POINT('Ctrl Pts',(-12.9111075533089,-4.94478592313273,
1.35858830385809));
#70671=CARTESIAN_POINT('Ctrl Pts',(-12.944003818762,-4.3605420522345,2.73052896938504));
#70672=CARTESIAN_POINT('Ctrl Pts',(-12.9769000842151,-3.3606514679749,3.65092213030985));
#70673=CARTESIAN_POINT('Ctrl Pts',(-13.0166554083541,-2.15227800267999,
4.76322250677954));
#70674=CARTESIAN_POINT('Ctrl Pts',(-13.0564107324932,-0.336858325563938,
5.21604406791286));
#70675=CARTESIAN_POINT('Ctrl Pts',(-13.0961660566323,1.25234576260349,4.80154566589518));
#70676=CARTESIAN_POINT('Ctrl Pts',(-13.1359213807713,2.84154985077095,4.38704726387748));
#70677=CARTESIAN_POINT('Ctrl Pts',(-13.1756767049104,4.20453834998979,3.10522889870875));
#70678=CARTESIAN_POINT('Ctrl Pts',(-13.2154320290494,4.71571142480423,1.54443402214475));
#70679=CARTESIAN_POINT('Ctrl Pts',(-13.2551873531885,5.22688449961866,-0.0163608544192304));
#70680=CARTESIAN_POINT('Ctrl Pts',(-13.2949426773275,4.88624215002873,-1.85613224237847));
#70681=CARTESIAN_POINT('Ctrl Pts',(-13.3346980014666,3.85013624398807,-3.13044111804054));
#70682=CARTESIAN_POINT('Ctrl Pts',(-13.3744533256057,2.8140303379474,-4.4047499937026));
#70683=CARTESIAN_POINT('Ctrl Pts',(-13.4142086497447,1.08246087545601,-5.1135963570675));
#70684=CARTESIAN_POINT('Ctrl Pts',(-13.4539639738837,-0.549796860028286,
-4.93162590871302));
#70685=CARTESIAN_POINT('Ctrl Pts',(-13.4937192980228,-2.1820545955126,-4.74965546035853));
#70686=CARTESIAN_POINT('Ctrl Pts',(-13.5334746221619,-3.71500060398981,
-3.67686820028464));
#70687=CARTESIAN_POINT('Ctrl Pts',(-13.5732299463009,-4.44502603533852,
-2.20566412582418));
#70688=CARTESIAN_POINT('Ctrl Pts',(-13.5915570601525,-4.78156609593791,
-1.52744239941352));
#70689=CARTESIAN_POINT('Ctrl Pts',(-13.6098841740042,-4.94747035920615,
-0.764549570119788));
#70690=CARTESIAN_POINT('Ctrl Pts',(-13.6282112878558,-4.94601675291934,
-0.00105820789737976));
#70691=CARTESIAN_POINT('Ctrl Pts',(-13.7335887121441,-4.94651950398206,
-0.00192876730649404));
#70692=CARTESIAN_POINT('Ctrl Pts',(-13.7166001115073,-4.94898957224751,
-0.709479369969114));
#70693=CARTESIAN_POINT('Ctrl Pts',(-13.6996115108704,-4.80733591544937,
-1.41608655817256));
#70694=CARTESIAN_POINT('Ctrl Pts',(-13.6826229102336,-4.51669681609159,
-2.05491149081309));
#70695=CARTESIAN_POINT('Ctrl Pts',(-13.6428675860945,-3.83656713093088,
-3.5498369886889));
#70696=CARTESIAN_POINT('Ctrl Pts',(-13.6031122619555,-2.34057072520854,
-4.67357664714119));
#70697=CARTESIAN_POINT('Ctrl Pts',(-13.5633569378164,-0.715356903585403,
-4.91034376231061));
#70698=CARTESIAN_POINT('Ctrl Pts',(-13.5236016136774,0.909856918037765,
-5.14711087748003));
#70699=CARTESIAN_POINT('Ctrl Pts',(-13.4838462895383,2.66428815556175,-4.49690544936654));
#70700=CARTESIAN_POINT('Ctrl Pts',(-13.4440909653993,3.74266817014626,-3.25816609947485));
#70701=CARTESIAN_POINT('Ctrl Pts',(-13.4043356412602,4.82104818473077,-2.01942674958316));
#70702=CARTESIAN_POINT('Ctrl Pts',(-13.3645803171212,5.22337697637581,-0.192153477913265));
#70703=CARTESIAN_POINT('Ctrl Pts',(-13.3248249929821,4.76498913815175,1.3849512182294));
#70704=CARTESIAN_POINT('Ctrl Pts',(-13.285069668843,4.3066012999277,2.96205591437203));
#70705=CARTESIAN_POINT('Ctrl Pts',(-13.245314344704,2.98749683183458,4.28899203498746));
#70706=CARTESIAN_POINT('Ctrl Pts',(-13.2055590205649,1.41313318172271,4.75670747201202));
#70707=CARTESIAN_POINT('Ctrl Pts',(-13.1658036964259,-0.161230468389194,
5.22442290903659));
#70708=CARTESIAN_POINT('Ctrl Pts',(-13.1260483722868,-1.99085330051983,
4.83291766247028));
#70709=CARTESIAN_POINT('Ctrl Pts',(-13.0862930481478,-3.2359543896031,3.76188922643825));
#70710=CARTESIAN_POINT('Ctrl Pts',(-13.0520582694799,-4.30815694679576,
2.83958706317767));
#70711=CARTESIAN_POINT('Ctrl Pts',(-13.017823490812,-4.94690340106977,1.41337982358395));
#70712=CARTESIAN_POINT('Ctrl Pts',(-12.9835887121441,-4.95857558632536,
-0.00363955744209949));
#70713=CARTESIAN_POINT('Origin',(10.45,0.,0.));
#70714=CARTESIAN_POINT('',(-12.1282112878558,-4.95954504035343,0.00318967636549851));
#70715=CARTESIAN_POINT('',(-12.2335887121441,-4.95809108523107,0.00382194074085128));
#70716=CARTESIAN_POINT('',(10.45,-4.954,-6.06690024297599E-16));
#70717=CARTESIAN_POINT('Ctrl Pts',(-12.1282112878558,-4.95954504035343,
0.00318967636549851));
#70718=CARTESIAN_POINT('Ctrl Pts',(-12.1328202843355,-4.9609705376935,0.193864214572376));
#70719=CARTESIAN_POINT('Ctrl Pts',(-12.1374292808152,-4.95093040129845,
0.384387214448792));
#70720=CARTESIAN_POINT('Ctrl Pts',(-12.1420382772949,-4.92892361674062,
0.57351780366819));
#70721=CARTESIAN_POINT('Ctrl Pts',(-12.181793601434,-4.73910206725498,2.20488114102573));
#70722=CARTESIAN_POINT('Ctrl Pts',(-12.2215489255731,-3.65895183048629,
3.73264795448116));
#70723=CARTESIAN_POINT('Ctrl Pts',(-12.2613042497121,-2.18425244586393,
4.45558659926224));
#70724=CARTESIAN_POINT('Ctrl Pts',(-12.3010595738512,-0.70955306124158,
5.17852524404332));
#70725=CARTESIAN_POINT('Ctrl Pts',(-12.3408148979902,1.15969547123444,5.09663572015007));
#70726=CARTESIAN_POINT('Ctrl Pts',(-12.3805702221293,2.56552437558869,4.24750460494725));
#70727=CARTESIAN_POINT('Ctrl Pts',(-12.4203255462683,3.97135327994293,3.39837348974444));
#70728=CARTESIAN_POINT('Ctrl Pts',(-12.4600808704074,4.91376255617541,1.78200078323208));
#70729=CARTESIAN_POINT('Ctrl Pts',(-12.4998361945464,4.96019456459868,0.140287462424448));
#70730=CARTESIAN_POINT('Ctrl Pts',(-12.5395915186855,5.00662657302196,-1.50142585838318));
#70731=CARTESIAN_POINT('Ctrl Pts',(-12.5793468428246,4.15708131363603,-3.16847979348607));
#70732=CARTESIAN_POINT('Ctrl Pts',(-12.6191021669636,2.80149265219899,-4.09571112390302));
#70733=CARTESIAN_POINT('Ctrl Pts',(-12.6588574911027,1.44590399076196,-5.02294245431997));
#70734=CARTESIAN_POINT('Ctrl Pts',(-12.6986128152417,-0.415728072726164,
-5.21035118005097));
#70735=CARTESIAN_POINT('Ctrl Pts',(-12.7383681393808,-1.9289306551374,-4.57191833024815));
#70736=CARTESIAN_POINT('Ctrl Pts',(-12.7781234635198,-3.44213323754866,
-3.93348548044531));
#70737=CARTESIAN_POINT('Ctrl Pts',(-12.8178787876589,-4.60690633888303,
-2.46921105510862));
#70738=CARTESIAN_POINT('Ctrl Pts',(-12.8576341117979,-4.88862926281331,
-0.851184246537236));
#70739=CARTESIAN_POINT('Ctrl Pts',(-12.8644931704839,-4.93723543343982,
-0.572023125963481));
#70740=CARTESIAN_POINT('Ctrl Pts',(-12.8713522291698,-4.9595556453203,-0.288285222658431));
#70741=CARTESIAN_POINT('Ctrl Pts',(-12.8782112878558,-4.9570073981747,-0.00414712514969162));
#70742=CARTESIAN_POINT('Ctrl Pts',(-12.9835887121441,-4.95857558632536,
-0.00363955744209949));
#70743=CARTESIAN_POINT('Ctrl Pts',(-12.9780681666729,-4.9604577900947,-0.232141689801689));
#70744=CARTESIAN_POINT('Ctrl Pts',(-12.9725476212018,-4.94603397597445,
-0.46040490726145));
#70745=CARTESIAN_POINT('Ctrl Pts',(-12.9670270757306,-4.91449226833891,
-0.686277719308069));
#70746=CARTESIAN_POINT('Ctrl Pts',(-12.9272717515915,-4.68734971195556,
-2.31286460352462));
#70747=CARTESIAN_POINT('Ctrl Pts',(-12.8875164274525,-3.57248525315302,
-3.81548674645999));
#70748=CARTESIAN_POINT('Ctrl Pts',(-12.8477611033134,-2.08161195655509,
-4.5044536878415));
#70749=CARTESIAN_POINT('Ctrl Pts',(-12.8080057791744,-0.590738659957164,
-5.19342062922301));
#70750=CARTESIAN_POINT('Ctrl Pts',(-12.7682504550353,1.27614347443615,-5.06873236905063));
#70751=CARTESIAN_POINT('Ctrl Pts',(-12.7284951308963,2.66215182673351,-4.18761973142282));
#70752=CARTESIAN_POINT('Ctrl Pts',(-12.6887398067572,4.04816017903089,-3.30650709379501));
#70753=CARTESIAN_POINT('Ctrl Pts',(-12.6489844826182,4.95329474923234,-1.66897007871172));
#70754=CARTESIAN_POINT('Ctrl Pts',(-12.6092291584791,4.9621066626716,-0.0266238962620294));
#70755=CARTESIAN_POINT('Ctrl Pts',(-12.56947383434,4.97091857611086,1.61572228618765));
#70756=CARTESIAN_POINT('Ctrl Pts',(-12.529718510201,4.08340783278798,3.26287763600375));
#70757=CARTESIAN_POINT('Ctrl Pts',(-12.4899631860619,2.70693412451721,4.15881221132986));
#70758=CARTESIAN_POINT('Ctrl Pts',(-12.4502078619229,1.33046041624645,5.05474678665596));
#70759=CARTESIAN_POINT('Ctrl Pts',(-12.4104525377838,-0.534976256972191,
5.19946058749209));
#70760=CARTESIAN_POINT('Ctrl Pts',(-12.3706972136448,-2.0331567293218,4.52653124120398));
#70761=CARTESIAN_POINT('Ctrl Pts',(-12.3309418895057,-3.53133720167143,
3.85360189491585));
#70762=CARTESIAN_POINT('Ctrl Pts',(-12.2911865653667,-4.66226147315203,
2.36302940150349));
#70763=CARTESIAN_POINT('Ctrl Pts',(-12.2514312412276,-4.9068451651669,0.738973537185428));
#70764=CARTESIAN_POINT('Ctrl Pts',(-12.2454837315331,-4.9434355819445,0.496010155383642));
#70765=CARTESIAN_POINT('Ctrl Pts',(-12.2395362218386,-4.9601887995945,0.250059280658444));
#70766=CARTESIAN_POINT('Ctrl Pts',(-12.2335887121441,-4.95809108523107,
0.00382194074085128));
#70767=CARTESIAN_POINT('Origin',(10.45,0.,0.));
#70768=CARTESIAN_POINT('',(-11.3782112878558,-4.94702647513278,0.00247992552970894));
#70769=CARTESIAN_POINT('',(-11.4835887121441,-4.94632723583785,0.00165774955501003));
#70770=CARTESIAN_POINT('',(10.45,-4.954,-6.06690024297599E-16));
#70771=CARTESIAN_POINT('Ctrl Pts',(-11.3782112878558,-4.94702647513278,
0.00247992552970894));
#70772=CARTESIAN_POINT('Ctrl Pts',(-11.3942883395012,-4.95004983254863,
0.671894317539847));
#70773=CARTESIAN_POINT('Ctrl Pts',(-11.4103653911466,-4.82370826570512,
1.340215185172));
#70774=CARTESIAN_POINT('Ctrl Pts',(-11.426442442792,-4.56258483798423,1.95090499178823));
#70775=CARTESIAN_POINT('Ctrl Pts',(-11.466197766931,-3.91687897484982,3.46101839727712));
#70776=CARTESIAN_POINT('Ctrl Pts',(-11.5059530910701,-2.44701747748665,
4.61873302051397));
#70777=CARTESIAN_POINT('Ctrl Pts',(-11.5457084152091,-0.827653955533048,
4.8926679450662));
#70778=CARTESIAN_POINT('Ctrl Pts',(-11.5854637393482,0.791709566420588,
5.16660286961844));
#70779=CARTESIAN_POINT('Ctrl Pts',(-11.6252190634872,2.56057511296464,4.55675809548603));
#70780=CARTESIAN_POINT('Ctrl Pts',(-11.6649743876263,3.66704882329549,3.34304705595883));
#70781=CARTESIAN_POINT('Ctrl Pts',(-11.7047297117653,4.77352253362632,2.12933601643165));
#70782=CARTESIAN_POINT('Ctrl Pts',(-11.7444850359044,5.21760440774395,0.311758711509695));
#70783=CARTESIAN_POINT('Ctrl Pts',(-11.7842403600434,4.79546473796103,-1.27543272568967));
#70784=CARTESIAN_POINT('Ctrl Pts',(-11.8239956841825,4.37332506817812,-2.86262416288903));
#70785=CARTESIAN_POINT('Ctrl Pts',(-11.8637510083216,3.08496385449466,-4.21942973236582));
#70786=CARTESIAN_POINT('Ctrl Pts',(-11.9035063324606,1.52172765907916,-4.72308750949856));
#70787=CARTESIAN_POINT('Ctrl Pts',(-11.9432616565997,-0.0415085363363632,
-5.2267452866313));
#70788=CARTESIAN_POINT('Ctrl Pts',(-11.9830169807387,-1.87961971348394,
-4.87725527141997));
#70789=CARTESIAN_POINT('Ctrl Pts',(-12.0227723048778,-3.14892887095642,
-3.83503033318447));
#70790=CARTESIAN_POINT('Ctrl Pts',(-12.0579186325371,-4.27108185337152,
-2.91363477253381));
#70791=CARTESIAN_POINT('Ctrl Pts',(-12.0930649601964,-4.94867477893918,
-1.45081659714675));
#70792=CARTESIAN_POINT('Ctrl Pts',(-12.1282112878558,-4.95954504035343,
0.00318967636549851));
#70793=CARTESIAN_POINT('Ctrl Pts',(-12.2335887121441,-4.95809108523107,
0.00382194074085128));
#70794=CARTESIAN_POINT('Ctrl Pts',(-12.1997808976995,-4.94616691165269,
-1.39588091387461));
#70795=CARTESIAN_POINT('Ctrl Pts',(-12.165973083255,-4.32513137411095,-2.80484003252773));
#70796=CARTESIAN_POINT('Ctrl Pts',(-12.1321652688104,-3.2761353178338,-3.72694898580919));
#70797=CARTESIAN_POINT('Ctrl Pts',(-12.0924099446714,-2.04259866593666,
-4.81127640926203));
#70798=CARTESIAN_POINT('Ctrl Pts',(-12.0526546205323,-0.217282249593205,
-5.22239202094398));
#70799=CARTESIAN_POINT('Ctrl Pts',(-12.0128992963933,1.36200961342418,-4.77159734014955));
#70800=CARTESIAN_POINT('Ctrl Pts',(-11.9731439722542,2.94130147644158,-4.32080265935511));
#70801=CARTESIAN_POINT('Ctrl Pts',(-11.9333886481152,4.27456878613291,-3.00809768608432));
#70802=CARTESIAN_POINT('Ctrl Pts',(-11.8936333239761,4.74985347385727,-1.43600255587105));
#70803=CARTESIAN_POINT('Ctrl Pts',(-11.8538779998371,5.22513816158162,0.136092574342198));
#70804=CARTESIAN_POINT('Ctrl Pts',(-11.814122675698,4.842440227339,1.96757786149789));
#70805=CARTESIAN_POINT('Ctrl Pts',(-11.7743673515589,3.77741468570125,3.21781752991537));
#70806=CARTESIAN_POINT('Ctrl Pts',(-11.7346120274199,2.71238914406348,4.46805719833287));
#70807=CARTESIAN_POINT('Ctrl Pts',(-11.6948567032808,0.965035995030541,
5.13705124801214));
#70808=CARTESIAN_POINT('Ctrl Pts',(-11.6551013791418,-0.662624903456663,
4.91773724398744));
#70809=CARTESIAN_POINT('Ctrl Pts',(-11.6153460550027,-2.29028580194385,
4.69842323996274));
#70810=CARTESIAN_POINT('Ctrl Pts',(-11.5755907308637,-3.79825444988532,
3.59080118223412));
#70811=CARTESIAN_POINT('Ctrl Pts',(-11.5358354067246,-4.49438638783357,
2.10325993648869));
#70812=CARTESIAN_POINT('Ctrl Pts',(-11.5184198418644,-4.79934003062556,
1.45161461328974));
#70813=CARTESIAN_POINT('Ctrl Pts',(-11.5010042770043,-4.94849878013362,
0.727061193394733));
#70814=CARTESIAN_POINT('Ctrl Pts',(-11.4835887121441,-4.94632723583785,
0.00165774955501003));
#70815=CARTESIAN_POINT('Origin',(10.45,0.,0.));
#70816=CARTESIAN_POINT('',(-10.6282112878558,-4.95044820539071,-0.00419555124727688));
#70817=CARTESIAN_POINT('',(-10.7335887121441,-4.95199589610219,-0.00447753941358037));
#70818=CARTESIAN_POINT('',(10.45,-4.954,-6.06690024297599E-16));
#70819=CARTESIAN_POINT('Ctrl Pts',(-10.6282112878558,-4.95044820539071,
-0.00419555124727689));
#70820=CARTESIAN_POINT('Ctrl Pts',(-10.6557563946668,-4.94128684808288,
1.14073304265234));
#70821=CARTESIAN_POINT('Ctrl Pts',(-10.6833015014779,-4.54618067767775,
2.29136724379881));
#70822=CARTESIAN_POINT('Ctrl Pts',(-10.710846608289,-3.81983564793575,3.1673437315118));
#70823=CARTESIAN_POINT('Ctrl Pts',(-10.750601932428,-2.77151580324431,4.43162378844124));
#70824=CARTESIAN_POINT('Ctrl Pts',(-10.7903572565671,-1.03320570459301,
5.12377548511912));
#70825=CARTESIAN_POINT('Ctrl Pts',(-10.8301125807061,0.597225471344212,
4.92610722854929));
#70826=CARTESIAN_POINT('Ctrl Pts',(-10.8698679048452,2.22765664728147,4.72843897197945));
#70827=CARTESIAN_POINT('Ctrl Pts',(-10.9096232289842,3.75020890050466,3.64095076216186));
#70828=CARTESIAN_POINT('Ctrl Pts',(-10.9493785531233,4.46604402391554,2.16279020416594));
#70829=CARTESIAN_POINT('Ctrl Pts',(-10.9891338772624,5.18187914732642,0.684629646170029));
#70830=CARTESIAN_POINT('Ctrl Pts',(-11.0288892014014,5.09099714092502,-1.1842032600042));
#70831=CARTESIAN_POINT('Ctrl Pts',(-11.0686445255405,4.2351120531301,-2.58593050722946));
#70832=CARTESIAN_POINT('Ctrl Pts',(-11.1083998496795,3.37922696533518,-3.98765775445471));
#70833=CARTESIAN_POINT('Ctrl Pts',(-11.1481551738186,1.75833879614674,-4.92227934273101));
#70834=CARTESIAN_POINT('Ctrl Pts',(-11.1879104979576,0.11642108057116,-4.96081211323171));
#70835=CARTESIAN_POINT('Ctrl Pts',(-11.2276658220967,-1.52549663500446,
-4.99934488373241));
#70836=CARTESIAN_POINT('Ctrl Pts',(-11.2674211462357,-3.18844389696722,
-4.14178883645749));
#70837=CARTESIAN_POINT('Ctrl Pts',(-11.3071764703748,-4.10914241349577,
-2.78175471894954));
#70838=CARTESIAN_POINT('Ctrl Pts',(-11.3308547428684,-4.65751048320689,
-1.971718349421));
#70839=CARTESIAN_POINT('Ctrl Pts',(-11.3545330153621,-4.94257367605512,
-0.983433209217081));
#70840=CARTESIAN_POINT('Ctrl Pts',(-11.3782112878558,-4.94702647513278,
0.00247992552970894));
#70841=CARTESIAN_POINT('Ctrl Pts',(-11.4835887121441,-4.94632723583785,
0.00165774955501003));
#70842=CARTESIAN_POINT('Ctrl Pts',(-11.4612489528652,-4.94354169444311,
-0.928851162762755));
#70843=CARTESIAN_POINT('Ctrl Pts',(-11.4389091935863,-4.69175135052043,
-1.86075873782794));
#70844=CARTESIAN_POINT('Ctrl Pts',(-11.4165694343075,-4.20037955308557,
-2.64197331053946));
#70845=CARTESIAN_POINT('Ctrl Pts',(-11.3768141101684,-3.32594555243426,
-4.03220487805994));
#70846=CARTESIAN_POINT('Ctrl Pts',(-11.3370587860293,-1.69278232317659,
-4.94520757933866));
#70847=CARTESIAN_POINT('Ctrl Pts',(-11.2973034618903,-0.0504975458483708,
-4.96192113615739));
#70848=CARTESIAN_POINT('Ctrl Pts',(-11.2575481377512,1.59178723147983,-4.97863469297612));
#70849=CARTESIAN_POINT('Ctrl Pts',(-11.2177928136122,3.24319355687857,-4.0990591053349));
#70850=CARTESIAN_POINT('Ctrl Pts',(-11.1780374894731,4.14574032776884,-2.72691189778716));
#70851=CARTESIAN_POINT('Ctrl Pts',(-11.1382821653341,5.04828709865911,-1.35476469023944));
#70852=CARTESIAN_POINT('Ctrl Pts',(-11.098526841195,5.20197431504088,0.509954137214785));
#70853=CARTESIAN_POINT('Ctrl Pts',(-11.058771517056,4.53626088479547,2.01135490370464));
#70854=CARTESIAN_POINT('Ctrl Pts',(-11.0190161929169,3.87054745455005,3.51275567019453));
#70855=CARTESIAN_POINT('Ctrl Pts',(-10.9792608687779,2.38543337767741,4.65083837572004));
#70856=CARTESIAN_POINT('Ctrl Pts',(-10.9395055446388,0.762573064803474,
4.90323298288164));
#70857=CARTESIAN_POINT('Ctrl Pts',(-10.8997502204998,-0.86028724807043,
5.15562759004323));
#70858=CARTESIAN_POINT('Ctrl Pts',(-10.8599948963607,-2.62089379694564,
4.52233409884093));
#70859=CARTESIAN_POINT('Ctrl Pts',(-10.8202395722216,-3.71114352892745,
3.29402869921955));
#70860=CARTESIAN_POINT('Ctrl Pts',(-10.7913559521958,-4.5032477231154,2.40162228054039));
#70861=CARTESIAN_POINT('Ctrl Pts',(-10.7624723321699,-4.94150234199152,
1.19513729087675));
#70862=CARTESIAN_POINT('Ctrl Pts',(-10.7335887121441,-4.95199589610219,
-0.00447753941358037));
#70863=CARTESIAN_POINT('Origin',(10.45,0.,0.));
#70864=CARTESIAN_POINT('',(-9.87821128785577,-4.96209602020563,-0.000574989514468549));
#70865=CARTESIAN_POINT('',(-9.98358871214408,-4.96212480437208,0.0004625561064964));
#70866=CARTESIAN_POINT('',(10.45,-4.954,-6.06690024297599E-16));
#70867=CARTESIAN_POINT('Ctrl Pts',(-9.87821128785577,-4.96209602020563,
-0.000574989514468549));
#70868=CARTESIAN_POINT('Ctrl Pts',(-9.9172244498325,-4.9594571116787,1.61120643364145));
#70869=CARTESIAN_POINT('Ctrl Pts',(-9.95623761180925,-4.10092863156834,
3.22539966553874));
#70870=CARTESIAN_POINT('Ctrl Pts',(-9.99525077378598,-2.76195239279821,
4.12247858341363));
#70871=CARTESIAN_POINT('Ctrl Pts',(-10.035006097925,-1.39750430170163,5.03662297344527));
#70872=CARTESIAN_POINT('Ctrl Pts',(-10.0747614220641,0.465844896295108,
5.20610965909354));
#70873=CARTESIAN_POINT('Ctrl Pts',(-10.1145167462031,1.97283416829854,4.55314572962272));
#70874=CARTESIAN_POINT('Ctrl Pts',(-10.1542720703422,3.479823440302,3.9001818001519));
#70875=CARTESIAN_POINT('Ctrl Pts',(-10.1940273944813,4.63045278631214,2.42476725556195));
#70876=CARTESIAN_POINT('Ctrl Pts',(-10.2337827186203,4.8965933703576,0.804104505744015));
#70877=CARTESIAN_POINT('Ctrl Pts',(-10.2735380427594,5.16273395440306,-0.8165582440739));
#70878=CARTESIAN_POINT('Ctrl Pts',(-10.3132933668984,4.54438577648385,-2.58246919911981));
#70879=CARTESIAN_POINT('Ctrl Pts',(-10.3530486910375,3.32536525807565,-3.68309063032276));
#70880=CARTESIAN_POINT('Ctrl Pts',(-10.3928040151765,2.10634473966745,-4.7837120615257));
#70881=CARTESIAN_POINT('Ctrl Pts',(-10.4325593393156,0.286651880770261,
-5.2190439688857));
#70882=CARTESIAN_POINT('Ctrl Pts',(-10.4723146634546,-1.29849016467224,
-4.7892728031547));
#70883=CARTESIAN_POINT('Ctrl Pts',(-10.5120699875937,-2.88363221011477,
-4.3595016374237));
#70884=CARTESIAN_POINT('Ctrl Pts',(-10.5518253117327,-4.2342234421026,-3.06462739860169));
#70885=CARTESIAN_POINT('Ctrl Pts',(-10.5915806358718,-4.7303542627307,-1.49898607060017));
#70886=CARTESIAN_POINT('Ctrl Pts',(-10.6037908531998,-4.88273297612754,
-1.01812416627471));
#70887=CARTESIAN_POINT('Ctrl Pts',(-10.6160010705278,-4.95450925930186,
-0.511720428621469));
#70888=CARTESIAN_POINT('Ctrl Pts',(-10.6282112878558,-4.95044820539071,
-0.00419555124727689));
#70889=CARTESIAN_POINT('Ctrl Pts',(-10.7335887121441,-4.95199589610219,
-0.00447753941358037));
#70890=CARTESIAN_POINT('Ctrl Pts',(-10.7227170080309,-4.95594563700326,
-0.456008804298611));
#70891=CARTESIAN_POINT('Ctrl Pts',(-10.7118453039177,-4.89929249921127,
-0.90656674208727));
#70892=CARTESIAN_POINT('Ctrl Pts',(-10.7009735998045,-4.77809508776449,
-1.33903648040781));
#70893=CARTESIAN_POINT('Ctrl Pts',(-10.6612182756654,-4.3349039995313,-2.92047895237324));
#70894=CARTESIAN_POINT('Ctrl Pts',(-10.6214629515264,-3.02862890797651,
-4.26004658826364));
#70895=CARTESIAN_POINT('Ctrl Pts',(-10.5817076273873,-1.45883868899695,
-4.74288952465349));
#70896=CARTESIAN_POINT('Ctrl Pts',(-10.5419523032482,0.110951529982599,
-5.22573246104334));
#70897=CARTESIAN_POINT('Ctrl Pts',(-10.5021969791092,1.94425687638693,-4.85185069793267));
#70898=CARTESIAN_POINT('Ctrl Pts',(-10.4624416549701,3.1996061832117,-3.79285270422351));
#70899=CARTESIAN_POINT('Ctrl Pts',(-10.4226863308311,4.45495549003649,-2.73385471051433));
#70900=CARTESIAN_POINT('Ctrl Pts',(-10.382931006692,5.13234875728171,-0.989740486206656));
#70901=CARTESIAN_POINT('Ctrl Pts',(-10.343175682553,4.92086838236267,0.638956748963116));
#70902=CARTESIAN_POINT('Ctrl Pts',(-10.3034203584139,4.70938800744364,2.26765398413285));
#70903=CARTESIAN_POINT('Ctrl Pts',(-10.2636650342749,3.60903399036037,3.78093423016469));
#70904=CARTESIAN_POINT('Ctrl Pts',(-10.2239097101358,2.12485922952337,4.48421505040642));
#70905=CARTESIAN_POINT('Ctrl Pts',(-10.1841543859968,0.640684468686361,
5.18749587064816));
#70906=CARTESIAN_POINT('Ctrl Pts',(-10.1443990618577,-1.22731103590437,
5.08077726509979));
#70907=CARTESIAN_POINT('Ctrl Pts',(-10.1046437377186,-2.62173363714599,
4.21304214308846));
#70908=CARTESIAN_POINT('Ctrl Pts',(-10.0648884135796,-4.01615623838763,
3.34530702107711));
#70909=CARTESIAN_POINT('Ctrl Pts',(-10.0251330894405,-4.93700593628012,
1.71655538260276));
#70910=CARTESIAN_POINT('Ctrl Pts',(-9.98537776530148,-4.9616207495878,0.0743700265021302));
#70911=CARTESIAN_POINT('Ctrl Pts',(-9.98478141424902,-4.9619899849076,0.0497363708430052));
#70912=CARTESIAN_POINT('Ctrl Pts',(-9.98418506319655,-4.96215755304679,
0.0250996923825981));
#70913=CARTESIAN_POINT('Ctrl Pts',(-9.98358871214408,-4.96212480437208,
0.0004625561064964));
#70914=CARTESIAN_POINT('Origin',(10.45,0.,0.));
#70915=CARTESIAN_POINT('',(-9.12821128785577,-4.95217176878245,0.00449694065580375));
#70916=CARTESIAN_POINT('',(-9.23358871214408,-4.95061007082821,0.00423510493672524));
#70917=CARTESIAN_POINT('',(10.45,-4.954,-6.06690024297599E-16));
#70918=CARTESIAN_POINT('Ctrl Pts',(-9.12821128785577,-4.95217176878245,
0.00449694065580375));
#70919=CARTESIAN_POINT('Ctrl Pts',(-9.13893718085912,-4.95609640839351,
0.449932082821765));
#70920=CARTESIAN_POINT('Ctrl Pts',(-9.14966307386248,-4.90097753069107,
0.894412768863136));
#70921=CARTESIAN_POINT('Ctrl Pts',(-9.16038896686583,-4.78297000480896,
1.32151754581074));
#70922=CARTESIAN_POINT('Ctrl Pts',(-9.20014429100488,-4.34557729160315,
2.90457350614757));
#70923=CARTESIAN_POINT('Ctrl Pts',(-9.23989961514394,-3.0442200017842,4.24891913675094));
#70924=CARTESIAN_POINT('Ctrl Pts',(-9.27965493928299,-1.47620978313698,
4.73751151628769));
#70925=CARTESIAN_POINT('Ctrl Pts',(-9.31941026342205,0.0918004355102117,
5.22610389582444));
#70926=CARTESIAN_POINT('Ctrl Pts',(-9.3591655875611,1.92646358298569,4.85894302429461));
#70927=CARTESIAN_POINT('Ctrl Pts',(-9.39892091170016,3.18568527343389,3.8045525399729));
#70928=CARTESIAN_POINT('Ctrl Pts',(-9.43867623583921,4.4449069638821,2.7501620556512));
#70929=CARTESIAN_POINT('Ctrl Pts',(-9.47843155997827,5.12868719730307,1.00854195853761));
#70930=CARTESIAN_POINT('Ctrl Pts',(-9.51818688411732,4.92317680933377,-0.620919314263967));
#70931=CARTESIAN_POINT('Ctrl Pts',(-9.55794220825638,4.71766642136447,-2.25038058706556));
#70932=CARTESIAN_POINT('Ctrl Pts',(-9.59769753239543,3.62286541200492,-3.7676830355551));
#70933=CARTESIAN_POINT('Ctrl Pts',(-9.63745285653448,2.14127789754436,-4.47639806722725));
#70934=CARTESIAN_POINT('Ctrl Pts',(-9.67720818067354,0.659690383083816,
-5.18511309889938));
#70935=CARTESIAN_POINT('Ctrl Pts',(-9.7169635048126,-1.20868363647773,-5.08524071375409));
#70936=CARTESIAN_POINT('Ctrl Pts',(-9.75671882895165,-2.60627677896655,
-4.22262146565467));
#70937=CARTESIAN_POINT('Ctrl Pts',(-9.79647415309071,-4.0038699214554,-3.36000221755523));
#70938=CARTESIAN_POINT('Ctrl Pts',(-9.83622947722975,-4.93068218687153,
-1.73463610650163));
#70939=CARTESIAN_POINT('Ctrl Pts',(-9.87598480136881,-4.96131482748137,
-0.0925520037673158));
#70940=CARTESIAN_POINT('Ctrl Pts',(-9.87672696353113,-4.96188668514534,
-0.0618971741366425));
#70941=CARTESIAN_POINT('Ctrl Pts',(-9.87746912569345,-4.96214622116242,
-0.0312365182290158));
#70942=CARTESIAN_POINT('Ctrl Pts',(-9.87821128785577,-4.96209602020563,
-0.000574989514468549));
#70943=CARTESIAN_POINT('Ctrl Pts',(-9.98358871214408,-4.96212480437208,
0.0004625561064964));
#70944=CARTESIAN_POINT('Ctrl Pts',(-9.94442973905749,-4.9599743856448,-1.61731769660458));
#70945=CARTESIAN_POINT('Ctrl Pts',(-9.9052707659709,-4.09409792840036,-3.23707195902456));
#70946=CARTESIAN_POINT('Ctrl Pts',(-9.86611179288432,-2.7468265476734,-4.13257247735339));
#70947=CARTESIAN_POINT('Ctrl Pts',(-9.82635646874526,-1.3790376037284,-5.04171055138142));
#70948=CARTESIAN_POINT('Ctrl Pts',(-9.78660114460621,0.484920212884461,
-5.20436762571052));
#70949=CARTESIAN_POINT('Ctrl Pts',(-9.74684582046715,1.98950651863428,-4.54588552164414));
#70950=CARTESIAN_POINT('Ctrl Pts',(-9.7070904963281,3.49409282438405,-3.88740341757779));
#70951=CARTESIAN_POINT('Ctrl Pts',(-9.66733517218905,4.63930761927079,-2.40778213511593));
#70952=CARTESIAN_POINT('Ctrl Pts',(-9.62757984804999,4.89950729907218,-0.786154940148899));
#70953=CARTESIAN_POINT('Ctrl Pts',(-9.58782452391094,5.15970697887357,0.835472254818157));
#70954=CARTESIAN_POINT('Ctrl Pts',(-9.54806919977187,4.53489154358963,2.59910536229043));
#70955=CARTESIAN_POINT('Ctrl Pts',(-9.50831387563282,3.3118458294299,3.69525216536976));
#70956=CARTESIAN_POINT('Ctrl Pts',(-9.46855855149377,2.08880011527016,4.79139896844909));
#70957=CARTESIAN_POINT('Ctrl Pts',(-9.42880322735472,0.267524122234651,
5.22005946713543));
#70958=CARTESIAN_POINT('Ctrl Pts',(-9.38904790321567,-1.31603235096888,
4.78448223058519));
#70959=CARTESIAN_POINT('Ctrl Pts',(-9.34929257907661,-2.89958882417239,
4.34890499403496));
#70960=CARTESIAN_POINT('Ctrl Pts',(-9.30953725493755,-4.2454257775439,3.04909002224817));
#70961=CARTESIAN_POINT('Ctrl Pts',(-9.26978193079849,-4.73581578560452,
1.4816410524824));
#70962=CARTESIAN_POINT('Ctrl Pts',(-9.25771752458035,-4.88463268977224,
1.00597291225268));
#70963=CARTESIAN_POINT('Ctrl Pts',(-9.24565311836222,-4.95466988245972,
0.505657855859816));
#70964=CARTESIAN_POINT('Ctrl Pts',(-9.23358871214408,-4.95061007082821,
0.00423510493672523));
#70965=CARTESIAN_POINT('Origin',(10.45,0.,0.));
#70966=CARTESIAN_POINT('',(-8.37821128785577,-4.94626828646249,-0.0015636080438286));
#70967=CARTESIAN_POINT('',(-8.48358871214408,-4.94693680463334,-0.00239458277972477));
#70968=CARTESIAN_POINT('',(10.45,-4.954,-6.06690024297599E-16));
#70969=CARTESIAN_POINT('Ctrl Pts',(-8.37821128785577,-4.94626828646249,
-0.0015636080438286));
#70970=CARTESIAN_POINT('Ctrl Pts',(-8.4004052360248,-4.94365983576389,0.922899349173829));
#70971=CARTESIAN_POINT('Ctrl Pts',(-8.42259918419382,-4.69535029940576,
1.84866339909468));
#70972=CARTESIAN_POINT('Ctrl Pts',(-8.44479313236284,-4.21003313165683,
2.62656271981837));
#70973=CARTESIAN_POINT('Ctrl Pts',(-8.4845484565019,-3.34069969142485,4.01998940566081));
#70974=CARTESIAN_POINT('Ctrl Pts',(-8.52430378064095,-1.71089326297385,
4.93897089408532));
#70975=CARTESIAN_POINT('Ctrl Pts',(-8.56405910478,-0.0686807845416902,4.96170269571067));
#70976=CARTESIAN_POINT('Ctrl Pts',(-8.60381442891905,1.57353169389047,4.98443449733603));
#70977=CARTESIAN_POINT('Ctrl Pts',(-8.64356975305811,3.22815022230378,4.11091661216223));
#70978=CARTESIAN_POINT('Ctrl Pts',(-8.68332507719717,4.13571932494693,2.74208613213524));
#70979=CARTESIAN_POINT('Ctrl Pts',(-8.72308040133623,5.04328842759009,1.37325565210822));
#70980=CARTESIAN_POINT('Ctrl Pts',(-8.76283572547528,5.20380810446308,-0.490887422771993));
#70981=CARTESIAN_POINT('Ctrl Pts',(-8.80259104961434,4.5436012236629,-1.99471767704526));
#70982=CARTESIAN_POINT('Ctrl Pts',(-8.84234637375339,3.88339434286273,-3.49854793131853));
#70983=CARTESIAN_POINT('Ctrl Pts',(-8.88210169789244,2.40246090438938,-4.64206536498485));
#70984=CARTESIAN_POINT('Ctrl Pts',(-8.9218570220315,0.780536442300002,-4.90040544782057));
#70985=CARTESIAN_POINT('Ctrl Pts',(-8.96161234617055,-0.841388019789334,
-5.15874553065628));
#70986=CARTESIAN_POINT('Ctrl Pts',(-9.0013676703096,-2.6043035054947,-4.53190826266146));
#70987=CARTESIAN_POINT('Ctrl Pts',(-9.04112299444866,-3.69904718005105,
-3.30760648362894));
#70988=CARTESIAN_POINT('Ctrl Pts',(-9.07015242558436,-4.49843158453039,
-2.41361844672019));
#70989=CARTESIAN_POINT('Ctrl Pts',(-9.09918185672007,-4.94154980422565,
-1.20106503734346));
#70990=CARTESIAN_POINT('Ctrl Pts',(-9.12821128785577,-4.95217176878245,
0.00449694065580375));
#70991=CARTESIAN_POINT('Ctrl Pts',(-9.23358871214408,-4.95061007082821,
0.00423510493672523));
#70992=CARTESIAN_POINT('Ctrl Pts',(-9.20589779422316,-4.9412917580468,-1.14665918595834));
#70993=CARTESIAN_POINT('Ctrl Pts',(-9.17820687630225,-4.54161511541906,
-2.30338904052803));
#70994=CARTESIAN_POINT('Ctrl Pts',(-9.15051595838133,-3.80820292464108,
-3.18132077105363));
#70995=CARTESIAN_POINT('Ctrl Pts',(-9.11076063424228,-2.75525699286724,
-4.44175065707925));
#70996=CARTESIAN_POINT('Ctrl Pts',(-9.07100531010322,-1.01442206656976,
-5.12752746138567));
#70997=CARTESIAN_POINT('Ctrl Pts',(-9.03124998596417,0.615273803705024,
-4.92388561098412));
#70998=CARTESIAN_POINT('Ctrl Pts',(-8.99149466182511,2.24496967397974,-4.72024376058259));
#70999=CARTESIAN_POINT('Ctrl Pts',(-8.95173933768606,3.76352648823178,-3.62718325547323));
#71000=CARTESIAN_POINT('Ctrl Pts',(-8.911984013547,4.47393991100926,-2.14640933567216));
#71001=CARTESIAN_POINT('Ctrl Pts',(-8.87222868940795,5.18435333378674,-0.665635415871093));
#71002=CARTESIAN_POINT('Ctrl Pts',(-8.83247336526889,5.08662336508962,1.20285191862169));
#71003=CARTESIAN_POINT('Ctrl Pts',(-8.79271804112984,4.22560720831403,2.60143327506715));
#71004=CARTESIAN_POINT('Ctrl Pts',(-8.75296271699079,3.36459105153842,4.00001463151265));
#71005=CARTESIAN_POINT('Ctrl Pts',(-8.71320739285173,1.74028870668433,4.92869000991082));
#71006=CARTESIAN_POINT('Ctrl Pts',(-8.67345206871267,0.0982407856159575,
4.96120550991629));
#71007=CARTESIAN_POINT('Ctrl Pts',(-8.63369674457362,-1.54380713545237,
4.99372100992175));
#71008=CARTESIAN_POINT('Ctrl Pts',(-8.59394142043456,-3.20360063273498,
4.13007663153452));
#71009=CARTESIAN_POINT('Ctrl Pts',(-8.5541860962955,-4.11930896489686,2.76667761318562));
#71010=CARTESIAN_POINT('Ctrl Pts',(-8.53065363491169,-4.66134632547929,
1.95963766457907));
#71011=CARTESIAN_POINT('Ctrl Pts',(-8.50712117352789,-4.942668242245,0.977491748450743));
#71012=CARTESIAN_POINT('Ctrl Pts',(-8.48358871214408,-4.94693680463334,
-0.00239458277972477));
#71013=CARTESIAN_POINT('Origin',(10.45,0.,0.));
#71014=CARTESIAN_POINT('',(-7.62821128785578,-4.95792182903176,-0.00387990541073024));
#71015=CARTESIAN_POINT('',(-7.73358871214408,-4.95939673491496,-0.00326695968845118));
#71016=CARTESIAN_POINT('',(10.45,-4.954,-6.06690024297599E-16));
#71017=CARTESIAN_POINT('Ctrl Pts',(-7.62821128785578,-4.95792182903176,
-0.00387990541073024));
#71018=CARTESIAN_POINT('Ctrl Pts',(-7.66187329119047,-4.94592861234691,
1.38990971447958));
#71019=CARTESIAN_POINT('Ctrl Pts',(-7.69553529452516,-4.33087130523565,
2.79296473185555));
#71020=CARTESIAN_POINT('Ctrl Pts',(-7.72919729785985,-3.28977114370411,
3.71491810311339));
#71021=CARTESIAN_POINT('Ctrl Pts',(-7.76895262199891,-2.0602164445561,4.80375867956457));
#71022=CARTESIAN_POINT('Ctrl Pts',(-7.80870794613796,-0.236418894111356,
5.22156062460434));
#71023=CARTESIAN_POINT('Ctrl Pts',(-7.84846327027702,1.34451433606028,4.77655648882291));
#71024=CARTESIAN_POINT('Ctrl Pts',(-7.88821859441607,2.92544756623186,4.33155235304148));
#71025=CARTESIAN_POINT('Ctrl Pts',(-7.92797391855513,4.26351647613036,3.02374213643891));
#71026=CARTESIAN_POINT('Ctrl Pts',(-7.96772924269418,4.74455910449121,1.45339932392216));
#71027=CARTESIAN_POINT('Ctrl Pts',(-8.00748456683323,5.22560173285208,-0.11694348859464));
#71028=CARTESIAN_POINT('Ctrl Pts',(-8.04723989097229,4.84961807967525,-1.94981889702563));
#71029=CARTESIAN_POINT('Ctrl Pts',(-8.08699521511134,3.78918136307401,-3.20395307214704));
#71030=CARTESIAN_POINT('Ctrl Pts',(-8.1267505392504,2.72874464647277,-4.45808724726844));
#71031=CARTESIAN_POINT('Ctrl Pts',(-8.16650586338946,0.983854866447135,
-5.13348018908026));
#71032=CARTESIAN_POINT('Ctrl Pts',(-8.20626118752851,-0.644598783955043,
-4.92013242692831));
#71033=CARTESIAN_POINT('Ctrl Pts',(-8.24601651166757,-2.27305243435722,
-4.70678466477637));
#71034=CARTESIAN_POINT('Ctrl Pts',(-8.28577183580661,-3.78506995513594,
-3.60469619866064));
#71035=CARTESIAN_POINT('Ctrl Pts',(-8.32552715994567,-4.48664848951884,
-2.11971602397259));
#71036=CARTESIAN_POINT('Ctrl Pts',(-8.3430885359157,-4.79656130450954,-1.46374614520803));
#71037=CARTESIAN_POINT('Ctrl Pts',(-8.36064991188574,-4.94833227179167,
-0.733062187675864));
#71038=CARTESIAN_POINT('Ctrl Pts',(-8.37821128785577,-4.94626828646249,
-0.0015636080438286));
#71039=CARTESIAN_POINT('Ctrl Pts',(-8.48358871214408,-4.94693680463334,
-0.00239458277972477));
#71040=CARTESIAN_POINT('Ctrl Pts',(-8.46736584938883,-4.94987947606319,
-0.677910892273384));
#71041=CARTESIAN_POINT('Ctrl Pts',(-8.45114298663359,-4.82115310072354,
-1.35235333861075));
#71042=CARTESIAN_POINT('Ctrl Pts',(-8.43492012387834,-4.55540492895606,
-1.96761207986355));
#71043=CARTESIAN_POINT('Ctrl Pts',(-8.39516479973929,-3.90416939381222,
-3.47534909625313));
#71044=CARTESIAN_POINT('Ctrl Pts',(-8.35540947560023,-2.43007515648339,
-4.62766947072172));
#71045=CARTESIAN_POINT('Ctrl Pts',(-8.31565415146118,-0.809718617341338,
-4.8956681999818));
#71046=CARTESIAN_POINT('Ctrl Pts',(-8.27589882732213,0.810637921800733,
-5.16366692924188));
#71047=CARTESIAN_POINT('Ctrl Pts',(-8.23614350318307,2.57725676275602,-4.54734401329347));
#71048=CARTESIAN_POINT('Ctrl Pts',(-8.19638817904401,3.6792752629942,-3.32958629602854));
#71049=CARTESIAN_POINT('Ctrl Pts',(-8.15663285490496,4.78129376323237,-2.11182857876362));
#71050=CARTESIAN_POINT('Ctrl Pts',(-8.1168775307659,5.21871192275341,-0.292636060182249));
#71051=CARTESIAN_POINT('Ctrl Pts',(-8.07712220662685,4.79075862076016,1.29299775761381));
#71052=CARTESIAN_POINT('Ctrl Pts',(-8.03736688248779,4.3628053187669,2.87863157540991));
#71053=CARTESIAN_POINT('Ctrl Pts',(-7.99761155834874,3.06948055525926,4.23070669242067));
#71054=CARTESIAN_POINT('Ctrl Pts',(-7.95785623420969,1.50440911849139,4.72863242045542));
#71055=CARTESIAN_POINT('Ctrl Pts',(-7.91810091007063,-0.060662318276431,
5.22655814849016));
#71056=CARTESIAN_POINT('Ctrl Pts',(-7.87834558593158,-1.89748042830445,
4.87033448754899));
#71057=CARTESIAN_POINT('Ctrl Pts',(-7.83859026179252,-3.16296171671753,
3.82346499162231));
#71058=CARTESIAN_POINT('Ctrl Pts',(-7.80358974524304,-4.27708918863134,
2.90180295236524));
#71059=CARTESIAN_POINT('Ctrl Pts',(-7.76858922869356,-4.94837290551537,
1.44482061973698));
#71060=CARTESIAN_POINT('Ctrl Pts',(-7.73358871214408,-4.95939673491496,
-0.00326695968845118));
#71061=CARTESIAN_POINT('Origin',(10.45,0.,0.));
#71062=CARTESIAN_POINT('',(-6.87821128785577,-4.9587369089069,0.00357303255080571));
#71063=CARTESIAN_POINT('',(-6.98358871214407,-4.95718456603373,0.00410112652448823));
#71064=CARTESIAN_POINT('',(10.45,-4.954,-6.06690024297599E-16));
#71065=CARTESIAN_POINT('Ctrl Pts',(-6.87821128785577,-4.9587369089069,0.00357303255080571));
#71066=CARTESIAN_POINT('Ctrl Pts',(-6.88358602221708,-4.9605454351019,0.226020979139462));
#71067=CARTESIAN_POINT('Ctrl Pts',(-6.88896075657839,-4.94687668270747,
0.448245317794466));
#71068=CARTESIAN_POINT('Ctrl Pts',(-6.8943354909397,-4.91697415180519,0.668263332278103));
#71069=CARTESIAN_POINT('Ctrl Pts',(-6.93409081507876,-4.69579395410926,
2.29567166434186));
#71070=CARTESIAN_POINT('Ctrl Pts',(-6.97384613921781,-3.58644354271542,
3.80236925676953));
#71071=CARTESIAN_POINT('Ctrl Pts',(-7.01360146335687,-2.09810508257134,
4.49679505351046));
#71072=CARTESIAN_POINT('Ctrl Pts',(-7.05335678749592,-0.609766622427246,
5.1912208502514));
#71073=CARTESIAN_POINT('Ctrl Pts',(-7.09311211163498,1.25755988646708,5.0733748513056));
#71074=CARTESIAN_POINT('Ctrl Pts',(-7.13286743577403,2.64678786019961,4.19734734253526));
#71075=CARTESIAN_POINT('Ctrl Pts',(-7.17262275991308,4.03601583393218,3.3213198337649));
#71076=CARTESIAN_POINT('Ctrl Pts',(-7.21237808405213,4.94714527250291,1.68711081516997));
#71077=CARTESIAN_POINT('Ctrl Pts',(-7.25213340819119,4.96197570894114,0.0448079754724352));
#71078=CARTESIAN_POINT('Ctrl Pts',(-7.29188873233025,4.97680614537936,-1.5974948642251));
#71079=CARTESIAN_POINT('Ctrl Pts',(-7.33164405646931,4.09533757968508,-3.24789152502519));
#71080=CARTESIAN_POINT('Ctrl Pts',(-7.37139938060836,2.72215639683076,-4.148864331595));
#71081=CARTESIAN_POINT('Ctrl Pts',(-7.41115470474741,1.34897521397647,-5.04983713816479));
#71082=CARTESIAN_POINT('Ctrl Pts',(-7.45091002888646,-0.515918586037916,
-5.20138609050432));
#71083=CARTESIAN_POINT('Ctrl Pts',(-7.49066535302552,-2.01655501146214,
-4.53395154104395));
#71084=CARTESIAN_POINT('Ctrl Pts',(-7.53042067716457,-3.51719143688638,
-3.86651699158356));
#71085=CARTESIAN_POINT('Ctrl Pts',(-7.57017600130363,-4.65357048772051,
-2.38009894032327));
#71086=CARTESIAN_POINT('Ctrl Pts',(-7.60993132544269,-4.90410408921195,
-0.756950310761838));
#71087=CARTESIAN_POINT('Ctrl Pts',(-7.61602464624705,-4.94250351467808,
-0.508169410913484));
#71088=CARTESIAN_POINT('Ctrl Pts',(-7.62211796705141,-4.96009277875244,
-0.25617645482694));
#71089=CARTESIAN_POINT('Ctrl Pts',(-7.62821128785578,-4.95792182903176,
-0.00387990541073024));
#71090=CARTESIAN_POINT('Ctrl Pts',(-7.73358871214408,-4.95939673491496,
-0.00326695968845118));
#71091=CARTESIAN_POINT('Ctrl Pts',(-7.72883390455451,-4.96089431817551,
-0.199989136725148));
#71092=CARTESIAN_POINT('Ctrl Pts',(-7.72407909696493,-4.95020672280133,
-0.396547159981269));
#71093=CARTESIAN_POINT('Ctrl Pts',(-7.71932428937536,-4.9267888600081,-0.591576615902107));
#71094=CARTESIAN_POINT('Ctrl Pts',(-7.6795689652363,-4.73099024808745,-2.22223339658757));
#71095=CARTESIAN_POINT('Ctrl Pts',(-7.63981364109725,-3.64524855744802,
-3.74603162704625));
#71096=CARTESIAN_POINT('Ctrl Pts',(-7.60005831695819,-2.16790975608666,
-4.46356120749413));
#71097=CARTESIAN_POINT('Ctrl Pts',(-7.56030299281914,-0.690570954725322,
-5.18109078794199));
#71098=CARTESIAN_POINT('Ctrl Pts',(-7.52054766868008,1.17836495735796,-5.09235171837907));
#71099=CARTESIAN_POINT('Ctrl Pts',(-7.48079234454102,2.58107269422186,-4.23807445790236));
#71100=CARTESIAN_POINT('Ctrl Pts',(-7.44103702040197,3.98378043108578,-3.38379719742564));
#71101=CARTESIAN_POINT('Ctrl Pts',(-7.40128169626292,4.92025999273031,-1.76398174603515));
#71102=CARTESIAN_POINT('Ctrl Pts',(-7.36152637212387,4.96067542675493,-0.122109270622357));
#71103=CARTESIAN_POINT('Ctrl Pts',(-7.32177104798481,5.00109086077955,1.51976320479041));
#71104=CARTESIAN_POINT('Ctrl Pts',(-7.28201572384575,4.14544216718425,3.18369270422544));
#71105=CARTESIAN_POINT('Ctrl Pts',(-7.2422603997067,2.78646463480541,4.10595009742701));
#71106=CARTESIAN_POINT('Ctrl Pts',(-7.20250507556765,1.42748710242655,5.0282074906286));
#71107=CARTESIAN_POINT('Ctrl Pts',(-7.16274975142859,-0.434819268735898,
5.20879277759671));
#71108=CARTESIAN_POINT('Ctrl Pts',(-7.12299442728954,-1.94567209421158,
4.56481888637309));
#71109=CARTESIAN_POINT('Ctrl Pts',(-7.08323910315048,-3.45652491968723,
3.92084499514948));
#71110=CARTESIAN_POINT('Ctrl Pts',(-7.04348377901142,-4.61592419947615,
2.45231192573416));
#71111=CARTESIAN_POINT('Ctrl Pts',(-7.00372845487237,-4.89171577447908,
0.83326355092171));
#71112=CARTESIAN_POINT('Ctrl Pts',(-6.99701520729627,-4.93828707436135,
0.559864382051187));
#71113=CARTESIAN_POINT('Ctrl Pts',(-6.99030195972017,-4.95966222198897,
0.282173255866473));
#71114=CARTESIAN_POINT('Ctrl Pts',(-6.98358871214407,-4.95718456603373,
0.00410112652448823));
#71115=CARTESIAN_POINT('Origin',(10.45,0.,0.));
#71116=CARTESIAN_POINT('',(-6.12821128785577,-4.94659179946477,0.00201959180113259));
#71117=CARTESIAN_POINT('',(-6.23358871214408,-4.94605717997479,0.00115570248479588));
#71118=CARTESIAN_POINT('',(10.45,-4.954,-6.06690024297599E-16));
#71119=CARTESIAN_POINT('Ctrl Pts',(-6.12821128785577,-4.94659179946477,
0.00201959180113259));
#71120=CARTESIAN_POINT('Ctrl Pts',(-6.14505407738275,-4.94915812932308,
0.703471731949359));
#71121=CARTESIAN_POINT('Ctrl Pts',(-6.16189686690973,-4.81001858480067,
1.40395201041217));
#71122=CARTESIAN_POINT('Ctrl Pts',(-6.17873965643671,-4.52419690513961,
2.03834566605201));
#71123=CARTESIAN_POINT('Ctrl Pts',(-6.21849498057577,-3.84955013699639,
3.53575352544014));
#71124=CARTESIAN_POINT('Ctrl Pts',(-6.25825030471482,-2.3576818810049,4.6649678881952));
#71125=CARTESIAN_POINT('Ctrl Pts',(-6.29800562885388,-0.733346657108161,
4.90768920891453));
#71126=CARTESIAN_POINT('Ctrl Pts',(-6.33776095299293,0.890988566788603,
5.15041052963386));
#71127=CARTESIAN_POINT('Ctrl Pts',(-6.37751627713199,2.6477907585907,4.50663880831747));
#71128=CARTESIAN_POINT('Ctrl Pts',(-6.41727160127105,3.73070303212477,3.2718596511591));
#71129=CARTESIAN_POINT('Ctrl Pts',(-6.4570269254101,4.81361530565883,2.03708049400074));
#71130=CARTESIAN_POINT('Ctrl Pts',(-6.49678224954915,5.22263766092491,0.211293901000479));
#71131=CARTESIAN_POINT('Ctrl Pts',(-6.5365375736882,4.7700324036586,-1.36748000308405));
#71132=CARTESIAN_POINT('Ctrl Pts',(-6.57629289782726,4.3174271463923,-2.94625390716858));
#71133=CARTESIAN_POINT('Ctrl Pts',(-6.61604822196632,3.00319427659351,-4.27801512233737));
#71134=CARTESIAN_POINT('Ctrl Pts',(-6.65580354610537,1.43055522097884,-4.75149686420164));
#71135=CARTESIAN_POINT('Ctrl Pts',(-6.69555887024443,-0.142083834635853,
-5.22497860606591));
#71136=CARTESIAN_POINT('Ctrl Pts',(-6.73531419438348,-1.97312907606641,
-4.84018087462572));
#71137=CARTESIAN_POINT('Ctrl Pts',(-6.77506951852254,-3.22214670478274,
-3.77372247305569));
#71138=CARTESIAN_POINT('Ctrl Pts',(-6.80945010830028,-4.30230297688017,
-2.85144427225017));
#71139=CARTESIAN_POINT('Ctrl Pts',(-6.84383069807803,-4.94716830048226,
-1.41936084370118));
#71140=CARTESIAN_POINT('Ctrl Pts',(-6.87821128785577,-4.9587369089069,0.00357303255080571));
#71141=CARTESIAN_POINT('Ctrl Pts',(-6.98358871214407,-4.95718456603373,
0.00410112652448823));
#71142=CARTESIAN_POINT('Ctrl Pts',(-6.95054663558112,-4.94498973829323,
-1.36454802332293));
#71143=CARTESIAN_POINT('Ctrl Pts',(-6.91750455901817,-4.35495335507998,
-2.74242709267509));
#71144=CARTESIAN_POINT('Ctrl Pts',(-6.88446248245521,-3.34724968835376,
-3.66321319163897));
#71145=CARTESIAN_POINT('Ctrl Pts',(-6.84470715831616,-2.13480815700861,
-4.77107787917753));
#71146=CARTESIAN_POINT('Ctrl Pts',(-6.80495183417709,-0.317741224101409,
-5.21724357404503));
#71147=CARTESIAN_POINT('Ctrl Pts',(-6.76519651003804,1.26993323355469,-4.79692411300152));
#71148=CARTESIAN_POINT('Ctrl Pts',(-6.72544118589898,2.8576076912108,-4.37660465195801));
#71149=CARTESIAN_POINT('Ctrl Pts',(-6.68568586175993,4.21588967361574,-3.08980003500352));
#71150=CARTESIAN_POINT('Ctrl Pts',(-6.64593053762088,4.72133959548887,-1.5271423599819));
#71151=CARTESIAN_POINT('Ctrl Pts',(-6.60617521348182,5.22678951736199,0.0355153150397139));
#71152=CARTESIAN_POINT('Ctrl Pts',(-6.56641988934277,4.87940737870325,1.87402604812845));
#71153=CARTESIAN_POINT('Ctrl Pts',(-6.52666456520372,3.83863855187625,3.14452944518438));
#71154=CARTESIAN_POINT('Ctrl Pts',(-6.48690924106466,2.79786972504925,4.4150328422403));
#71155=CARTESIAN_POINT('Ctrl Pts',(-6.4471539169256,1.06371421005396,5.11752890326346));
#71156=CARTESIAN_POINT('Ctrl Pts',(-6.40739859278654,-0.567865734104478,
4.92957806222927));
#71157=CARTESIAN_POINT('Ctrl Pts',(-6.36764326864749,-2.19944567826289,
4.74162722119508));
#71158=CARTESIAN_POINT('Ctrl Pts',(-6.32788794450843,-3.72845005158446,
3.66322947810363));
#71159=CARTESIAN_POINT('Ctrl Pts',(-6.28813262036938,-4.45307918011037,
2.18935999306868));
#71160=CARTESIAN_POINT('Ctrl Pts',(-6.26995131762761,-4.78447382589796,
1.51531524838128));
#71161=CARTESIAN_POINT('Ctrl Pts',(-6.25177001488584,-4.94763279638995,
0.758557297392875));
#71162=CARTESIAN_POINT('Ctrl Pts',(-6.23358871214408,-4.94605717997479,
0.00115570248479588));
#71163=CARTESIAN_POINT('Origin',(10.45,0.,0.));
#71164=CARTESIAN_POINT('',(-5.37821128785577,-4.95131745647145,-0.00437947150781604));
#71165=CARTESIAN_POINT('',(-5.48358871214407,-4.95293198292091,-0.00455366204130441));
#71166=CARTESIAN_POINT('',(10.45,-4.954,-6.06690024297599E-16));
#71167=CARTESIAN_POINT('Ctrl Pts',(-5.37821128785577,-4.95131745647145,
-0.00437947150781604));
#71168=CARTESIAN_POINT('Ctrl Pts',(-5.40652213254842,-4.9413622877759,1.17185497477651));
#71169=CARTESIAN_POINT('Ctrl Pts',(-5.43483297724108,-4.52190080861264,
2.35447063781816));
#71170=CARTESIAN_POINT('Ctrl Pts',(-5.46314382193373,-3.75817622776498,
3.24026575018933));
#71171=CARTESIAN_POINT('Ctrl Pts',(-5.50289914607278,-2.68572082792868,
4.48413791986167));
#71172=CARTESIAN_POINT('Ctrl Pts',(-5.54265447021184,-0.934412930545154,
5.1427095703667));
#71173=CARTESIAN_POINT('Ctrl Pts',(-5.58240979435089,0.691912411438593,
4.91370205707316));
#71174=CARTESIAN_POINT('Ctrl Pts',(-5.62216511848994,2.31823775342232,4.68469454377963));
#71175=CARTESIAN_POINT('Ctrl Pts',(-5.661920442629,3.81958054000623,3.56810786668746));
#71176=CARTESIAN_POINT('Ctrl Pts',(-5.70167576676805,4.50683752432629,2.07644557359742));
#71177=CARTESIAN_POINT('Ctrl Pts',(-5.74143109090711,5.19409450864639,0.584783280507319));
#71178=CARTESIAN_POINT('Ctrl Pts',(-5.78118641504617,5.06726569070262,-1.28195462858072));
#71179=CARTESIAN_POINT('Ctrl Pts',(-5.82094173918522,4.18456439194428,-2.6669517319329));
#71180=CARTESIAN_POINT('Ctrl Pts',(-5.86069706332428,3.30186309318596,-4.05194883528503));
#71181=CARTESIAN_POINT('Ctrl Pts',(-5.90045238746333,1.66328931361312,-4.95520513290133));
#71182=CARTESIAN_POINT('Ctrl Pts',(-5.94020771160238,0.020934129174502,
-4.96213386085296));
#71183=CARTESIAN_POINT('Ctrl Pts',(-5.97996303574144,-1.62142105526411,
-4.9690625888046));
#71184=CARTESIAN_POINT('Ctrl Pts',(-6.01971835988049,-3.2675576445685,-4.07966374709158));
#71185=CARTESIAN_POINT('Ctrl Pts',(-6.05947368401955,-4.16191329907318,
-2.70216364822446));
#71186=CARTESIAN_POINT('Ctrl Pts',(-6.08238621863162,-4.67736513686141,
-1.90825693567869));
#71187=CARTESIAN_POINT('Ctrl Pts',(-6.1052987532437,-4.94310062470359,-0.95221939658693));
#71188=CARTESIAN_POINT('Ctrl Pts',(-6.12821128785577,-4.94659179946477,
0.00201959180113259));
#71189=CARTESIAN_POINT('Ctrl Pts',(-6.23358871214408,-4.94605717997479,
0.00115570248479588));
#71190=CARTESIAN_POINT('Ctrl Pts',(-6.21201469074679,-4.94418754594816,
-0.897580677793857));
#71191=CARTESIAN_POINT('Ctrl Pts',(-6.19044066934951,-4.71036650847862,
-1.79722332865776));
#71192=CARTESIAN_POINT('Ctrl Pts',(-6.16886664795222,-4.25044360325777,
-2.56065236592303));
#71193=CARTESIAN_POINT('Ctrl Pts',(-6.12911132381317,-3.40292501414906,
-3.96745401290124));
#71194=CARTESIAN_POINT('Ctrl Pts',(-6.08935599967411,-1.78763395220142,
-4.91171607987924));
#71195=CARTESIAN_POINT('Ctrl Pts',(-6.04960067553505,-0.14597492900625,
-4.96003051237427));
#71196=CARTESIAN_POINT('Ctrl Pts',(-6.00984535139599,1.49568409418894,-5.0083449448693));
#71197=CARTESIAN_POINT('Ctrl Pts',(-5.97009002725694,3.16371107863165,-4.16071174288138));
#71198=CARTESIAN_POINT('Ctrl Pts',(-5.93033470311789,4.09249618417905,-2.80618715449666));
#71199=CARTESIAN_POINT('Ctrl Pts',(-5.89057937897884,5.02128128972644,-1.45166256611195));
#71200=CARTESIAN_POINT('Ctrl Pts',(-5.85082405483978,5.2108245163785,0.409753408669569));
#71201=CARTESIAN_POINT('Ctrl Pts',(-5.81106873070073,4.57412717597807,1.92368706955186));
#71202=CARTESIAN_POINT('Ctrl Pts',(-5.77131340656167,3.93742983557762,3.43762073043419));
#71203=CARTESIAN_POINT('Ctrl Pts',(-5.73155808242261,2.47449192812468,4.60407207741728));
#71204=CARTESIAN_POINT('Ctrl Pts',(-5.69180275828356,0.856789195864615,
4.88765011405602));
#71205=CARTESIAN_POINT('Ctrl Pts',(-5.6520474341445,-0.760913536395409,
5.17122815069474));
#71206=CARTESIAN_POINT('Ctrl Pts',(-5.61229211000545,-2.53338109346257,
4.57193287698912));
#71207=CARTESIAN_POINT('Ctrl Pts',(-5.5725367858664,-3.64706632311371,3.36483559752805));
#71208=CARTESIAN_POINT('Ctrl Pts',(-5.54288742795896,-4.47764820579843,
2.46458739070536));
#71209=CARTESIAN_POINT('Ctrl Pts',(-5.51323807005152,-4.94180776187748,
1.22627270001379));
#71210=CARTESIAN_POINT('Ctrl Pts',(-5.48358871214407,-4.95293198292091,
-0.00455366204130441));
#71211=CARTESIAN_POINT('Origin',(10.45,0.,0.));
#71212=CARTESIAN_POINT('',(-4.62821128785577,-4.96217793349678,1.83253063722107E-5));
#71213=CARTESIAN_POINT('',(-4.73358871214408,-4.96190938845054,0.00104730840813116));
#71214=CARTESIAN_POINT('',(10.45,-4.954,-6.06690024297599E-16));
#71215=CARTESIAN_POINT('Ctrl Pts',(-4.62821128785577,-4.96217793349678,
1.83253063722107E-5));
#71216=CARTESIAN_POINT('Ctrl Pts',(-4.66799018771409,-4.96226779169355,
1.64336216035063));
#71217=CARTESIAN_POINT('Ctrl Pts',(-4.70776908757242,-4.06471490519605,
3.28662169090852));
#71218=CARTESIAN_POINT('Ctrl Pts',(-4.74754798743074,-2.68210834911436,
4.1748659253201));
#71219=CARTESIAN_POINT('Ctrl Pts',(-4.7873033115698,-1.3003212210245,5.06258372494367));
#71220=CARTESIAN_POINT('Ctrl Pts',(-4.82705863570885,0.565944505497547,
5.1961809116512));
#71221=CARTESIAN_POINT('Ctrl Pts',(-4.8668139598479,2.06008913639825,4.51433754175314));
#71222=CARTESIAN_POINT('Ctrl Pts',(-4.90656928398696,3.55423376729897,3.83249417185506));
#71223=CARTESIAN_POINT('Ctrl Pts',(-4.94632460812601,4.67625730257835,2.33521024535137));
#71224=CARTESIAN_POINT('Ctrl Pts',(-4.98607993226507,4.91116072393883,0.70972602772372));
#71225=CARTESIAN_POINT('Ctrl Pts',(-5.02583525640412,5.14606414529932,-0.91575818990395));
#71226=CARTESIAN_POINT('Ctrl Pts',(-5.06559058054318,4.49384745274089,-2.66944269865558));
#71227=CARTESIAN_POINT('Ctrl Pts',(-5.10534590468223,3.25387242061459,-3.74640160169083));
#71228=CARTESIAN_POINT('Ctrl Pts',(-5.14510122882129,2.01389738848831,-4.82336050472606));
#71229=CARTESIAN_POINT('Ctrl Pts',(-5.18485655296034,0.186164016794188,
-5.22359380204494));
#71230=CARTESIAN_POINT('Ctrl Pts',(-5.2246118770994,-1.39041401526609,-4.76339790033747));
#71231=CARTESIAN_POINT('Ctrl Pts',(-5.26436720123845,-2.96699204732638,
-4.30320199863));
#71232=CARTESIAN_POINT('Ctrl Pts',(-5.30412252537751,-4.29241473975282,
-2.98257689789619));
#71233=CARTESIAN_POINT('Ctrl Pts',(-5.34387784951656,-4.75832463482155,
-1.40767800310946));
#71234=CARTESIAN_POINT('Ctrl Pts',(-5.35532232896297,-4.89244745568799,
-0.954307330831556));
#71235=CARTESIAN_POINT('Ctrl Pts',(-5.36676680840937,-4.95534177029036,
-0.479864787851824));
#71236=CARTESIAN_POINT('Ctrl Pts',(-5.37821128785577,-4.95131745647145,
-0.00437947150781604));
#71237=CARTESIAN_POINT('Ctrl Pts',(-5.48358871214407,-4.95293198292091,
-0.00455366204130441));
#71238=CARTESIAN_POINT('Ctrl Pts',(-5.47348274591246,-4.95672366713103,
-0.424080104763632));
#71239=CARTESIAN_POINT('Ctrl Pts',(-5.46337677968084,-4.9078824662274,-0.842736566029038));
#71240=CARTESIAN_POINT('Ctrl Pts',(-5.45327081344923,-4.80297856458869,
-1.24683931269579));
#71241=CARTESIAN_POINT('Ctrl Pts',(-5.41351548931017,-4.39030267417733,
-2.83651765824206));
#71242=CARTESIAN_POINT('Ctrl Pts',(-5.37376016517112,-3.11004799111942,
-4.20097506411805));
#71243=CARTESIAN_POINT('Ctrl Pts',(-5.33400484103207,-1.54984025071783,
-4.71393747952145));
#71244=CARTESIAN_POINT('Ctrl Pts',(-5.29424951689301,0.0103674896837219,
-5.22689989492483));
#71245=CARTESIAN_POINT('Ctrl Pts',(-5.25449419275395,1.85052828742895,-4.88836731985566));
#71246=CARTESIAN_POINT('Ctrl Pts',(-5.2147388686149,3.12602438312975,-3.85372325416089));
#71247=CARTESIAN_POINT('Ctrl Pts',(-5.17498354447584,4.40152047883059,-2.81907918846609));
#71248=CARTESIAN_POINT('Ctrl Pts',(-5.1352282203368,5.11235187248696,-1.08832363214565));
#71249=CARTESIAN_POINT('Ctrl Pts',(-5.09547289619774,4.93225315308238,0.544141707178393));
#71250=CARTESIAN_POINT('Ctrl Pts',(-5.05571757205869,4.7521544336778,2.17660704650244));
#71251=CARTESIAN_POINT('Ctrl Pts',(-5.01596224791963,3.68112560121227,3.71078216883009));
#71252=CARTESIAN_POINT('Ctrl Pts',(-4.97620692378057,2.2107595500815,4.4424940714992));
#71253=CARTESIAN_POINT('Ctrl Pts',(-4.93645159964152,0.74039349895078,5.1742059741683));
#71254=CARTESIAN_POINT('Ctrl Pts',(-4.89669627550247,-1.12930977084514,
5.10345465717892));
#71255=CARTESIAN_POINT('Ctrl Pts',(-4.85694095136341,-2.54017276286649,
4.2627143580556));
#71256=CARTESIAN_POINT('Ctrl Pts',(-4.81718562722436,-3.95103575488788,
3.42197405893225));
#71257=CARTESIAN_POINT('Ctrl Pts',(-4.7774303030853,-4.90305846913465,1.81124477767492));
#71258=CARTESIAN_POINT('Ctrl Pts',(-4.73767497894624,-4.95927078170297,
0.169837208318289));
#71259=CARTESIAN_POINT('Ctrl Pts',(-4.73631289001219,-4.96119671667055,
0.113599631719194));
#71260=CARTESIAN_POINT('Ctrl Pts',(-4.73495080107814,-4.96207108588767,
0.0573260427708458));
#71261=CARTESIAN_POINT('Ctrl Pts',(-4.73358871214408,-4.96190938845054,
0.00104730840813116));
#71262=CARTESIAN_POINT('Origin',(10.45,0.,0.));
#71263=CARTESIAN_POINT('',(-3.87821128785577,-4.95126260644063,0.00436986867149824));
#71264=CARTESIAN_POINT('',(-3.98358871214407,-4.94978226424517,0.00400445798880121));
#71265=CARTESIAN_POINT('',(10.45,-4.954,-6.06690024297599E-16));
#71266=CARTESIAN_POINT('Ctrl Pts',(-3.87821128785577,-4.95126260644063,
0.00436986867149824));
#71267=CARTESIAN_POINT('Ctrl Pts',(-3.88970291874071,-4.95529130462732,
0.481827588074343));
#71268=CARTESIAN_POINT('Ctrl Pts',(-3.90119454962565,-4.89186792492517,
0.958237191039586));
#71269=CARTESIAN_POINT('Ctrl Pts',(-3.91268618051059,-4.75665313243704,
1.41331584172282));
#71270=CARTESIAN_POINT('Ctrl Pts',(-3.95244150464964,-4.28887723904272,
2.98766150665242));
#71271=CARTESIAN_POINT('Ctrl Pts',(-3.9921968287887,-2.96189047760415,4.30671499505008));
#71272=CARTESIAN_POINT('Ctrl Pts',(-4.03195215292775,-1.38476819988259,
4.76504225829968));
#71273=CARTESIAN_POINT('Ctrl Pts',(-4.07170747706681,0.192354077838921,
5.22336952154927));
#71274=CARTESIAN_POINT('Ctrl Pts',(-4.11146280120586,2.0196118718434,4.82097055965087));
#71275=CARTESIAN_POINT('Ctrl Pts',(-4.15121812534491,3.25830978894152,3.74254298707118));
#71276=CARTESIAN_POINT('Ctrl Pts',(-4.19097344948397,4.49700770603967,2.66411541449148));
#71277=CARTESIAN_POINT('Ctrl Pts',(-4.23072877362303,5.14714574623144,0.909659231230486));
#71278=CARTESIAN_POINT('Ctrl Pts',(-4.27048409776208,4.91031621847561,-0.715545474000941));
#71279=CARTESIAN_POINT('Ctrl Pts',(-4.31023942190114,4.67348669071978,-2.34075017923237));
#71280=CARTESIAN_POINT('Ctrl Pts',(-4.34999474604019,3.54968959501634,-3.83670340643423));
#71281=CARTESIAN_POINT('Ctrl Pts',(-4.38975007017924,2.05473799843147,-4.51677566950028));
#71282=CARTESIAN_POINT('Ctrl Pts',(-4.4295053943183,0.559786401846604,-5.19684793256633));
#71283=CARTESIAN_POINT('Ctrl Pts',(-4.46926071845735,-1.30631969561969,
-5.06103923149656));
#71284=CARTESIAN_POINT('Ctrl Pts',(-4.50901604259641,-2.68705386825844,
-4.17168457578772));
#71285=CARTESIAN_POINT('Ctrl Pts',(-4.54874779101619,-4.06696923732954,
-3.28285732555593));
#71286=CARTESIAN_POINT('Ctrl Pts',(-4.58847953943598,-4.96208818181233,
-1.64137759196963));
#71287=CARTESIAN_POINT('Ctrl Pts',(-4.62821128785577,-4.96217793349678,
1.83253063722107E-5));
#71288=CARTESIAN_POINT('Ctrl Pts',(-4.73358871214408,-4.96190938845054,
0.00104730840813116));
#71289=CARTESIAN_POINT('Ctrl Pts',(-4.69519547693908,-4.95735161870378,
-1.58528279927264));
#71290=CARTESIAN_POINT('Ctrl Pts',(-4.65680224173408,-4.12963019580917,
-3.17570098185821));
#71291=CARTESIAN_POINT('Ctrl Pts',(-4.61840900652908,-2.82584471571655,
-4.0789475365882));
#71292=CARTESIAN_POINT('Ctrl Pts',(-4.57865368239002,-1.47580442627195,
-5.01423885468211));
#71293=CARTESIAN_POINT('Ctrl Pts',(-4.53889835825097,0.384678063507157,
-5.212735633414));
#71294=CARTESIAN_POINT('Ctrl Pts',(-4.49914303411192,1.90165751480054,-4.58332958229983));
#71295=CARTESIAN_POINT('Ctrl Pts',(-4.45938770997286,3.41863696609391,-3.95392353118567));
#71296=CARTESIAN_POINT('Ctrl Pts',(-4.4196323858338,4.59211337890157,-2.49661465022554));
#71297=CARTESIAN_POINT('Ctrl Pts',(-4.37987706169475,4.88347131282572,-0.88029500759142));
#71298=CARTESIAN_POINT('Ctrl Pts',(-4.34012173755569,5.17482924674987,0.736024635042727));
#71299=CARTESIAN_POINT('Ctrl Pts',(-4.30036641341664,4.58406870179042,2.5113550393509));
#71300=CARTESIAN_POINT('Ctrl Pts',(-4.26061108927758,3.3823436164673,3.63083503119117));
#71301=CARTESIAN_POINT('Ctrl Pts',(-4.22085576513853,2.18061853114421,4.75031502303142));
#71302=CARTESIAN_POINT('Ctrl Pts',(-4.18110044099947,0.367928905457532,
5.21394460240387));
#71303=CARTESIAN_POINT('Ctrl Pts',(-4.14134511686042,-1.22371652962239,
4.80892183537132));
#71304=CARTESIAN_POINT('Ctrl Pts',(-4.10158979272137,-2.81536196470231,
4.40389906833878));
#71305=CARTESIAN_POINT('Ctrl Pts',(-4.06183446858231,-4.18596320917542,
3.13022395490121));
#71306=CARTESIAN_POINT('Ctrl Pts',(-4.02207914444326,-4.70642624389953,
1.57250226528164));
#71307=CARTESIAN_POINT('Ctrl Pts',(-4.00924900034353,-4.87439407911917,
1.06978233586574));
#71308=CARTESIAN_POINT('Ctrl Pts',(-3.9964188562438,-4.95381732933038,0.537478056608055));
#71309=CARTESIAN_POINT('Ctrl Pts',(-3.98358871214407,-4.94978226424517,
0.00400445798880121));
#71310=CARTESIAN_POINT('Origin',(10.45,0.,0.));
#71311=CARTESIAN_POINT('',(-3.12821128785576,-4.94661592217658,-0.00204876029963219));
#71312=CARTESIAN_POINT('',(-3.23358871214408,-4.94744349501179,-0.00282914305488679));
#71313=CARTESIAN_POINT('',(10.45,-4.954,-6.06690024297599E-16));
#71314=CARTESIAN_POINT('Ctrl Pts',(-3.12821128785576,-4.94661592217658,
-0.00204876029963219));
#71315=CARTESIAN_POINT('Ctrl Pts',(-3.15117097390638,-4.94306604476936,
0.954142296727101));
#71316=CARTESIAN_POINT('Ctrl Pts',(-3.17413065995699,-4.67616316064024,
1.91216596896721));
#71317=CARTESIAN_POINT('Ctrl Pts',(-3.1970903460076,-4.15870819221125,2.70709380384627));
#71318=CARTESIAN_POINT('Ctrl Pts',(-3.23684567014666,-3.26272076660311,
4.08353308411823));
#71319=CARTESIAN_POINT('Ctrl Pts',(-3.27660099428571,-1.61553135584163,
4.97098055600742));
#71320=CARTESIAN_POINT('Ctrl Pts',(-3.31635631842476,0.0268144645398234,
4.96210556873584));
#71321=CARTESIAN_POINT('Ctrl Pts',(-3.35611164256382,1.66916028492123,4.95323058146427));
#71322=CARTESIAN_POINT('Ctrl Pts',(-3.39586696670287,3.30666251492261,4.04803313503198));
#71323=CARTESIAN_POINT('Ctrl Pts',(-3.43562229084193,4.18772191050428,2.66199096374692));
#71324=CARTESIAN_POINT('Ctrl Pts',(-3.47537761498098,5.06878130608597,1.27594879246181));
#71325=CARTESIAN_POINT('Ctrl Pts',(-3.51513293912004,5.1933978672479,-0.590938103676095));
#71326=CARTESIAN_POINT('Ctrl Pts',(-3.55488826325909,4.50437367911208,-2.08178491917636));
#71327=CARTESIAN_POINT('Ctrl Pts',(-3.59464358739815,3.81534949097627,-3.57263173467662));
#71328=CARTESIAN_POINT('Ctrl Pts',(-3.6343989115372,2.3126845535427,-4.68743846953923));
#71329=CARTESIAN_POINT('Ctrl Pts',(-3.67415423567626,0.686088969385792,
-4.91451855392519));
#71330=CARTESIAN_POINT('Ctrl Pts',(-3.71390955981531,-0.940506614771073,
-5.14159863831115));
#71331=CARTESIAN_POINT('Ctrl Pts',(-3.75366488395437,-2.69103284565128,
-4.4809520722205));
#71332=CARTESIAN_POINT('Ctrl Pts',(-3.79342020809342,-3.76201344841635,
-3.23580986844443));
#71333=CARTESIAN_POINT('Ctrl Pts',(-3.82168390134754,-4.52341755951813,
-2.35058711985895));
#71334=CARTESIAN_POINT('Ctrl Pts',(-3.84994759460165,-4.94135401375244,
-1.16993851785152));
#71335=CARTESIAN_POINT('Ctrl Pts',(-3.87821128785577,-4.95126260644063,
0.00436986867149824));
#71336=CARTESIAN_POINT('Ctrl Pts',(-3.98358871214407,-4.94978226424517,
0.00400445798880121));
#71337=CARTESIAN_POINT('Ctrl Pts',(-3.95666353210474,-4.94131432709302,
-1.11553656800441));
#71338=CARTESIAN_POINT('Ctrl Pts',(-3.92973835206541,-4.56529016919644,
-2.24022735773114));
#71339=CARTESIAN_POINT('Ctrl Pts',(-3.90281317202609,-3.86871874929071,
-3.10744695891477));
#71340=CARTESIAN_POINT('Ctrl Pts',(-3.86305784788703,-2.84022339498269,
-4.38790622769));
#71341=CARTESIAN_POINT('Ctrl Pts',(-3.82330252374798,-1.11290786139162,
-5.10705649943884));
#71342=CARTESIAN_POINT('Ctrl Pts',(-3.78354719960893,0.520405084295247,
-4.93481407064357));
#71343=CARTESIAN_POINT('Ctrl Pts',(-3.74379187546987,2.15371802998204,-4.76257164184831));
#71344=CARTESIAN_POINT('Ctrl Pts',(-3.70403655133082,3.69302838776461,-3.698936512509));
#71345=CARTESIAN_POINT('Ctrl Pts',(-3.66428122719176,4.43180612668787,-2.23210793176182));
#71346=CARTESIAN_POINT('Ctrl Pts',(-3.6245259030527,5.17058386561115,-0.76527935101459));
#71347=CARTESIAN_POINT('Ctrl Pts',(-3.58477057891365,5.10882898567509,1.10474268114056));
#71348=CARTESIAN_POINT('Ctrl Pts',(-3.5450152547746,4.27488643824851,2.5196343591206));
#71349=CARTESIAN_POINT('Ctrl Pts',(-3.50525993063554,3.44094389082193,3.93452603710064));
#71350=CARTESIAN_POINT('Ctrl Pts',(-3.46550460649649,1.8348136759048,4.89428736090561));
#71351=CARTESIAN_POINT('Ctrl Pts',(-3.42574928235743,0.193695556186975,
4.95839625232752));
#71352=CARTESIAN_POINT('Ctrl Pts',(-3.38599395821838,-1.44742256353083,
5.02250514374942));
#71353=CARTESIAN_POINT('Ctrl Pts',(-3.34623863407933,-3.1235285880493,4.19096160278835));
#71354=CARTESIAN_POINT('Ctrl Pts',(-3.30648330994027,-4.06530446828262,
2.84543686342598));
#71355=CARTESIAN_POINT('Ctrl Pts',(-3.28218511067487,-4.64091184910068,
2.02306076810869));
#71356=CARTESIAN_POINT('Ctrl Pts',(-3.25788691140947,-4.94220462071748,
1.00868308784557));
#71357=CARTESIAN_POINT('Ctrl Pts',(-3.23358871214408,-4.94744349501179,
-0.00282914305488679));
#71358=CARTESIAN_POINT('Origin',(10.45,0.,0.));
#71359=CARTESIAN_POINT('',(-2.37821128785577,-4.95878862246057,-0.00355106645011816));
#71360=CARTESIAN_POINT('',(-2.48358871214407,-4.9601430818857,-0.00283985261795904));
#71361=CARTESIAN_POINT('',(10.45,-4.954,-6.06690024297599E-16));
#71362=CARTESIAN_POINT('Ctrl Pts',(-2.37821128785577,-4.95878862246057,
-0.00355106645011816));
#71363=CARTESIAN_POINT('Ctrl Pts',(-2.41263902907205,-4.9472554647168,1.42129552477773));
#71364=CARTESIAN_POINT('Ctrl Pts',(-2.44706677028833,-4.30040375105269,
2.85527758425018));
#71365=CARTESIAN_POINT('Ctrl Pts',(-2.48149451150461,-3.21767241276599,
3.77753821091363));
#71366=CARTESIAN_POINT('Ctrl Pts',(-2.52124983564367,-1.96739186026945,
4.84251572202474));
#71367=CARTESIAN_POINT('Ctrl Pts',(-2.56100515978272,-0.135891902052169,
5.22514331295018));
#71368=CARTESIAN_POINT('Ctrl Pts',(-2.60076048392178,1.43618495231579,4.74979825608725));
#71369=CARTESIAN_POINT('Ctrl Pts',(-2.64051580806083,3.00826180668371,4.27445319922434));
#71370=CARTESIAN_POINT('Ctrl Pts',(-2.68027113219989,4.32091555720235,2.94113549457312));
#71371=CARTESIAN_POINT('Ctrl Pts',(-2.72002645633894,4.77164957913437,1.36182634162164));
#71372=CARTESIAN_POINT('Ctrl Pts',(-2.75978178047799,5.22238360106641,-0.2174828113299));
#71373=CARTESIAN_POINT('Ctrl Pts',(-2.79953710461705,4.8111978944118,-2.04278341258168));
#71374=CARTESIAN_POINT('Ctrl Pts',(-2.8392924287561,3.72682311285719,-3.27627840335056));
#71375=CARTESIAN_POINT('Ctrl Pts',(-2.87904775289516,2.64244833130259,-4.50977339411943));
#71376=CARTESIAN_POINT('Ctrl Pts',(-2.91880307703422,0.884884474847997,
-5.15146277440537));
#71377=CARTESIAN_POINT('Ctrl Pts',(-2.95855840117327,-0.739161972899706,
-4.90681671438896));
#71378=CARTESIAN_POINT('Ctrl Pts',(-2.99831372531233,-2.36320842064736,
-4.66217065437255));
#71379=CARTESIAN_POINT('Ctrl Pts',(-3.03806904945138,-3.85373745968816,
-3.53118915405384));
#71380=CARTESIAN_POINT('Ctrl Pts',(-3.07782437359043,-4.52660925898116,
-2.03298285956715));
#71381=CARTESIAN_POINT('Ctrl Pts',(-3.09462001167887,-4.81088089971325,
-1.40002787180222));
#71382=CARTESIAN_POINT('Ctrl Pts',(-3.11141564976732,-4.94921275455742,
-0.701528661802854));
#71383=CARTESIAN_POINT('Ctrl Pts',(-3.12821128785576,-4.94661592217658,
-0.00204876029963219));
#71384=CARTESIAN_POINT('Ctrl Pts',(-3.23358871214408,-4.94744349501179,
-0.00282914305488679));
#71385=CARTESIAN_POINT('Ctrl Pts',(-3.21813158727042,-4.95077616725141,
-0.646295380757791));
#71386=CARTESIAN_POINT('Ctrl Pts',(-3.20267446239676,-4.83430243494921,
-1.28860203505834));
#71387=CARTESIAN_POINT('Ctrl Pts',(-3.1872173375231,-4.59242589231839,-1.87958393990419));
#71388=CARTESIAN_POINT('Ctrl Pts',(-3.14746201338405,-3.97032570017272,
-3.39957406610822));
#71389=CARTESIAN_POINT('Ctrl Pts',(-3.107706689245,-2.51867957993331,-4.5800483807526));
#71390=CARTESIAN_POINT('Ctrl Pts',(-3.06795136510594,-0.903780441982408,
-4.87917946752035));
#71391=CARTESIAN_POINT('Ctrl Pts',(-3.02819604096689,0.711118695968514,
-5.17831055428811));
#71392=CARTESIAN_POINT('Ctrl Pts',(-2.98844071682783,2.48927085163095,-4.59609841317917));
#71393=CARTESIAN_POINT('Ctrl Pts',(-2.94868539268878,3.61451969159798,-3.39977333989084));
#71394=CARTESIAN_POINT('Ctrl Pts',(-2.90893006854972,4.73976853156503,-2.20344826660249));
#71395=CARTESIAN_POINT('Ctrl Pts',(-2.86917474441066,5.2121140558367,-0.393010261134748));
#71396=CARTESIAN_POINT('Ctrl Pts',(-2.82941942027161,4.8147537877728,1.20056541958762));
#71397=CARTESIAN_POINT('Ctrl Pts',(-2.78966409613256,4.41739351970892,2.79414110030994));
#71398=CARTESIAN_POINT('Ctrl Pts',(-2.7499087719935,3.15032745930952,4.17085445628686));
#71399=CARTESIAN_POINT('Ctrl Pts',(-2.71015344785445,1.59512787908609,4.6988060624955));
#71400=CARTESIAN_POINT('Ctrl Pts',(-2.67039812371539,0.0399282988626437,
5.22675766870414));
#71401=CARTESIAN_POINT('Ctrl Pts',(-2.63064279957634,-1.80340480118489,
4.90594752514445));
#71402=CARTESIAN_POINT('Ctrl Pts',(-2.59088747543728,-3.08879760257501,
3.88362469014566));
#71403=CARTESIAN_POINT('Ctrl Pts',(-2.55512122100621,-4.2452134279769,2.96388225516099));
#71404=CARTESIAN_POINT('Ctrl Pts',(-2.51935496657514,-4.95003952369581,
1.47634443515309));
#71405=CARTESIAN_POINT('Ctrl Pts',(-2.48358871214407,-4.9601430818857,-0.00283985261795904));
#71406=CARTESIAN_POINT('Origin',(10.45,0.,0.));
#71407=CARTESIAN_POINT('',(-1.62821128785576,-4.95786674368922,0.00389817196716477));
#71408=CARTESIAN_POINT('',(-1.73358871214408,-4.95624245093516,0.0043165021388984));
#71409=CARTESIAN_POINT('',(10.45,-4.954,-6.06690024297599E-16));
#71410=CARTESIAN_POINT('Ctrl Pts',(-1.62821128785576,-4.95786674368922,
0.00389817196716477));
#71411=CARTESIAN_POINT('Ctrl Pts',(-1.63435176009866,-4.96006131004143,
0.258154385410107));
#71412=CARTESIAN_POINT('Ctrl Pts',(-1.64049223234156,-4.94219726502405,
0.512101374217645));
#71413=CARTESIAN_POINT('Ctrl Pts',(-1.64663270458446,-4.90320362582084,
0.762761361452733));
#71414=CARTESIAN_POINT('Ctrl Pts',(-1.68638802872351,-4.6507466966851,2.38561195779698));
#71415=CARTESIAN_POINT('Ctrl Pts',(-1.72614335286257,-3.51260697205389,
3.87068230545853));
#71416=CARTESIAN_POINT('Ctrl Pts',(-1.76589867700162,-2.01118066059901,
4.53633806513804));
#71417=CARTESIAN_POINT('Ctrl Pts',(-1.80565400114068,-0.509754349144126,
5.20199382481756));
#71418=CARTESIAN_POINT('Ctrl Pts',(-1.84540932527974,1.35495854913438,5.04823499651502));
#71419=CARTESIAN_POINT('Ctrl Pts',(-1.88516464941879,2.72707107480563,4.14563554159628));
#71420=CARTESIAN_POINT('Ctrl Pts',(-1.92491997355785,4.09918360047684,3.24303608667757));
#71421=CARTESIAN_POINT('Ctrl Pts',(-1.9646752976969,4.97869575354077,1.59159600514272));
#71422=CARTESIAN_POINT('Ctrl Pts',(-2.00443062183595,4.96191912536181,-0.0506881066571491));
#71423=CARTESIAN_POINT('Ctrl Pts',(-2.04418594597501,4.94514249718285,-1.69297221845702));
#71424=CARTESIAN_POINT('Ctrl Pts',(-2.08394127011406,4.03207708776091,-3.32610036052202));
#71425=CARTESIAN_POINT('Ctrl Pts',(-2.12369659425312,2.64181195780517,-4.20048095703164));
#71426=CARTESIAN_POINT('Ctrl Pts',(-2.16345191839217,1.25154682784939,-5.07486155354129));
#71427=CARTESIAN_POINT('Ctrl Pts',(-2.20320724253123,-0.61591802264022,
-5.19049460449564));
#71428=CARTESIAN_POINT('Ctrl Pts',(-2.24296256667028,-2.10343251216577,
-4.49430554786297));
#71429=CARTESIAN_POINT('Ctrl Pts',(-2.28271789080934,-3.59094700169127,
-3.79811649123032));
#71430=CARTESIAN_POINT('Ctrl Pts',(-2.32247321494839,-4.69851113025268,
-2.29010532701072));
#71431=CARTESIAN_POINT('Ctrl Pts',(-2.36222853908745,-4.91776262114551,
-0.662436029252524));
#71432=CARTESIAN_POINT('Ctrl Pts',(-2.36755612201022,-4.9471443586604,-0.444313215706146));
#71433=CARTESIAN_POINT('Ctrl Pts',(-2.37288370493299,-4.96057334176166,
-0.224041522658353));
#71434=CARTESIAN_POINT('Ctrl Pts',(-2.37821128785577,-4.95878862246057,
-0.00355106645011816));
#71435=CARTESIAN_POINT('Ctrl Pts',(-2.48358871214407,-4.9601430818857,-0.00283985261795904));
#71436=CARTESIAN_POINT('Ctrl Pts',(-2.47959964243609,-4.96126994849667,
-0.167815730823135));
#71437=CARTESIAN_POINT('Ctrl Pts',(-2.4756105727281,-4.9537549453676,-0.332687696842427));
#71438=CARTESIAN_POINT('Ctrl Pts',(-2.47162150302012,-4.93726075563198,
-0.496656414917237));
#71439=CARTESIAN_POINT('Ctrl Pts',(-2.43186617888106,-4.77287860456607,
-2.13077915854342));
#71440=CARTESIAN_POINT('Ctrl Pts',(-2.39211085474201,-3.71666179970155,
-3.67518911935791));
#71441=CARTESIAN_POINT('Ctrl Pts',(-2.35235553060295,-2.25340464393075,
-4.42101559308418));
#71442=CARTESIAN_POINT('Ctrl Pts',(-2.3126002064639,-0.790147488159902,
-5.16684206681047));
#71443=CARTESIAN_POINT('Ctrl Pts',(-2.27284488232484,1.0801500185172,-5.11408505344847));
#71444=CARTESIAN_POINT('Ctrl Pts',(-2.23308955818579,2.49903763011426,-4.28695956207369));
#71445=CARTESIAN_POINT('Ctrl Pts',(-2.19333423404673,3.91792524171126,-3.45983407069895));
#71446=CARTESIAN_POINT('Ctrl Pts',(-2.15357890990768,4.88540295822824,-1.85834010131145));
#71447=CARTESIAN_POINT('Ctrl Pts',(-2.11382358576863,4.95740694449176,-0.217549420332463));
#71448=CARTESIAN_POINT('Ctrl Pts',(-2.07406826162957,5.02941093075529,1.42324126064658));
#71449=CARTESIAN_POINT('Ctrl Pts',(-2.03431293749051,4.20594118676532,3.10332865321719));
#71450=CARTESIAN_POINT('Ctrl Pts',(-1.99455761335146,2.86496314409989,4.05156729507624));
#71451=CARTESIAN_POINT('Ctrl Pts',(-1.9548022892124,1.52398510143443,4.99980593693532));
#71452=CARTESIAN_POINT('Ctrl Pts',(-1.91504696507335,-0.334501239906424,
5.21619582808284));
#71453=CARTESIAN_POINT('Ctrl Pts',(-1.8752916409343,-1.85746685582874,4.60141589546955));
#71454=CARTESIAN_POINT('Ctrl Pts',(-1.83553631679524,-3.38043247175097,
3.98663596285629));
#71455=CARTESIAN_POINT('Ctrl Pts',(-1.79578099265619,-4.56787736225463,
2.54068620648225));
#71456=CARTESIAN_POINT('Ctrl Pts',(-1.75602566851713,-4.87477467748886,
0.927244955389617));
#71457=CARTESIAN_POINT('Ctrl Pts',(-1.74854668305945,-4.93250985151514,
0.623715707041817));
#71458=CARTESIAN_POINT('Ctrl Pts',(-1.74106769760176,-4.95908142667506,
0.314258740644999));
#71459=CARTESIAN_POINT('Ctrl Pts',(-1.73358871214408,-4.95624245093516,
0.0043165021388984));
#71460=CARTESIAN_POINT('Origin',(10.45,0.,0.));
#71461=CARTESIAN_POINT('',(-0.878211287855769,-4.9462499908807,0.00153300580362309));
#71462=CARTESIAN_POINT('',(-0.983588712144078,-4.94588532464384,0.00063872631976612));
#71463=CARTESIAN_POINT('',(10.45,-4.954,-6.06690024297599E-16));
#71464=CARTESIAN_POINT('Ctrl Pts',(-0.878211287855769,-4.9462499908807,
0.00153300580362309));
#71465=CARTESIAN_POINT('Ctrl Pts',(-0.895819815264337,-4.94827859092613,
0.735002394484792));
#71466=CARTESIAN_POINT('Ctrl Pts',(-0.913428342672905,-4.79565751940137,
1.46766899677298));
#71467=CARTESIAN_POINT('Ctrl Pts',(-0.931036870081473,-4.48413338106601,
2.1250314142613));
#71468=CARTESIAN_POINT('Ctrl Pts',(-0.970792194220528,-3.78079557153196,
3.60917914437558));
#71469=CARTESIAN_POINT('Ctrl Pts',(-1.01054751835958,-2.26747308842599,
4.70947502840552));
#71470=CARTESIAN_POINT('Ctrl Pts',(-1.05030284249864,-0.638767754849003,
4.92089285050518));
#71471=CARTESIAN_POINT('Ctrl Pts',(-1.09005816663769,0.989937578727986,
5.13231067260483));
#71472=CARTESIAN_POINT('Ctrl Pts',(-1.12981349077675,2.73402576277599,4.4548504327742));
#71473=CARTESIAN_POINT('Ctrl Pts',(-1.1695688149158,3.79297552981071,3.19946047343064));
#71474=CARTESIAN_POINT('Ctrl Pts',(-1.20932413905486,4.85192529684539,1.94407051408712));
#71475=CARTESIAN_POINT('Ctrl Pts',(-1.24907946319391,5.22573664686682,0.110750835230702));
#71476=CARTESIAN_POINT('Ctrl Pts',(-1.28883478733297,4.7428334299669,-1.45902081766377));
#71477=CARTESIAN_POINT('Ctrl Pts',(-1.32859011147202,4.25993021306696,-3.02879247055829));
#71478=CARTESIAN_POINT('Ctrl Pts',(-1.36834543561108,2.92031242924562,-4.33501609749086));
#71479=CARTESIAN_POINT('Ctrl Pts',(-1.40810075975013,1.33885295939138,-4.77814644437744));
#71480=CARTESIAN_POINT('Ctrl Pts',(-1.44785608388919,-0.242606510462868,
-5.22127679126403));
#71481=CARTESIAN_POINT('Ctrl Pts',(-1.48761140802824,-2.06590766635002,
-4.80131385810463));
#71482=CARTESIAN_POINT('Ctrl Pts',(-1.5273667321673,-3.29417117747345,-3.71101696901146));
#71483=CARTESIAN_POINT('Ctrl Pts',(-1.56098158406345,-4.33272128139038,
-2.78912363161815));
#71484=CARTESIAN_POINT('Ctrl Pts',(-1.59459643595961,-4.94585300598505,
-1.38797929616193));
#71485=CARTESIAN_POINT('Ctrl Pts',(-1.62821128785576,-4.95786674368922,
0.00389817196716477));
#71486=CARTESIAN_POINT('Ctrl Pts',(-1.73358871214408,-4.95624245093516,
0.0043165021388984));
#71487=CARTESIAN_POINT('Ctrl Pts',(-1.70131237346271,-4.94399055620857,
-1.33327142583419));
#71488=CARTESIAN_POINT('Ctrl Pts',(-1.66903603478134,-4.38398371281437,
-2.67989727357355));
#71489=CARTESIAN_POINT('Ctrl Pts',(-1.63675969609996,-3.41712436432993,
-3.59812068200678));
#71490=CARTESIAN_POINT('Ctrl Pts',(-1.59700437196091,-2.22622699597197,
-4.72911232249915));
#71491=CARTESIAN_POINT('Ctrl Pts',(-1.55724904782185,-0.418082519291285,
-5.21016285767256));
#71492=CARTESIAN_POINT('Ctrl Pts',(-1.5174937236828,1.17738651850033,-4.82047428679334));
#71493=CARTESIAN_POINT('Ctrl Pts',(-1.47773839954375,2.77285555629184,-4.43078571591415));
#71494=CARTESIAN_POINT('Ctrl Pts',(-1.4379830754047,4.15564915519426,-3.17035803898244));
#71495=CARTESIAN_POINT('Ctrl Pts',(-1.39822775126564,4.69107711170357,-1.61771656838675));
#71496=CARTESIAN_POINT('Ctrl Pts',(-1.35847242712659,5.22650506821291,-0.0650750977909698));
#71497=CARTESIAN_POINT('Ctrl Pts',(-1.31871710298753,4.91456738232895,1.77978016646891));
#71498=CARTESIAN_POINT('Ctrl Pts',(-1.27896177884847,3.89844073167842,3.07007674581154));
#71499=CARTESIAN_POINT('Ctrl Pts',(-1.23920645470942,2.88231408102786,4.36037332515421));
#71500=CARTESIAN_POINT('Ctrl Pts',(-1.19945113057036,1.16199846561071,5.09611121957971));
#71501=CARTESIAN_POINT('Ctrl Pts',(-1.1596958064313,-0.472896248786042,
4.93959315141097));
#71502=CARTESIAN_POINT('Ctrl Pts',(-1.11994048229225,-2.10779096318271,
4.78307508324224));
#71503=CARTESIAN_POINT('Ctrl Pts',(-1.0801851581532,-3.65726477655895,3.73430105247941));
#71504=CARTESIAN_POINT('Ctrl Pts',(-1.04042983401414,-4.41012272047075,
2.27464919360542));
#71505=CARTESIAN_POINT('Ctrl Pts',(-1.02148279339079,-4.76892824792712,
1.57899185298591));
#71506=CARTESIAN_POINT('Ctrl Pts',(-1.00253575276743,-4.94679104943383,
0.79000803331864));
#71507=CARTESIAN_POINT('Ctrl Pts',(-0.983588712144078,-4.94588532464384,
0.00063872631976612));
#71508=CARTESIAN_POINT('Origin',(10.45,0.,0.));
#71509=CARTESIAN_POINT('',(-0.12821128785577,-4.95222891719584,-0.00450272491899106));
#71510=CARTESIAN_POINT('',(-0.23358871214408,-4.95389107247016,-0.00456502003026654));
#71511=CARTESIAN_POINT('',(10.45,-4.954,-6.06690024297599E-16));
#71512=CARTESIAN_POINT('Ctrl Pts',(-0.12821128785577,-4.95222891719584,
-0.00450272491899106));
#71513=CARTESIAN_POINT('Ctrl Pts',(-0.157287870430009,-4.94156622804037,
1.20298200617453));
#71514=CARTESIAN_POINT('Ctrl Pts',(-0.186364453004247,-4.49686831089669,
2.41749706190262));
#71515=CARTESIAN_POINT('Ctrl Pts',(-0.215441035578485,-3.69512492141951,
3.31198769712273));
#71516=CARTESIAN_POINT('Ctrl Pts',(-0.255196359717539,-2.59893116331091,
4.53499129638443));
#71517=CARTESIAN_POINT('Ctrl Pts',(-0.294951683856594,-0.8352740853285,
5.15973899071356));
#71518=CARTESIAN_POINT('Ctrl Pts',(-0.334707007995648,0.786343093374425,
4.89947703640809));
#71519=CARTESIAN_POINT('Ctrl Pts',(-0.374462332134704,2.40796027207744,
4.6392150821026));
#71520=CARTESIAN_POINT('Ctrl Pts',(-0.41421765627376,3.88753755150096,3.4939434791624));
#71521=CARTESIAN_POINT('Ctrl Pts',(-0.453972980412816,4.54596186276556,
1.98933190621096));
#71522=CARTESIAN_POINT('Ctrl Pts',(-0.49372830455187,5.20438617403012,0.484720333259615));
#71523=CARTESIAN_POINT('Ctrl Pts',(-0.533483628690924,5.04165751713587,
-1.37923120970292));
#71524=CARTESIAN_POINT('Ctrl Pts',(-0.573238952829979,4.13246692655254,
-2.74698521869653));
#71525=CARTESIAN_POINT('Ctrl Pts',(-0.612994276969034,3.22327633596919,
-4.11473922769018));
#71526=CARTESIAN_POINT('Ctrl Pts',(-0.65274960110809,1.56762381169672,-4.98629570271487));
#71527=CARTESIAN_POINT('Ctrl Pts',(-0.692504925247145,-0.0745605754309484,
-4.96161782197896));
#71528=CARTESIAN_POINT('Ctrl Pts',(-0.732260249386201,-1.71674496255866,
-4.93693994124305));
#71529=CARTESIAN_POINT('Ctrl Pts',(-0.772015573525258,-3.34546121254158,
-4.01602770474649));
#71530=CARTESIAN_POINT('Ctrl Pts',(-0.811770897664314,-4.21314276955191,
-2.62157179839887));
#71531=CARTESIAN_POINT('Ctrl Pts',(-0.833917694394799,-4.69650864534464,
-1.84475178305996));
#71532=CARTESIAN_POINT('Ctrl Pts',(-0.856064491125284,-4.94369855703214,
-0.920974429500177));
#71533=CARTESIAN_POINT('Ctrl Pts',(-0.878211287855769,-4.9462499908807,
0.00153300580362309));
#71534=CARTESIAN_POINT('Ctrl Pts',(-0.983588712144078,-4.94588532464384,
0.00063872631976612));
#71535=CARTESIAN_POINT('Ctrl Pts',(-0.962780428628378,-4.94489062691812,
-0.866273456175758));
#71536=CARTESIAN_POINT('Ctrl Pts',(-0.941972145112679,-4.72828002074546,
-1.73365058181824));
#71537=CARTESIAN_POINT('Ctrl Pts',(-0.921163861596979,-4.29893345005872,
-2.47838305262693));
#71538=CARTESIAN_POINT('Ctrl Pts',(-0.881408537457925,-3.47864416128752,
-3.90123375300017));
#71539=CARTESIAN_POINT('Ctrl Pts',(-0.841653213318871,-1.88182350929776,
-4.87640546676153));
#71540=CARTESIAN_POINT('Ctrl Pts',(-0.801897889179817,-0.241398248577849,
-4.95630288109652));
#71541=CARTESIAN_POINT('Ctrl Pts',(-0.762142565040761,1.39902701214211,
-5.03620029543151));
#71542=CARTESIAN_POINT('Ctrl Pts',(-0.722387240901707,3.08305688159219,
-4.22082341034007));
#71543=CARTESIAN_POINT('Ctrl Pts',(-0.682631916762651,4.0377363349613,-2.88442310573802));
#71544=CARTESIAN_POINT('Ctrl Pts',(-0.642876592623596,4.99241578833041,
-1.54802280113598));
#71545=CARTESIAN_POINT('Ctrl Pts',(-0.603121268484537,5.21774482561852,
0.309400922976757));
#71546=CARTESIAN_POINT('Ctrl Pts',(-0.563365944345481,4.61029938364994,
1.83530677454728));
#71547=CARTESIAN_POINT('Ctrl Pts',(-0.523610620206427,4.00285394168137,
3.36121262611776));
#71548=CARTESIAN_POINT('Ctrl Pts',(-0.483855296067373,2.56263402045623,
4.55560060514614));
#71549=CARTESIAN_POINT('Ctrl Pts',(-0.444099971928319,0.950688004649234,
4.87025704469468));
#71550=CARTESIAN_POINT('Ctrl Pts',(-0.404344647789265,-0.661258011157765,
5.18491348424322));
#71551=CARTESIAN_POINT('Ctrl Pts',(-0.364589323650211,-2.44493012154658,
4.61983838431192));
#71552=CARTESIAN_POINT('Ctrl Pts',(-0.324833999511157,-3.58163838202674,
3.43439628813785));
#71553=CARTESIAN_POINT('Ctrl Pts',(-0.294418903722131,-4.45128518721321,
2.52746531251895));
#71554=CARTESIAN_POINT('Ctrl Pts',(-0.264003807933106,-4.94225598096154,
1.25742579567596));
#71555=CARTESIAN_POINT('Ctrl Pts',(-0.23358871214408,-4.95389107247016,
-0.00456502003026654));
#71556=CARTESIAN_POINT('Origin',(10.45,0.,0.));
#71557=CARTESIAN_POINT('',(0.621788712144221,-4.9620854618724,0.000611260038189503));
#71558=CARTESIAN_POINT('',(0.516411287855919,-4.96154487360443,0.00161152755429558));
#71559=CARTESIAN_POINT('',(10.45,-4.954,-6.06690024297599E-16));
#71560=CARTESIAN_POINT('Ctrl Pts',(0.621788712144221,-4.9620854618724,0.000611260038189503));
#71561=CARTESIAN_POINT('Ctrl Pts',(0.620999398543369,-4.96214205437354,
0.0332209798384553));
#71562=CARTESIAN_POINT('Ctrl Pts',(0.620210084942517,-4.96184848967099,
0.0658296534178576));
#71563=CARTESIAN_POINT('Ctrl Pts',(0.619420771341666,-4.96120166556195,
0.0984313182539327));
#71564=CARTESIAN_POINT('Ctrl Pts',(0.579665447202611,-4.92862310352016,
1.7404779669271));
#71565=CARTESIAN_POINT('Ctrl Pts',(0.539910123063554,-3.9998853575048,3.36474462281019));
#71566=CARTESIAN_POINT('Ctrl Pts',(0.500154798924499,-2.60127095405371,
4.2257070549654));
#71567=CARTESIAN_POINT('Ctrl Pts',(0.460399474785444,-1.20265655060261,
5.08666948712061));
#71568=CARTESIAN_POINT('Ctrl Pts',(0.420644150646389,0.665834510284238,
5.18432769554799));
#71569=CARTESIAN_POINT('Ctrl Pts',(0.380888826507334,2.14658112548541,4.47385741418942));
#71570=CARTESIAN_POINT('Ctrl Pts',(0.34113350236828,3.62732774068654,3.76338713283087));
#71571=CARTESIAN_POINT('Ctrl Pts',(0.301378178229225,4.72032991020208,2.24478836168642));
#71572=CARTESIAN_POINT('Ctrl Pts',(0.261622854090171,4.92390916954468,0.61508469405576));
#71573=CARTESIAN_POINT('Ctrl Pts',(0.221867529951116,5.12748842888729,-1.01461897357494));
#71574=CARTESIAN_POINT('Ctrl Pts',(0.182112205812063,4.441644778057,-2.7554275376918));
#71575=CARTESIAN_POINT('Ctrl Pts',(0.142356881673009,3.18117447201399,-3.80832504775976));
#71576=CARTESIAN_POINT('Ctrl Pts',(0.102601557533955,1.92070416597101,-4.86122255782768));
#71577=CARTESIAN_POINT('Ctrl Pts',(0.0628462333949009,0.0856072047153433,
-5.22620901384664));
#71578=CARTESIAN_POINT('Ctrl Pts',(0.023090909255847,-1.48182290915536,
-4.73575881529985));
#71579=CARTESIAN_POINT('Ctrl Pts',(-0.0166644148832092,-3.04925302302614,
-4.24530861675302));
#71580=CARTESIAN_POINT('Ctrl Pts',(-0.0564197390222663,-4.34901628951197,
-2.8994217636403));
#71581=CARTESIAN_POINT('Ctrl Pts',(-0.0961750631613226,-4.78453270363744,
-1.31584858498675));
#71582=CARTESIAN_POINT('Ctrl Pts',(-0.106853804726138,-4.90151746817901,
-0.890482446235984));
#71583=CARTESIAN_POINT('Ctrl Pts',(-0.117532546290954,-4.95614492422956,
-0.447966717081306));
#71584=CARTESIAN_POINT('Ctrl Pts',(-0.12821128785577,-4.95222891719584,
-0.00450272491899106));
#71585=CARTESIAN_POINT('Ctrl Pts',(-0.23358871214408,-4.95389107247016,
-0.00456502003026654));
#71586=CARTESIAN_POINT('Ctrl Pts',(-0.224248483794051,-4.95746411436744,
-0.392112127430431));
#71587=CARTESIAN_POINT('Ctrl Pts',(-0.214908255444021,-4.91583320599101,
-0.778900198764109));
#71588=CARTESIAN_POINT('Ctrl Pts',(-0.205568027093992,-4.82608320001309,
-1.15418036291281));
#71589=CARTESIAN_POINT('Ctrl Pts',(-0.165812702954937,-4.44407534694778,
-2.75150582537247));
#71590=CARTESIAN_POINT('Ctrl Pts',(-0.126057378815881,-3.19031523024568,
-4.14034765787489));
#71591=CARTESIAN_POINT('Ctrl Pts',(-0.0863020546768254,-1.64026781029323,
-4.68323957043604));
#71592=CARTESIAN_POINT('Ctrl Pts',(-0.0465467305377712,-0.09022039034083,
-5.22613148299718));
#71593=CARTESIAN_POINT('Ctrl Pts',(-0.00679140639871754,1.75611433286191,
-4.92307347561709));
#71594=CARTESIAN_POINT('Ctrl Pts',(0.0329639177403364,3.05128482198043,
-3.91316653092275));
#71595=CARTESIAN_POINT('Ctrl Pts',(0.0727192418793914,4.346455311099,-2.90325958622838));
#71596=CARTESIAN_POINT('Ctrl Pts',(0.112474566018447,5.09046156613332,-1.18650370421971));
#71597=CARTESIAN_POINT('Ctrl Pts',(0.152229890157502,4.94181120398959,0.449125135908776));
#71598=CARTESIAN_POINT('Ctrl Pts',(0.191985214296558,4.79316084184586,2.08475397603727));
#71599=CARTESIAN_POINT('Ctrl Pts',(0.231740538435613,3.75185386252406,3.63925577428558));
#71600=CARTESIAN_POINT('Ctrl Pts',(0.271495862574668,2.2958410890108,4.39912776099897));
#71601=CARTESIAN_POINT('Ctrl Pts',(0.311251186713722,0.839828315497573,
5.15899974771234));
#71602=CARTESIAN_POINT('Ctrl Pts',(0.351006510852776,-1.03089025220709,
5.12424192289083));
#71603=CARTESIAN_POINT('Ctrl Pts',(0.39076183499183,-2.45767110477701,4.31080782502842));
#71604=CARTESIAN_POINT('Ctrl Pts',(0.430517159130886,-3.88445195734698,
3.49737372716599));
#71605=CARTESIAN_POINT('Ctrl Pts',(0.470272483269942,-4.86729509478217,
1.90526335626261));
#71606=CARTESIAN_POINT('Ctrl Pts',(0.510027807408997,-4.95508408769899,
0.265241488863219));
#71607=CARTESIAN_POINT('Ctrl Pts',(0.512155634224638,-4.95978282371214,
0.177462491124867));
#71608=CARTESIAN_POINT('Ctrl Pts',(0.514283461040279,-4.96191748152808,
0.0895462404344866));
#71609=CARTESIAN_POINT('Ctrl Pts',(0.516411287855919,-4.96154487360443,
0.00161152755429558));
#71610=CARTESIAN_POINT('Origin',(10.45,0.,0.));
#71611=CARTESIAN_POINT('',(1.37178871214422,-4.95039628575946,0.0041823139770486));
#71612=CARTESIAN_POINT('',(1.26641128785591,-4.94901391678264,0.00371957698114467));
#71613=CARTESIAN_POINT('',(10.45,-4.954,-6.06690024297599E-16));
#71614=CARTESIAN_POINT('Ctrl Pts',(1.37178871214422,-4.95039628575946,0.0041823139770486));
#71615=CARTESIAN_POINT('Ctrl Pts',(1.3595313433777,-4.95445714983158,0.513680565467405));
#71616=CARTESIAN_POINT('Ctrl Pts',(1.34727397461118,-4.88211365660348,1.02205349190173));
#71617=CARTESIAN_POINT('Ctrl Pts',(1.33501660584465,-4.72857457585134,1.50459069896108));
#71618=CARTESIAN_POINT('Ctrl Pts',(1.2952612817056,-4.2305887487475,3.06964299046034));
#71619=CARTESIAN_POINT('Ctrl Pts',(1.25550595756654,-2.87846398134063,4.36291580918494));
#71620=CARTESIAN_POINT('Ctrl Pts',(1.21575063342749,-1.29281375092011,4.79080820908328));
#71621=CARTESIAN_POINT('Ctrl Pts',(1.17599530928843,0.292836479500444,5.21870060898162));
#71622=CARTESIAN_POINT('Ctrl Pts',(1.13623998514938,2.1120121729346,4.78121259005364));
#71623=CARTESIAN_POINT('Ctrl Pts',(1.09648466101033,3.32972754987639,3.67914733795509));
#71624=CARTESIAN_POINT('Ctrl Pts',(1.05672933687127,4.54744292681818,2.57708208585653));
#71625=CARTESIAN_POINT('Ctrl Pts',(1.01697401273221,5.16369798726756,0.810439600587436));
#71626=CARTESIAN_POINT('Ctrl Pts',(0.977218688593158,4.89563703241488,-0.80990662278798));
#71627=CARTESIAN_POINT('Ctrl Pts',(0.937463364454104,4.62757607756223,-2.4302528461633));
#71628=CARTESIAN_POINT('Ctrl Pts',(0.89770804031505,3.47519910740752,-3.90430280764505));
#71629=CARTESIAN_POINT('Ctrl Pts',(0.857952716175997,1.96743710216473,-4.55548042908906));
#71630=CARTESIAN_POINT('Ctrl Pts',(0.81819739203694,0.459675096921814,-5.20665805053313));
#71631=CARTESIAN_POINT('Ctrl Pts',(0.778442067897883,-1.40347194340927,
-5.03496333193943));
#71632=CARTESIAN_POINT('Ctrl Pts',(0.738686743758827,-2.76683577454069,
-4.11920265191089));
#71633=CARTESIAN_POINT('Ctrl Pts',(0.699720733220624,-4.10313098937657,
-3.22162374691569));
#71634=CARTESIAN_POINT('Ctrl Pts',(0.660754722682423,-4.95929166230605,
-1.60923137286915));
#71635=CARTESIAN_POINT('Ctrl Pts',(0.621788712144221,-4.9620854618724,0.000611260038189503));
#71636=CARTESIAN_POINT('Ctrl Pts',(0.516411287855919,-4.96154487360443,
0.00161152755429558));
#71637=CARTESIAN_POINT('Ctrl Pts',(0.554038785179335,-4.95495584880843,
-1.55338493607397));
#71638=CARTESIAN_POINT('Ctrl Pts',(0.591666282502749,-4.16432635838302,
-3.11415466245088));
#71639=CARTESIAN_POINT('Ctrl Pts',(0.629293779826165,-2.90381629787506,
-4.02381190810124));
#71640=CARTESIAN_POINT('Ctrl Pts',(0.669049103965218,-1.57202466673599,
-4.98491007377075));
#71641=CARTESIAN_POINT('Ctrl Pts',(0.708804428104274,0.284293443940589,
-5.21917304121447));
#71642=CARTESIAN_POINT('Ctrl Pts',(0.748559752243328,1.81310420902785,-4.61907615122198));
#71643=CARTESIAN_POINT('Ctrl Pts',(0.788315076382382,3.3419149741151,-4.01897926122949));
#71644=CARTESIAN_POINT('Ctrl Pts',(0.828070400521436,4.5432183936131,-2.58452251380076));
#71645=CARTESIAN_POINT('Ctrl Pts',(0.867825724660489,4.8656266737133,-0.974109047094721));
#71646=CARTESIAN_POINT('Ctrl Pts',(0.907581048799544,5.1880349538135,0.636304419611366));
#71647=CARTESIAN_POINT('Ctrl Pts',(0.947336372938597,4.63154809451592,2.42267460559471));
#71648=CARTESIAN_POINT('Ctrl Pts',(0.987091697077652,3.45158871149887,3.56507317319515));
#71649=CARTESIAN_POINT('Ctrl Pts',(1.02684702121671,2.27162932848182,4.70747174079558));
#71650=CARTESIAN_POINT('Ctrl Pts',(1.06660234535576,0.468197421745252,5.20589869001297));
#71651=CARTESIAN_POINT('Ctrl Pts',(1.10635766949482,-1.1309474900082,4.83158039759521));
#71652=CARTESIAN_POINT('Ctrl Pts',(1.14611299363387,-2.73009240176166,4.45726210517745));
#71653=CARTESIAN_POINT('Ctrl Pts',(1.18586831777293,-4.12495031853205,3.21019857112453));
#71654=CARTESIAN_POINT('Ctrl Pts',(1.22562364191198,-4.67529362011846,1.66278108278323));
#71655=CARTESIAN_POINT('Ctrl Pts',(1.23921952389329,-4.86350495381055,1.13358138430474));
#71656=CARTESIAN_POINT('Ctrl Pts',(1.2528154058746,-4.95294485682679,0.56925335383431));
#71657=CARTESIAN_POINT('Ctrl Pts',(1.26641128785591,-4.94901391678264,0.00371957698114467));
#71658=CARTESIAN_POINT('Origin',(10.45,0.,0.));
#71659=CARTESIAN_POINT('',(2.12178871214422,-4.94705618274164,-0.00250727351567559));
#71660=CARTESIAN_POINT('',(2.01641128785591,-4.94803441261571,-0.00322654717566177));
#71661=CARTESIAN_POINT('',(10.45,-4.954,-6.06690024297599E-16));
#71662=CARTESIAN_POINT('Ctrl Pts',(2.12178871214422,-4.94705618274164,-0.00250727351567559));
#71663=CARTESIAN_POINT('Ctrl Pts',(2.09806328821203,-4.94254372780371,0.985354310079251));
#71664=CARTESIAN_POINT('Ctrl Pts',(2.07433786427983,-4.65626453545947,1.97562456187682));
#71665=CARTESIAN_POINT('Ctrl Pts',(2.05061244034764,-4.10584302471708,2.78662228283094));
#71666=CARTESIAN_POINT('Ctrl Pts',(2.01085711620858,-3.18353345354946,4.14556437654064));
#71667=CARTESIAN_POINT('Ctrl Pts',(1.97110179206953,-1.51957111706592,5.00114915495334));
#71668=CARTESIAN_POINT('Ctrl Pts',(1.93134646793047,0.12229978255891,4.96067066574409));
#71669=CARTESIAN_POINT('Ctrl Pts',(1.89159114379142,1.76417068218369,4.92019217653484));
#71670=CARTESIAN_POINT('Ctrl Pts',(1.85183581965237,3.38395014494975,3.98365041970373));
#71671=CARTESIAN_POINT('Ctrl Pts',(1.81208049551331,4.23817352243036,2.58090989469956));
#71672=CARTESIAN_POINT('Ctrl Pts',(1.77232517137425,5.09239689991098,1.17816936969535));
#71673=CARTESIAN_POINT('Ctrl Pts',(1.7325698472352,5.18106419210611,-0.690769923481942));
#71674=CARTESIAN_POINT('Ctrl Pts',(1.69281452309614,4.46347788510464,-2.16808114699834));
#71675=CARTESIAN_POINT('Ctrl Pts',(1.65305919895709,3.7458915781032,-3.64539237051469));
#71676=CARTESIAN_POINT('Ctrl Pts',(1.61330387481804,2.22205167190523,-4.73107552437016));
#71677=CARTESIAN_POINT('Ctrl Pts',(1.57354855067898,0.591387395095607,-4.92681150844132));
#71678=CARTESIAN_POINT('Ctrl Pts',(1.53379322653993,-1.03927688171411,-5.1225474925125));
#71679=CARTESIAN_POINT('Ctrl Pts',(1.49403790240087,-2.77676552913547,-4.42833630679926));
#71680=CARTESIAN_POINT('Ctrl Pts',(1.45428257826181,-3.82358640944574,-3.16281483180562));
#71681=CARTESIAN_POINT('Ctrl Pts',(1.42678462288928,-4.54765128561477,-2.28747916806827));
#71682=CARTESIAN_POINT('Ctrl Pts',(1.39928666751675,-4.94128621808051,-1.13881668105428));
#71683=CARTESIAN_POINT('Ctrl Pts',(1.37178871214422,-4.95039628575946,0.0041823139770486));
#71684=CARTESIAN_POINT('Ctrl Pts',(1.26641128785591,-4.94901391678264,0.00371957698114467));
#71685=CARTESIAN_POINT('Ctrl Pts',(1.29257073001366,-4.94145050906464,-1.08440755917517));
#71686=CARTESIAN_POINT('Ctrl Pts',(1.3187301721714,-4.58822364743875,-2.17699842775093));
#71687=CARTESIAN_POINT('Ctrl Pts',(1.34488961432915,-3.9278017470013,-3.03242226608294));
#71688=CARTESIAN_POINT('Ctrl Pts',(1.3846449384682,-2.92413788589535,-4.33243668397807));
#71689=CARTESIAN_POINT('Ctrl Pts',(1.42440026260725,-1.21098147728112,-5.08469407713871));
#71690=CARTESIAN_POINT('Ctrl Pts',(1.46415558674631,0.425343626546647,-4.94391486202365));
#71691=CARTESIAN_POINT('Ctrl Pts',(1.50391091088537,2.0616687303745,-4.80313564690857));
#71692=CARTESIAN_POINT('Ctrl Pts',(1.54366623502442,3.62116252941581,-3.76931982351759));
#71693=CARTESIAN_POINT('Ctrl Pts',(1.58342155916348,4.38803096918357,-2.31697983959033));
#71694=CARTESIAN_POINT('Ctrl Pts',(1.62317688330253,5.15489940895132,-0.864639855663081));
#71695=CARTESIAN_POINT('Ctrl Pts',(1.66293220744159,5.12914248944555,1.0062242888005));
#71696=CARTESIAN_POINT('Ctrl Pts',(1.70268753158064,4.32258241211102,2.43690226601122));
#71697=CARTESIAN_POINT('Ctrl Pts',(1.7424428557197,3.51602233477653,3.86758024322186));
#71698=CARTESIAN_POINT('Ctrl Pts',(1.78219817985875,1.92865909961348,4.8580720531797));
#71699=CARTESIAN_POINT('Ctrl Pts',(1.8219535039978,0.289078589258305,4.95375059251216));
#71700=CARTESIAN_POINT('Ctrl Pts',(1.86170882813686,-1.35050192109691,5.04942913184462));
#71701=CARTESIAN_POINT('Ctrl Pts',(1.90146415227591,-3.04229970664424,4.25029440055156));
#71702=CARTESIAN_POINT('Ctrl Pts',(1.94121947641497,-4.00979433682249,2.92314227159206));
#71703=CARTESIAN_POINT('Ctrl Pts',(1.96628341356195,-4.61975602436926,2.08643276751731));
#71704=CARTESIAN_POINT('Ctrl Pts',(1.99134735070893,-4.94182652830635,1.03985043263421));
#71705=CARTESIAN_POINT('Ctrl Pts',(2.01641128785591,-4.94803441261571,-0.00322654717566177));
#71706=CARTESIAN_POINT('Origin',(10.45,0.,0.));
#71707=CARTESIAN_POINT('',(2.87178871214422,-4.95959242193685,-0.00316426722878071));
#71708=CARTESIAN_POINT('',(2.76641128785591,-4.96079845433821,-0.0023638398085009));
#71709=CARTESIAN_POINT('',(10.45,-4.954,-6.06690024297599E-16));
#71710=CARTESIAN_POINT('Ctrl Pts',(2.87178871214422,-4.95959242193685,-0.00316426722878071));
#71711=CARTESIAN_POINT('Ctrl Pts',(2.83659523304635,-4.94877395635362,1.45275619981814));
#71712=CARTESIAN_POINT('Ctrl Pts',(2.80140175394849,-4.26913298345277,2.91745981281874));
#71713=CARTESIAN_POINT('Ctrl Pts',(2.76620827485063,-3.14438197780049,3.83875926159369));
#71714=CARTESIAN_POINT('Ctrl Pts',(2.72645295071157,-1.87383862853134,4.87947928001902));
#71715=CARTESIAN_POINT('Ctrl Pts',(2.68669762657252,-0.0353145807779898,
5.22679080605831));
#71716=CARTESIAN_POINT('Ctrl Pts',(2.64694230243346,1.52732366004471,4.72128087792449));
#71717=CARTESIAN_POINT('Ctrl Pts',(2.60718697829441,3.08996190086745,4.21577094979066));
#71718=CARTESIAN_POINT('Ctrl Pts',(2.56743165415535,4.37671433475958,2.85743956748367));
#71719=CARTESIAN_POINT('Ctrl Pts',(2.5276763300163,4.79697281544771,1.26974899040854));
#71720=CARTESIAN_POINT('Ctrl Pts',(2.48792100587724,5.21723129613585,-0.31794158666663));
#71721=CARTESIAN_POINT('Ctrl Pts',(2.44816568173819,4.77099582362001,-2.13499135850988));
#71722=CARTESIAN_POINT('Ctrl Pts',(2.40841035759913,3.66308458847222,-3.34739032508686));
#71723=CARTESIAN_POINT('Ctrl Pts',(2.36865503346008,2.5551733533245,-4.55978929166377));
#71724=CARTESIAN_POINT('Ctrl Pts',(2.32889970932102,0.785586355544888,-5.16753745297437));
#71725=CARTESIAN_POINT('Ctrl Pts',(2.28914438518197,-0.833451404237114,
-4.89168370273089));
#71726=CARTESIAN_POINT('Ctrl Pts',(2.24938906104291,-2.45248916401921,-4.6158299524874));
#71727=CARTESIAN_POINT('Ctrl Pts',(2.20963373690386,-3.92097768580372,-3.45637429068971));
#71728=CARTESIAN_POINT('Ctrl Pts',(2.1698784127648,-4.56489354377007,-1.9454967552875));
#71729=CARTESIAN_POINT('Ctrl Pts',(2.15384851255794,-4.82452938295254,-1.33628989704205));
#71730=CARTESIAN_POINT('Ctrl Pts',(2.13781861235108,-4.95010498821503,-0.669948354799339));
#71731=CARTESIAN_POINT('Ctrl Pts',(2.12178871214422,-4.94705618274164,-0.00250727351567559));
#71732=CARTESIAN_POINT('Ctrl Pts',(2.01641128785591,-4.94803441261571,-0.00322654717566177));
#71733=CARTESIAN_POINT('Ctrl Pts',(2.03110267484798,-4.95167320369055,-0.61463278726675));
#71734=CARTESIAN_POINT('Ctrl Pts',(2.04579406184006,-4.8467881316361,-1.22483465985581));
#71735=CARTESIAN_POINT('Ctrl Pts',(2.06048544883214,-4.62774599501834,-1.79085967322227));
#71736=CARTESIAN_POINT('Ctrl Pts',(2.10024077297119,-4.03501154822675,-3.32253996245104));
#71737=CARTESIAN_POINT('Ctrl Pts',(2.13999609711024,-2.60635117983441,-4.5307310142827));
#71738=CARTESIAN_POINT('Ctrl Pts',(2.17975142124929,-0.997507540568686,
-4.86088367172994));
#71739=CARTESIAN_POINT('Ctrl Pts',(2.21950674538835,0.611336098697178,-5.19103632917721));
#71740=CARTESIAN_POINT('Ctrl Pts',(2.25926206952741,2.40036300883642,-4.64315059223988));
#71741=CARTESIAN_POINT('Ctrl Pts',(2.29901739366647,3.54842543896859,-3.46870123643745));
#71742=CARTESIAN_POINT('Ctrl Pts',(2.33877271780552,4.69648786910072,-2.29425188063505));
#71743=CARTESIAN_POINT('Ctrl Pts',(2.37852804194458,5.20358581922579,-0.493238905967473));
#71744=CARTESIAN_POINT('Ctrl Pts',(2.41828336608364,4.83696575228884,1.10768843758836));
#71745=CARTESIAN_POINT('Ctrl Pts',(2.45803869022269,4.47034568535192,2.7086157811441));
#71746=CARTESIAN_POINT('Ctrl Pts',(2.49779401436174,3.23000760135317,4.10945749358819));
#71747=CARTESIAN_POINT('Ctrl Pts',(2.53754933850079,1.68525586471242,4.66723944468617));
#71748=CARTESIAN_POINT('Ctrl Pts',(2.57730466263984,0.140504128071592,5.22502139578419));
#71749=CARTESIAN_POINT('Ctrl Pts',(2.6170599867789,-1.70866126121123,4.93974358553597));
#71750=CARTESIAN_POINT('Ctrl Pts',(2.65681531091796,-3.01348951475503,3.94234604113384));
#71751=CARTESIAN_POINT('Ctrl Pts',(2.69334730323061,-4.21252327337962,3.02581674062289));
#71752=CARTESIAN_POINT('Ctrl Pts',(2.72987929554326,-4.95191040088857,1.50796260801061));
#71753=CARTESIAN_POINT('Ctrl Pts',(2.76641128785591,-4.96079845433821,-0.0023638398085009));
#71754=CARTESIAN_POINT('Origin',(10.45,0.,0.));
#71755=CARTESIAN_POINT('',(3.62178871214421,-4.95694986960482,0.0041615016535472));
#71756=CARTESIAN_POINT('',(3.5164112878559,-4.95527909032578,0.00446627358905836));
#71757=CARTESIAN_POINT('',(10.45,-4.954,-6.06690024297599E-16));
#71758=CARTESIAN_POINT('Ctrl Pts',(3.62178871214421,-4.95694986960482,0.0041615016535472));
#71759=CARTESIAN_POINT('Ctrl Pts',(3.61488250201974,-4.95952078581773,0.290261447214077));
#71760=CARTESIAN_POINT('Ctrl Pts',(3.60797629189526,-4.93689050256876,0.575954920042386));
#71761=CARTESIAN_POINT('Ctrl Pts',(3.60107008177079,-4.88761713886894,0.856976892700365));
#71762=CARTESIAN_POINT('Ctrl Pts',(3.56131475763173,-4.60397697878091,2.47466871091201));
#71763=CARTESIAN_POINT('Ctrl Pts',(3.52155943349267,-3.43746946477165,3.93756179998155));
#71764=CARTESIAN_POINT('Ctrl Pts',(3.48180410935361,-1.92351137346157,4.57420098891072));
#71765=CARTESIAN_POINT('Ctrl Pts',(3.44204878521456,-0.40955328215158,5.21084017783985));
#71766=CARTESIAN_POINT('Ctrl Pts',(3.40229346107551,1.4518553864592,5.0212254666287));
#71767=CARTESIAN_POINT('Ctrl Pts',(3.36253813693645,2.80634428554344,4.09238835422367));
#71768=CARTESIAN_POINT('Ctrl Pts',(3.3227828127974,4.16083318462772,3.16355124181862));
#71769=CARTESIAN_POINT('Ctrl Pts',(3.28302748865834,5.00840231418543,1.49549172821964));
#71770=CARTESIAN_POINT('Ctrl Pts',(3.24327216451929,4.96002483481713,-0.146165415831287));
#71771=CARTESIAN_POINT('Ctrl Pts',(3.20351684038023,4.91164735544884,-1.78782255988222));
#71772=CARTESIAN_POINT('Ctrl Pts',(3.16376151624118,3.96732326715453,-3.40307733438511));
#71773=CARTESIAN_POINT('Ctrl Pts',(3.12400619210212,2.56048909166029,-4.25054188336929));
#71774=CARTESIAN_POINT('Ctrl Pts',(3.08425086796307,1.15365491616609,-5.09800643235344));
#71775=CARTESIAN_POINT('Ctrl Pts',(3.04449554382401,-0.715689346528007,
-5.17768075581891));
#71776=CARTESIAN_POINT('Ctrl Pts',(3.00474021968496,-2.18953098111131,-4.45299503408005));
#71777=CARTESIAN_POINT('Ctrl Pts',(2.9649848955459,-3.66337261569465,-3.72830931234117));
#71778=CARTESIAN_POINT('Ctrl Pts',(2.92522957140685,-4.74171162216717,-2.1992635453979));
#71779=CARTESIAN_POINT('Ctrl Pts',(2.88547424726779,-4.92959980001093,-0.567676406520532));
#71780=CARTESIAN_POINT('Ctrl Pts',(2.8809124022266,-4.9511595978734,-0.380455000081328));
#71781=CARTESIAN_POINT('Ctrl Pts',(2.87635055718541,-4.96099473182037,-0.191883420129216));
#71782=CARTESIAN_POINT('Ctrl Pts',(2.87178871214422,-4.95959242193685,-0.00316426722878071));
#71783=CARTESIAN_POINT('Ctrl Pts',(2.76641128785591,-4.96079845433821,-0.0023638398085009));
#71784=CARTESIAN_POINT('Ctrl Pts',(2.76963461968231,-4.9615826750649,-0.135624661333186));
#71785=CARTESIAN_POINT('Ctrl Pts',(2.77285795150872,-4.95667989894731,-0.268826879197462));
#71786=CARTESIAN_POINT('Ctrl Pts',(2.77608128333513,-4.94590407681699,-0.401552271201664));
#71787=CARTESIAN_POINT('Ctrl Pts',(2.81583660747418,-4.81299926753041,-2.03853576057897));
#71788=CARTESIAN_POINT('Ctrl Pts',(2.85559193161323,-3.78669853115255,-3.60298546077758));
#71789=CARTESIAN_POINT('Ctrl Pts',(2.89534725575229,-2.33806495601783,-4.37683260189643));
#71790=CARTESIAN_POINT('Ctrl Pts',(2.93510257989134,-0.889431380883065,
-5.15067974301529));
#71791=CARTESIAN_POINT('Ctrl Pts',(2.9748579040304,0.981535033008546,-5.13392432505433));
#71792=CARTESIAN_POINT('Ctrl Pts',(3.01461322816945,2.41607701709231,-4.33425693874514));
#71793=CARTESIAN_POINT('Ctrl Pts',(3.05436855230851,3.85061900117604,-3.53458955243598));
#71794=CARTESIAN_POINT('Ctrl Pts',(3.09412387644756,4.84873655545191,-1.95201019777866));
#71795=CARTESIAN_POINT('Ctrl Pts',(3.13387920058661,4.95230242640418,-0.312908997974529));
#71796=CARTESIAN_POINT('Ctrl Pts',(3.17363452472567,5.05586829735645,1.3261922018296));
#71797=CARTESIAN_POINT('Ctrl Pts',(3.21338984886473,4.26488248498501,3.02181524678059));
#71798=CARTESIAN_POINT('Ctrl Pts',(3.25314517300378,2.94240057952509,3.99568394560838));
#71799=CARTESIAN_POINT('Ctrl Pts',(3.29290049714284,1.61991867406513,4.96955264443619));
#71800=CARTESIAN_POINT('Ctrl Pts',(3.33265582128189,-0.234059324483335,
5.22166699714087));
#71801=CARTESIAN_POINT('Ctrl Pts',(3.37241114542095,-1.76857368205384,4.63630871434686));
#71802=CARTESIAN_POINT('Ctrl Pts',(3.41216646956,-3.30308803962434,4.05095043155286));
#71803=CARTESIAN_POINT('Ctrl Pts',(3.45192179369905,-4.51813875621684,2.62811951326019));
#71804=CARTESIAN_POINT('Ctrl Pts',(3.49167711783811,-4.85602814853717,1.02088294343515));
#71805=CARTESIAN_POINT('Ctrl Pts',(3.49992184117737,-4.92610189637556,0.687563541671297));
#71806=CARTESIAN_POINT('Ctrl Pts',(3.50816656451664,-4.95844961896943,0.346312996487832));
#71807=CARTESIAN_POINT('Ctrl Pts',(3.5164112878559,-4.95527909032578,0.00446627358905836));
#71808=CARTESIAN_POINT('Origin',(10.45,0.,0.));
#71809=CARTESIAN_POINT('',(4.37178871214421,-4.94600446667643,0.00102657243331056));
#71810=CARTESIAN_POINT('',(4.26641128785591,-4.9458133698942,0.00011351553366993));
#71811=CARTESIAN_POINT('',(10.45,-4.954,-6.06690024297599E-16));
#71812=CARTESIAN_POINT('Ctrl Pts',(4.37178871214421,-4.94600446667643,0.00102657243331056));
#71813=CARTESIAN_POINT('Ctrl Pts',(4.35341444685407,-4.94741804923094,0.766486964319902));
#71814=CARTESIAN_POINT('Ctrl Pts',(4.33504018156392,-4.78062055825104,1.53136381525057));
#71815=CARTESIAN_POINT('Ctrl Pts',(4.31666591627377,-4.44240910377579,2.21093013129719));
#71816=CARTESIAN_POINT('Ctrl Pts',(4.27691059213471,-3.71064074254432,3.6812680600143));
#71817=CARTESIAN_POINT('Ctrl Pts',(4.23715526799566,-2.17642450967098,4.75223795738543));
#71818=CARTESIAN_POINT('Ctrl Pts',(4.1973999438566,-0.543952277199825,4.93227397970926));
#71819=CARTESIAN_POINT('Ctrl Pts',(4.15764461971755,1.08851995527132,5.11231000203308));
#71820=CARTESIAN_POINT('Ctrl Pts',(4.11788929557849,2.81924818734023,4.40141214930961));
#71821=CARTESIAN_POINT('Ctrl Pts',(4.07813397143944,3.85384325297807,3.12587633668757));
#71822=CARTESIAN_POINT('Ctrl Pts',(4.03837864730038,4.88843831861585,1.8503405240656));
#71823=CARTESIAN_POINT('Ctrl Pts',(3.99862332316133,5.22690021782261,0.0101667515450213));
#71824=CARTESIAN_POINT('Ctrl Pts',(3.95886799902227,4.71387789035592,-1.55002126617717));
#71825=CARTESIAN_POINT('Ctrl Pts',(3.91911267488322,4.20085556288919,-3.11020928389944));
#71826=CARTESIAN_POINT('Ctrl Pts',(3.87935735074416,2.83634900874898,-4.39041154682338));
#71827=CARTESIAN_POINT('Ctrl Pts',(3.83960202660511,1.24665483736224,-4.80302638003053));
#71828=CARTESIAN_POINT('Ctrl Pts',(3.79984670246605,-0.343039334024497,
-5.21564121323768));
#71829=CARTESIAN_POINT('Ctrl Pts',(3.760091378327,-2.1579211226577,-4.76066861672802));
#71830=CARTESIAN_POINT('Ctrl Pts',(3.72033605418794,-3.36497561389084,-3.64693704479633));
#71831=CARTESIAN_POINT('Ctrl Pts',(3.68748694017336,-4.362343173155,-2.7266805463195));
#71832=CARTESIAN_POINT('Ctrl Pts',(3.65463782615879,-4.94472140880247,-1.3566615202199));
#71833=CARTESIAN_POINT('Ctrl Pts',(3.62178871214421,-4.95694986960482,0.0041615016535472));
#71834=CARTESIAN_POINT('Ctrl Pts',(3.5164112878559,-4.95527909032578,0.00446627358905836));
#71835=CARTESIAN_POINT('Ctrl Pts',(3.54792188865569,-4.94316161126636,-1.30204155896344));
#71836=CARTESIAN_POINT('Ctrl Pts',(3.57943248945548,-4.41222884013198,-2.61725776269742));
#71837=CARTESIAN_POINT('Ctrl Pts',(3.61094309025527,-3.48573346682789,-3.53169556471366));
#71838=CARTESIAN_POINT('Ctrl Pts',(3.65069841439433,-2.31682132475008,-4.68539528168019));
#71839=CARTESIAN_POINT('Ctrl Pts',(3.69045373853338,-0.518268972546314,
-5.20115249425582));
#71840=CARTESIAN_POINT('Ctrl Pts',(3.73020906267244,1.0844037440602,-4.84223913943233));
#71841=CARTESIAN_POINT('Ctrl Pts',(3.76996438681149,2.68707646066668,-4.48332578460886));
#71842=CARTESIAN_POINT('Ctrl Pts',(3.80971971095054,4.09386954167586,-3.24974186238633));
#71843=CARTESIAN_POINT('Ctrl Pts',(3.8494750350896,4.65907723057969,-1.70769163582773));
#71844=CARTESIAN_POINT('Ctrl Pts',(3.88923035922865,5.22428491948354,-0.165641409269088));
#71845=CARTESIAN_POINT('Ctrl Pts',(3.92898568336772,4.94790721628189,1.68487512162573));
#71846=CARTESIAN_POINT('Ctrl Pts',(3.96874100750677,3.95679907664445,2.99448700625796));
#71847=CARTESIAN_POINT('Ctrl Pts',(4.00849633164583,2.96569093700703,4.30409889089015));
#71848=CARTESIAN_POINT('Ctrl Pts',(4.04825165578488,1.2598523609339,5.0728061292599));
#71849=CARTESIAN_POINT('Ctrl Pts',(4.08800697992393,-0.377751620602646,
4.94777880232274));
#71850=CARTESIAN_POINT('Ctrl Pts',(4.12776230406299,-2.01535560213924,4.82275147538557));
#71851=CARTESIAN_POINT('Ctrl Pts',(4.16751762820205,-3.58472498913921,3.80398958314144));
#71852=CARTESIAN_POINT('Ctrl Pts',(4.2072729523411,-4.36553291836083,2.35909595020848));
#71853=CARTESIAN_POINT('Ctrl Pts',(4.22698573084604,-4.75269851434006,1.64264177039663));
#71854=CARTESIAN_POINT('Ctrl Pts',(4.24669850935098,-4.9459807075739,0.821414689135449));
#71855=CARTESIAN_POINT('Ctrl Pts',(4.26641128785591,-4.9458133698942,0.00011351553366993));
#71856=CARTESIAN_POINT('Origin',(10.45,0.,0.));
#71857=CARTESIAN_POINT('',(5.12178871214421,-4.95317189454166,-0.0045626926160558));
#71858=CARTESIAN_POINT('',(5.01641128785591,-4.95486112143639,-0.00451032264997429));
#71859=CARTESIAN_POINT('',(10.45,-4.954,-6.06690024297599E-16));
#71860=CARTESIAN_POINT('Ctrl Pts',(5.12178871214421,-4.95317189454166,-0.0045626926160558));
#71861=CARTESIAN_POINT('Ctrl Pts',(5.09194639168839,-4.94190686525697,1.23412115705393));
#71862=CARTESIAN_POINT('Ctrl Pts',(5.06210407123257,-4.47107698524871,2.48044077126415));
#71863=CARTESIAN_POINT('Ctrl Pts',(5.03226175077675,-3.63070508071573,3.38248300921865));
#71864=CARTESIAN_POINT('Ctrl Pts',(4.9925064266377,-2.51117895299637,4.58416508384454));
#71865=CARTESIAN_POINT('Ctrl Pts',(4.95275110249865,-0.73582588621741,5.17485743910726));
#71866=CARTESIAN_POINT('Ctrl Pts',(4.91299577835959,0.880482543602865,4.88343743496305));
#71867=CARTESIAN_POINT('Ctrl Pts',(4.87324045422053,2.49679097342314,4.59201743081884));
#71868=CARTESIAN_POINT('Ctrl Pts',(4.83348513008148,3.95405476628473,3.41848506726771));
#71869=CARTESIAN_POINT('Ctrl Pts',(4.79372980594242,4.58340254905962,1.90148146561086));
#71870=CARTESIAN_POINT('Ctrl Pts',(4.75397448180337,5.2127503318345,0.38447786395402));
#71871=CARTESIAN_POINT('Ctrl Pts',(4.71421915766431,5.01418210452267,-1.47599697580854));
#71872=CARTESIAN_POINT('Ctrl Pts',(4.67446383352526,4.07883895188329,-2.8260013261475));
#71873=CARTESIAN_POINT('Ctrl Pts',(4.63470850938621,3.14349579924394,-4.17600567648642));
#71874=CARTESIAN_POINT('Ctrl Pts',(4.59495318524715,1.47137772127709,-5.0155395374018));
#71875=CARTESIAN_POINT('Ctrl Pts',(4.55519786110809,-0.170027665622429,
-4.95926418773096));
#71876=CARTESIAN_POINT('Ctrl Pts',(4.51544253696904,-1.811433052522,-4.90298883806013));
#71877=CARTESIAN_POINT('Ctrl Pts',(4.47568721282998,-3.42212574835423,-3.95090427780303));
#71878=CARTESIAN_POINT('Ctrl Pts',(4.43593188869093,-4.26281185147555,-2.54000901764294));
#71879=CARTESIAN_POINT('Ctrl Pts',(4.41455082984202,-4.71494648837151,-1.78120663732256));
#71880=CARTESIAN_POINT('Ctrl Pts',(4.39316977099312,-4.94435956325806,-0.889694957216481));
#71881=CARTESIAN_POINT('Ctrl Pts',(4.37178871214421,-4.94600446667643,0.00102657243331056));
#71882=CARTESIAN_POINT('Ctrl Pts',(4.26641128785591,-4.9458133698942,0.00011351553366993));
#71883=CARTESIAN_POINT('Ctrl Pts',(4.28645383349003,-4.94564323288989,-0.834926874492772));
#71884=CARTESIAN_POINT('Ctrl Pts',(4.30649637912414,-4.74549715038149,-1.67004385651608));
#71885=CARTESIAN_POINT('Ctrl Pts',(4.32653892475826,-4.34583113468504,-2.39519584008996));
#71886=CARTESIAN_POINT('Ctrl Pts',(4.36629424889731,-3.55307495034434,-3.83356862383383));
#71887=CARTESIAN_POINT('Ctrl Pts',(4.40604957303637,-1.9753161102196,-4.83928881769982));
#71888=CARTESIAN_POINT('Ctrl Pts',(4.44580489717543,-0.336732163378222,
-4.95073962289765));
#71889=CARTESIAN_POINT('Ctrl Pts',(4.48556022131448,1.3018517834632,-5.06219042809548));
#71890=CARTESIAN_POINT('Ctrl Pts',(4.52531554545354,3.00126083702131,-4.27937184462509));
#71891=CARTESIAN_POINT('Ctrl Pts',(4.5650708695926,3.9814810610906,-2.96159077587687));
#71892=CARTESIAN_POINT('Ctrl Pts',(4.60482619373165,4.96170128515981,-1.64380970712876));
#71893=CARTESIAN_POINT('Ctrl Pts',(4.6445815178707,5.22273267974038,0.208933846896972));
#71894=CARTESIAN_POINT('Ctrl Pts',(4.68433684200975,4.64476411099516,1.74624675140529));
#71895=CARTESIAN_POINT('Ctrl Pts',(4.72409216614881,4.06679554224988,3.28355965591373));
#71896=CARTESIAN_POINT('Ctrl Pts',(4.76384749028786,2.64982701017859,4.50544191090461));
#71897=CARTESIAN_POINT('Ctrl Pts',(4.80360281442692,1.04423471459389,4.85106021653197));
#71898=CARTESIAN_POINT('Ctrl Pts',(4.84335813856597,-0.561357580990757,
5.19667852215931));
#71899=CARTESIAN_POINT('Ctrl Pts',(4.88311346270503,-2.35557364008884,4.66603287842319));
#71900=CARTESIAN_POINT('Ctrl Pts',(4.92286878684409,-3.51488393769876,3.50268500840274));
#71901=CARTESIAN_POINT('Ctrl Pts',(4.95404962051469,-4.42415237771845,2.59024982590285));
#71902=CARTESIAN_POINT('Ctrl Pts',(4.9852304541853,-4.94285510384131,1.28860444610743));
#71903=CARTESIAN_POINT('Ctrl Pts',(5.01641128785591,-4.95486112143639,-0.00451032264997429));
#71904=CARTESIAN_POINT('Origin',(10.45,0.,0.));
#71905=CARTESIAN_POINT('',(5.87178871214421,-4.96183083301335,0.00119183136441884));
#71906=CARTESIAN_POINT('',(5.76641128785591,-4.96104854467068,0.00214542622588053));
#71907=CARTESIAN_POINT('',(10.45,-4.954,-6.06690024297599E-16));
#71908=CARTESIAN_POINT('Ctrl Pts',(5.87178871214421,-4.96183083301335,0.00119183136441884));
#71909=CARTESIAN_POINT('Ctrl Pts',(5.87023366066177,-4.96203861228002,0.0654461038831422));
#71910=CARTESIAN_POINT('Ctrl Pts',(5.86867860917934,-4.9608988621157,0.129692834246658));
#71911=CARTESIAN_POINT('Ctrl Pts',(5.86712355769691,-4.95838874209328,0.193885979561458));
#71912=CARTESIAN_POINT('Ctrl Pts',(5.82736823355785,-4.89421682479881,1.83500161355999));
#71913=CARTESIAN_POINT('Ctrl Pts',(5.7876129094188,-3.93439383172108,3.44109494591861));
#71914=CARTESIAN_POINT('Ctrl Pts',(5.74785758527974,-2.51947014672649,4.27498314272019));
#71915=CARTESIAN_POINT('Ctrl Pts',(5.70810226114069,-1.10454646173199,5.10887133952172));
#71916=CARTESIAN_POINT('Ctrl Pts',(5.66834693700163,0.765477915179317,5.17055440076632));
#71917=CARTESIAN_POINT('Ctrl Pts',(5.62859161286258,2.23227810220183,4.43172033923825));
#71918=CARTESIAN_POINT('Ctrl Pts',(5.58883628872352,3.69907828922439,3.69288627771017));
#71919=CARTESIAN_POINT('Ctrl Pts',(5.54908096458447,4.76265428635814,2.15353509340939));
#71920=CARTESIAN_POINT('Ctrl Pts',(5.50932564044541,4.93483398563358,0.520215556306828));
#71921=CARTESIAN_POINT('Ctrl Pts',(5.46957031630636,5.10701368490903,-1.11310398079573));
#71922=CARTESIAN_POINT('Ctrl Pts',(5.4298149921673,4.38779708632616,-2.84039187070006));
#71923=CARTESIAN_POINT('Ctrl Pts',(5.39005966802825,3.10729833684114,-3.86883803442999));
#71924=CARTESIAN_POINT('Ctrl Pts',(5.35030434388919,1.82679958735616,-4.89728419815988));
#71925=CARTESIAN_POINT('Ctrl Pts',(5.31054901975014,-0.0149813130309392,
-5.22688863571542));
#71926=CARTESIAN_POINT('Ctrl Pts',(5.27079369561108,-1.57268299194724,-4.70636578451226));
#71927=CARTESIAN_POINT('Ctrl Pts',(5.23103837147203,-3.13038467086359,-4.18584293330909));
#71928=CARTESIAN_POINT('Ctrl Pts',(5.19128304733297,-4.40400712830913,-2.81519279334715));
#71929=CARTESIAN_POINT('Ctrl Pts',(5.15152772319392,-4.80896876270199,-1.22353182637166));
#71930=CARTESIAN_POINT('Ctrl Pts',(5.14161471951068,-4.90994608486552,-0.826650619394185));
#71931=CARTESIAN_POINT('Ctrl Pts',(5.13170171582745,-4.95691390505175,-0.416027933139852));
#71932=CARTESIAN_POINT('Ctrl Pts',(5.12178871214421,-4.95317189454166,-0.0045626926160558));
#71933=CARTESIAN_POINT('Ctrl Pts',(5.01641128785591,-4.95486112143639,-0.00451032264997429));
#71934=CARTESIAN_POINT('Ctrl Pts',(5.02498577832435,-4.95816268432983,-0.360106981047611));
#71935=CARTESIAN_POINT('Ctrl Pts',(5.0335602687928,-4.92314744283978,-0.7150585479163));
#71936=CARTESIAN_POINT('Ctrl Pts',(5.04213475926125,-4.84740043695557,-1.06109394842542));
#71937=CARTESIAN_POINT('Ctrl Pts',(5.0818900834003,-4.49620210248069,-2.6654749389285));
#71938=CARTESIAN_POINT('Ctrl Pts',(5.12164540753936,-3.26940089740912,-4.07818682362985));
#71939=CARTESIAN_POINT('Ctrl Pts',(5.16140073167841,-1.73008787677899,-4.65080716674047));
#71940=CARTESIAN_POINT('Ctrl Pts',(5.20115605581747,-0.19077485614891,-5.22342750985107));
#71941=CARTESIAN_POINT('Ctrl Pts',(5.24091137995653,1.66104998003982,-4.95595631137092));
#71942=CARTESIAN_POINT('Ctrl Pts',(5.28066670409558,2.97541518046736,-3.97116051897005));
#71943=CARTESIAN_POINT('Ctrl Pts',(5.32042202823464,4.28978038089491,-2.98636472656919));
#71944=CARTESIAN_POINT('Ctrl Pts',(5.36017735237369,5.06668594556141,-1.28424434024762));
#71945=CARTESIAN_POINT('Ctrl Pts',(5.39993267651274,4.94953899514414,0.353942225694542));
#71946=CARTESIAN_POINT('Ctrl Pts',(5.4396880006518,4.83239204472687,1.99212879163675));
#71947=CARTESIAN_POINT('Ctrl Pts',(5.47944332479086,3.82119257922581,3.56638153719948));
#71948=CARTESIAN_POINT('Ctrl Pts',(5.51919864892991,2.38007233533071,4.35413218014515));
#71949=CARTESIAN_POINT('Ctrl Pts',(5.55895397306896,0.938952091435656,5.1418828230908));
#71950=CARTESIAN_POINT('Ctrl Pts',(5.59870929720802,-0.932088930853352,
5.14313136341939));
#71951=CARTESIAN_POINT('Ctrl Pts',(5.63846462134707,-2.37425921836786,4.35730473200778));
#71952=CARTESIAN_POINT('Ctrl Pts',(5.67821994548612,-3.81642950588238,3.57147810059616));
#71953=CARTESIAN_POINT('Ctrl Pts',(5.71797526962518,-4.82972905862235,1.99857629744435));
#71954=CARTESIAN_POINT('Ctrl Pts',(5.75773059376423,-4.94906221816879,0.360547534003953));
#71955=CARTESIAN_POINT('Ctrl Pts',(5.76062415846146,-4.95774780243076,0.241324705223826));
#71956=CARTESIAN_POINT('Ctrl Pts',(5.76351772315868,-4.96169754703925,0.121756862533341));
#71957=CARTESIAN_POINT('Ctrl Pts',(5.76641128785591,-4.96104854467068,0.00214542622588053));
#71958=CARTESIAN_POINT('Origin',(10.45,0.,0.));
#71959=CARTESIAN_POINT('',(6.6217887121442,-4.94958263022186,0.00393761749848148));
#71960=CARTESIAN_POINT('',(6.5164112878559,-4.94831334867398,0.00338484824665104));
#71961=CARTESIAN_POINT('',(10.45,-4.954,-6.06690024297599E-16));
#71962=CARTESIAN_POINT('Ctrl Pts',(6.6217887121442,-4.94958263022186,0.00393761749848148));
#71963=CARTESIAN_POINT('Ctrl Pts',(6.6087656054961,-4.95359906417513,0.545489558835211));
#71964=CARTESIAN_POINT('Ctrl Pts',(6.595742498848,-4.87171144893763,1.08586043165447));
#71965=CARTESIAN_POINT('Ctrl Pts',(6.58271939219989,-4.69874473428602,1.59530831277444));
#71966=CARTESIAN_POINT('Ctrl Pts',(6.54296406806084,-4.17073340856723,3.15048759473392));
#71967=CARTESIAN_POINT('Ctrl Pts',(6.50320874392178,-2.7939714110088,4.4175007645021));
#71968=CARTESIAN_POINT('Ctrl Pts',(6.46345341978272,-1.20038049269541,4.81479982590597));
#71969=CARTESIAN_POINT('Ctrl Pts',(6.42369809564367,0.393210425618072,5.21209888730986));
#71970=CARTESIAN_POINT('Ctrl Pts',(6.38394277150462,2.20363026468645,4.73968384034942));
#71971=CARTESIAN_POINT('Ctrl Pts',(6.34418744736557,3.39991210580398,3.61438907197266));
#71972=CARTESIAN_POINT('Ctrl Pts',(6.30443212322651,4.59619394692144,2.48909430359597));
#71973=CARTESIAN_POINT('Ctrl Pts',(6.26467679908746,5.17833779008799,0.710919813803045));
#71974=CARTESIAN_POINT('Ctrl Pts',(6.2249214749484,4.87914468776635,-0.903967812828126));
#71975=CARTESIAN_POINT('Ctrl Pts',(6.18516615080935,4.5799515854447,-2.51885543945934));
#71976=CARTESIAN_POINT('Ctrl Pts',(6.14541082667029,3.39942153763477,-3.97045620292885));
#71977=CARTESIAN_POINT('Ctrl Pts',(6.10565550253123,1.87940754169061,-4.59249801121615));
#71978=CARTESIAN_POINT('Ctrl Pts',(6.06590017839218,0.3593935457465,-5.21453981950343));
#71979=CARTESIAN_POINT('Ctrl Pts',(6.02614485425313,-1.50010439833188,-5.00702267260859));
#71980=CARTESIAN_POINT('Ctrl Pts',(5.98638953011408,-2.84559294961542,-4.06519513134202));
#71981=CARTESIAN_POINT('Ctrl Pts',(5.94818925745746,-4.13845197236205,-3.16020769504152));
#71982=CARTESIAN_POINT('Ctrl Pts',(5.90998898480083,-4.95672667747323,-1.57723226410399));
#71983=CARTESIAN_POINT('Ctrl Pts',(5.87178871214421,-4.96183083301335,0.00119183136441884));
#71984=CARTESIAN_POINT('Ctrl Pts',(5.76641128785591,-4.96104854467068,0.00214542622588053));
#71985=CARTESIAN_POINT('Ctrl Pts',(5.80327304729774,-4.95278076022806,-1.52161106551157));
#71986=CARTESIAN_POINT('Ctrl Pts',(5.84013480673957,-4.19819269721077,-3.05244226706159));
#71987=CARTESIAN_POINT('Ctrl Pts',(5.8769965661814,-2.98071241642748,-3.96718601204142));
#71988=CARTESIAN_POINT('Ctrl Pts',(5.91675189032046,-1.66766268878702,-4.95373507091722));
#71989=CARTESIAN_POINT('Ctrl Pts',(5.95650721445951,0.183803532846682,-5.22367746493987));
#71990=CARTESIAN_POINT('Ctrl Pts',(5.99626253859856,1.72387939810757,-4.65311198923499));
#71991=CARTESIAN_POINT('Ctrl Pts',(6.03601786273762,3.26395526336846,-4.08254651353011));
#71992=CARTESIAN_POINT('Ctrl Pts',(6.07577318687667,4.4926407722565,-2.67147316809771));
#71993=CARTESIAN_POINT('Ctrl Pts',(6.11552851101573,4.84597999071355,-1.06756231349089));
#71994=CARTESIAN_POINT('Ctrl Pts',(6.15528383515478,5.19931920917062,0.536348541116021));
#71995=CARTESIAN_POINT('Ctrl Pts',(6.19503915929383,4.67731213719657,2.33309690489733));
#71996=CARTESIAN_POINT('Ctrl Pts',(6.23479448343289,3.51955546876279,3.49799094708435));
#71997=CARTESIAN_POINT('Ctrl Pts',(6.27454980757194,2.36179880032908,4.66288498927131));
#71998=CARTESIAN_POINT('Ctrl Pts',(6.314305131711,0.568292535435575,5.19592470986405));
#71999=CARTESIAN_POINT('Ctrl Pts',(6.35406045585006,-1.03775959026624,4.8524495253833));
#72000=CARTESIAN_POINT('Ctrl Pts',(6.39381577998912,-2.64381171596806,4.50897434090254));
#72001=CARTESIAN_POINT('Ctrl Pts',(6.43357110412817,-4.0624097024783,3.28898425134839));
#72002=CARTESIAN_POINT('Ctrl Pts',(6.47332642826722,-4.64242944460635,1.7524440691315));
#72003=CARTESIAN_POINT('Ctrl Pts',(6.48768804813011,-4.85196170801539,1.19736857977379));
#72004=CARTESIAN_POINT('Ctrl Pts',(6.502049667993,-4.9520580628245,0.6009827568366));
#72005=CARTESIAN_POINT('Ctrl Pts',(6.5164112878559,-4.94831334867398,0.00338484824665104));
#72006=CARTESIAN_POINT('Origin',(10.45,0.,0.));
#72007=CARTESIAN_POINT('',(7.3717887121442,-4.94758462196668,-0.0029330133969574));
#72008=CARTESIAN_POINT('',(7.2664112878559,-4.94870345086251,-0.00358126079844738));
#72009=CARTESIAN_POINT('',(10.45,-4.954,-6.06690024297599E-16));
#72010=CARTESIAN_POINT('Ctrl Pts',(7.3717887121442,-4.94758462196668,-0.0029330133969574));
#72011=CARTESIAN_POINT('Ctrl Pts',(7.34729755033043,-4.94210089569579,1.01653919561904));
#72012=CARTESIAN_POINT('Ctrl Pts',(7.32280638851666,-4.63564882247797,2.03903518839942));
#72013=CARTESIAN_POINT('Ctrl Pts',(7.29831522670288,-4.05145720843067,2.86511870243504));
#72014=CARTESIAN_POINT('Ctrl Pts',(7.25855990256383,-3.10316708024632,4.20606030888607));
#72015=CARTESIAN_POINT('Ctrl Pts',(7.21880457842477,-1.42304808668591,5.02946551761624));
#72016=CARTESIAN_POINT('Ctrl Pts',(7.17904925428572,0.217739805369029,4.95739851816915));
#72017=CARTESIAN_POINT('Ctrl Pts',(7.13929393014666,1.85852769742402,4.88533151872206));
#72018=CARTESIAN_POINT('Ctrl Pts',(7.09953860600761,3.45998448797345,3.91779231109747));
#72019=CARTESIAN_POINT('Ctrl Pts',(7.05978328186855,4.28705547535841,2.49887295435108));
#72020=CARTESIAN_POINT('Ctrl Pts',(7.0200279577295,5.11412646274337,1.07995359760469));
#72021=CARTESIAN_POINT('Ctrl Pts',(6.98027263359043,5.16681164696395,-0.790345908263659));
#72022=CARTESIAN_POINT('Ctrl Pts',(6.94051730945138,4.42092898789413,-2.25357439965606));
#72023=CARTESIAN_POINT('Ctrl Pts',(6.90076198531233,3.67504632882437,-3.71680289104838));
#72024=CARTESIAN_POINT('Ctrl Pts',(6.86100666117328,2.13059582646437,-4.7729603679649));
#72025=CARTESIAN_POINT('Ctrl Pts',(6.82125133703422,0.4964667933065,-4.9372797585241));
#72026=CARTESIAN_POINT('Ctrl Pts',(6.78149601289517,-1.13766223985146,-5.10159914908331));
#72027=CARTESIAN_POINT('Ctrl Pts',(6.74174068875611,-2.86146980380727,-4.37408045328508));
#72028=CARTESIAN_POINT('Ctrl Pts',(6.70198536461705,-3.88374325884562,-3.08864840831052));
#72029=CARTESIAN_POINT('Ctrl Pts',(6.6752531471261,-4.57113889520683,-2.22430005396414));
#72030=CARTESIAN_POINT('Ctrl Pts',(6.64852092963515,-4.94133819293988,-1.10769301485678));
#72031=CARTESIAN_POINT('Ctrl Pts',(6.6217887121442,-4.94958263022186,0.00393761749848148));
#72032=CARTESIAN_POINT('Ctrl Pts',(6.5164112878559,-4.94831334867398,0.00338484824665104));
#72033=CARTESIAN_POINT('Ctrl Pts',(6.54180499213206,-4.94169207860521,-1.05326647045278));
#72034=CARTESIAN_POINT('Ctrl Pts',(6.56719869640822,-4.6104215531534,-2.11370726000965));
#72035=CARTESIAN_POINT('Ctrl Pts',(6.59259240068438,-3.98543003566754,-2.95627447886375));
#72036=CARTESIAN_POINT('Ctrl Pts',(6.63234772482344,-3.00696938685488,-4.27536256976238));
#72037=CARTESIAN_POINT('Ctrl Pts',(6.6721030489625,-1.30860659148386,-5.06044847667997));
#72038=CARTESIAN_POINT('Ctrl Pts',(6.71185837310155,0.330124637624449,-4.95118461453574));
#72039=CARTESIAN_POINT('Ctrl Pts',(6.75161369724061,1.96885586673271,-4.84192075239152));
#72040=CARTESIAN_POINT('Ctrl Pts',(6.79136902137966,3.5479555295782,-3.83830712118545));
#72041=CARTESIAN_POINT('Ctrl Pts',(6.83112434551871,4.34263065115712,-2.40099362581679));
#72042=CARTESIAN_POINT('Ctrl Pts',(6.87087966965777,5.13730577273608,-0.963680130448044));
#72043=CARTESIAN_POINT('Ctrl Pts',(6.91063499379683,5.14755635304839,0.907333229083402));
#72044=CARTESIAN_POINT('Ctrl Pts',(6.95039031793589,4.36867746511897,2.35326763657341));
#72045=CARTESIAN_POINT('Ctrl Pts',(6.99014564207494,3.58979857718957,3.79920204406338));
#72046=CARTESIAN_POINT('Ctrl Pts',(7.02990096621399,2.02179022101859,4.82005749951193));
#72047=CARTESIAN_POINT('Ctrl Pts',(7.06965629035304,0.384354558565735,4.94727025104672));
#72048=CARTESIAN_POINT('Ctrl Pts',(7.1094116144921,-1.25308110388707,5.0744830025815));
#72049=CARTESIAN_POINT('Ctrl Pts',(7.14916693863116,-2.95994407262174,4.30805305020248));
#72050=CARTESIAN_POINT('Ctrl Pts',(7.18892226277021,-3.95279912936723,2.99976505854306));
#72051=CARTESIAN_POINT('Ctrl Pts',(7.21475193779878,-4.59787306654607,2.14974925814021));
#72052=CARTESIAN_POINT('Ctrl Pts',(7.24058161282734,-4.94154210184746,1.07099836052273));
#72053=CARTESIAN_POINT('Ctrl Pts',(7.2664112878559,-4.94870345086251,-0.00358126079844738));
#72054=CARTESIAN_POINT('Origin',(10.45,0.,0.));
#72055=CARTESIAN_POINT('',(8.1217887121442,-4.96031738439419,-0.00272426264678605));
#72056=CARTESIAN_POINT('',(8.01641128785589,-4.96134628578967,-0.00184569647040522));
#72057=CARTESIAN_POINT('',(10.45,-4.954,-6.06690024297599E-16));
#72058=CARTESIAN_POINT('Ctrl Pts',(8.1217887121442,-4.96031738439419,-0.00272426264678605));
#72059=CARTESIAN_POINT('Ctrl Pts',(8.08582949516476,-4.95049138164272,1.48430270424084));
#72060=CARTESIAN_POINT('Ctrl Pts',(8.04987027818531,-4.23705260128488,2.97950340891386));
#72061=CARTESIAN_POINT('Ctrl Pts',(8.01391106120587,-3.06992698280977,3.89855858119438));
#72062=CARTESIAN_POINT('Ctrl Pts',(7.97415573706681,-1.77959139791648,4.91463566364519));
#72063=CARTESIAN_POINT('Ctrl Pts',(7.93440041292776,0.0652758196799033,
5.22650249375973));
#72064=CARTESIAN_POINT('Ctrl Pts',(7.8946450887887,1.61789670492097,4.69101491609158));
#72065=CARTESIAN_POINT('Ctrl Pts',(7.85488976464965,3.17051759016195,4.15552733842346));
#72066=CARTESIAN_POINT('Ctrl Pts',(7.8151344405106,4.43089214304765,2.77268535297278));
#72067=CARTESIAN_POINT('Ctrl Pts',(7.77537911637154,4.82051943466333,1.17720137224732));
#72068=CARTESIAN_POINT('Ctrl Pts',(7.73562379223248,5.21014672627902,-0.418282608478192));
#72069=CARTESIAN_POINT('Ctrl Pts',(7.69586846809343,4.72902675662464,-2.22640858447849));
#72070=CARTESIAN_POINT('Ctrl Pts',(7.65611314395437,3.59798939625515,-3.41726250019271));
#72071=CARTESIAN_POINT('Ctrl Pts',(7.61635781981532,2.46695203588565,-4.60811641590694));
#72072=CARTESIAN_POINT('Ctrl Pts',(7.57660249567626,0.685997284801031,-5.18169827133508));
#72073=CARTESIAN_POINT('Ctrl Pts',(7.53684717153721,-0.927432156732568,
-4.87473899664856));
#72074=CARTESIAN_POINT('Ctrl Pts',(7.49709184739816,-2.54086159826608,-4.56777972196205));
#72075=CARTESIAN_POINT('Ctrl Pts',(7.4573365232591,-3.98676573024859,-3.380279317161));
#72076=CARTESIAN_POINT('Ctrl Pts',(7.41758119912005,-4.60148716483585,-1.85729011267458));
#72077=CARTESIAN_POINT('Ctrl Pts',(7.40231703679476,-4.83751109283982,-1.27253436132866));
#72078=CARTESIAN_POINT('Ctrl Pts',(7.38705287446948,-4.95100236460309,-0.63832097101446));
#72079=CARTESIAN_POINT('Ctrl Pts',(7.3717887121442,-4.94758462196668,-0.0029330133969574));
#72080=CARTESIAN_POINT('Ctrl Pts',(7.2664112878559,-4.94870345086251,-0.00358126079844738));
#72081=CARTESIAN_POINT('Ctrl Pts',(7.28033693696639,-4.95256437568759,-0.58292338303811));
#72082=CARTESIAN_POINT('Ctrl Pts',(7.29426258607689,-4.85861423275224,-1.16105306049541));
#72083=CARTESIAN_POINT('Ctrl Pts',(7.30818823518738,-4.6613521558272,-1.70147213992685));
#72084=CARTESIAN_POINT('Ctrl Pts',(7.34794355932643,-4.09820298078534,-3.24427531579696));
#72085=CARTESIAN_POINT('Ctrl Pts',(7.38769888346549,-2.69305748594547,-4.47973563659737));
#72086=CARTESIAN_POINT('Ctrl Pts',(7.42745420760454,-1.0908652001314,-4.84078758868063));
#72087=CARTESIAN_POINT('Ctrl Pts',(7.4672095317436,0.511327085682714,-5.20183954076389));
#72088=CARTESIAN_POINT('Ctrl Pts',(7.50696485588265,2.31056616247103,-4.68848312412996));
#72089=CARTESIAN_POINT('Ctrl Pts',(7.54672018002171,3.48101698391448,-3.53634445738549));
#72090=CARTESIAN_POINT('Ctrl Pts',(7.58647550416076,4.65146780535801,-2.38420579064096));
#72091=CARTESIAN_POINT('Ctrl Pts',(7.62623082829981,5.19313037145658,-0.593284873785803));
#72092=CARTESIAN_POINT('Ctrl Pts',(7.66598615243887,4.85738628783773,1.01440120973319));
#72093=CARTESIAN_POINT('Ctrl Pts',(7.70574147657793,4.52164220421889,2.62208729325209));
#72094=CARTESIAN_POINT('Ctrl Pts',(7.74549680071698,3.30849147088272,4.04653854343484));
#72095=CARTESIAN_POINT('Ctrl Pts',(7.78525212485604,1.77475969537718,4.63394425810743));
#72096=CARTESIAN_POINT('Ctrl Pts',(7.82500744899509,0.241027919871597,5.22134997278003));
#72097=CARTESIAN_POINT('Ctrl Pts',(7.86476277313414,-1.61328489780338,4.97171015194241));
#72098=CARTESIAN_POINT('Ctrl Pts',(7.9045180972732,-2.93706534452188,3.99960729642182));
#72099=CARTESIAN_POINT('Ctrl Pts',(7.94181582746743,-4.17901235432128,3.08759787852779));
#72100=CARTESIAN_POINT('Ctrl Pts',(7.97911355766166,-4.95399246532965,1.53968697513372));
#72101=CARTESIAN_POINT('Ctrl Pts',(8.01641128785589,-4.96134628578967,-0.00184569647040522));
#72102=CARTESIAN_POINT('Origin',(10.45,0.,0.));
#72103=CARTESIAN_POINT('',(8.87178871214419,-4.95600107193163,0.00436047568620729));
#72104=CARTESIAN_POINT('',(8.76641128785588,-4.95430821334551,0.00454960891578283));
#72105=CARTESIAN_POINT('',(10.45,-4.954,-6.06690024297599E-16));
#72106=CARTESIAN_POINT('Ctrl Pts',(8.87178871214419,-4.95600107193163,0.00436047568620729));
#72107=CARTESIAN_POINT('Ctrl Pts',(8.86411676413813,-4.95892682062427,0.32233931392055));
#72108=CARTESIAN_POINT('Ctrl Pts',(8.85644481613207,-4.93095453643991,0.639805423207782));
#72109=CARTESIAN_POINT('Ctrl Pts',(8.84877286812601,-4.87022046359406,0.950875032155887));
#72110=CARTESIAN_POINT('Ctrl Pts',(8.80901754398696,-4.55550212212915,2.56280894043786));
#72111=CARTESIAN_POINT('Ctrl Pts',(8.76926221984791,-3.36105884895625,4.00298297070627));
#72112=CARTESIAN_POINT('Ctrl Pts',(8.72950689570886,-1.83512969054333,4.61036980183522));
#72113=CARTESIAN_POINT('Ctrl Pts',(8.6897515715698,-0.309200532130504,5.21775663296414));
#72114=CARTESIAN_POINT('Ctrl Pts',(8.64999624743074,1.54821451152233,4.99235626495374));
#72115=CARTESIAN_POINT('Ctrl Pts',(8.61024092329168,2.88457813261785,4.03762550115916));
#72116=CARTESIAN_POINT('Ctrl Pts',(8.57048559915263,4.22094175371341,3.08289473736455));
#72117=CARTESIAN_POINT('Ctrl Pts',(8.53073027501358,5.03625395225163,1.39883357778585));
#72118=CARTESIAN_POINT('Ctrl Pts',(8.49097495087453,4.95629353888058,-0.241588590869826));
#72119=CARTESIAN_POINT('Ctrl Pts',(8.45121962673548,4.87633312550953,-1.88201075952545));
#72120=CARTESIAN_POINT('Ctrl Pts',(8.41146430259642,3.90110010022918,-3.47879393725799));
#72121=CARTESIAN_POINT('Ctrl Pts',(8.37170897845736,2.47821791730663,-4.29902856993627));
#72122=CARTESIAN_POINT('Ctrl Pts',(8.33195365431831,1.05533573438403,-5.11926320261456));
#72123=CARTESIAN_POINT('Ctrl Pts',(8.29219833017925,-0.815195606180847,
-5.16294929023855));
#72124=CARTESIAN_POINT('Ctrl Pts',(8.2524430060402,-2.27481853068622,-4.41003529954517));
#72125=CARTESIAN_POINT('Ctrl Pts',(8.21268768190114,-3.7344414551916,-3.65712130885178));
#72126=CARTESIAN_POINT('Ctrl Pts',(8.17293235776209,-4.78315596363752,-2.10760723984099));
#72127=CARTESIAN_POINT('Ctrl Pts',(8.13317703362303,-4.93961124176535,-0.472706537942125));
#72128=CARTESIAN_POINT('Ctrl Pts',(8.12938092646342,-4.95455064961378,-0.316595164330307));
#72129=CARTESIAN_POINT('Ctrl Pts',(8.12558481930381,-4.96135468616349,-0.159705259167466));
#72130=CARTESIAN_POINT('Ctrl Pts',(8.1217887121442,-4.96031738439419,-0.00272426264678605));
#72131=CARTESIAN_POINT('Ctrl Pts',(8.01641128785589,-4.96134628578967,-0.00184569647040522));
#72132=CARTESIAN_POINT('Ctrl Pts',(8.01886888180072,-4.96183083818843,-0.103419206165346));
#72133=CARTESIAN_POINT('Ctrl Pts',(8.02132647574554,-4.95898262098761,-0.204965023769395));
#72134=CARTESIAN_POINT('Ctrl Pts',(8.02378406969036,-4.95271562240422,-0.306299407729264));
#72135=CARTESIAN_POINT('Ctrl Pts',(8.06353939382942,-4.85133737780601,-1.9455373661562));
#72136=CARTESIAN_POINT('Ctrl Pts',(8.10329471796847,-3.85533281284763,-3.52944739280642));
#72137=CARTESIAN_POINT('Ctrl Pts',(8.14305004210753,-2.42185933737396,-4.33102859763783));
#72138=CARTESIAN_POINT('Ctrl Pts',(8.18280536624658,-0.988385861900328,
-5.13260980246921));
#72139=CARTESIAN_POINT('Ctrl Pts',(8.22256069038564,0.882556524088673,-5.15186218548167));
#72140=CARTESIAN_POINT('Ctrl Pts',(8.26231601452469,2.33222158062585,-4.37994907075929));
#72141=CARTESIAN_POINT('Ctrl Pts',(8.30207133866375,3.78188663716307,-3.60803595603689));
#72142=CARTESIAN_POINT('Ctrl Pts',(8.3418266628028,4.81027436424862,-2.04495734357959));
#72143=CARTESIAN_POINT('Ctrl Pts',(8.38158198694186,4.94536376301241,-0.408152685971623));
#72144=CARTESIAN_POINT('Ctrl Pts',(8.42133731108091,5.0804531617762,1.22865197163634));
#72145=CARTESIAN_POINT('Ctrl Pts',(8.46109263521996,4.3222442322183,2.93918267439492));
#72146=CARTESIAN_POINT('Ctrl Pts',(8.50084795935901,3.01874826118703,3.93832074610009));
#72147=CARTESIAN_POINT('Ctrl Pts',(8.54060328349807,1.71525229015575,4.93745881780527));
#72148=CARTESIAN_POINT('Ctrl Pts',(8.58035860763713,-0.133530722348902,
5.22520425845695));
#72149=CARTESIAN_POINT('Ctrl Pts',(8.62011393177619,-1.67902549555258,4.66948442002611));
#72150=CARTESIAN_POINT('Ctrl Pts',(8.65986925591524,-3.22452026875627,4.11376458159526));
#72151=CARTESIAN_POINT('Ctrl Pts',(8.69962458005429,-4.46672680265902,2.71457946408189));
#72152=CARTESIAN_POINT('Ctrl Pts',(8.73937990419334,-4.83548313062843,1.1141428350934));
#72153=CARTESIAN_POINT('Ctrl Pts',(8.74839036541419,-4.91906098252792,0.751407214287453));
#72154=CARTESIAN_POINT('Ctrl Pts',(8.75740082663503,-4.95777032957647,0.378333449008531));
#72155=CARTESIAN_POINT('Ctrl Pts',(8.76641128785588,-4.95430821334551,0.00454960891578283));
#72156=CARTESIAN_POINT('Origin',(10.45,0.,0.));
#72157=CARTESIAN_POINT('',(9.62178871214419,-4.94585766451186,0.000506886091347358));
#72158=CARTESIAN_POINT('',(9.51641128785588,-4.94584202552434,-0.00041315751885764));
#72159=CARTESIAN_POINT('',(10.45,-4.954,-6.06690024297599E-16));
#72160=CARTESIAN_POINT('Ctrl Pts',(9.62178871214419,-4.94585766451186,0.000506886091347358));
#72161=CARTESIAN_POINT('Ctrl Pts',(9.60264870897246,-4.94658353356567,0.797926455850933));
#72162=CARTESIAN_POINT('Ctrl Pts',(9.58350870580073,-4.76490303293466,1.59503395194384));
#72163=CARTESIAN_POINT('Ctrl Pts',(9.564368702629,-4.39903952636143,2.29601000352735));
#72164=CARTESIAN_POINT('Ctrl Pts',(9.52461337848995,-3.63911163272578,3.75199357335154));
#72165=CARTESIAN_POINT('Ctrl Pts',(9.4848580543509,-2.08456986568594,4.7932408373652));
#72166=CARTESIAN_POINT('Ctrl Pts',(9.44510273021185,-0.448935340223443,
4.94182838138743));
#72167=CARTESIAN_POINT('Ctrl Pts',(9.40534740607279,1.18669918523901,5.09041592540966));
#72168=CARTESIAN_POINT('Ctrl Pts',(9.36559208193373,2.90342646912413,4.34634374944051));
#72169=CARTESIAN_POINT('Ctrl Pts',(9.32583675779467,3.9132836585268,3.05113449370803));
#72170=CARTESIAN_POINT('Ctrl Pts',(9.28608143365562,4.9231408479295,1.75592523797551));
#72171=CARTESIAN_POINT('Ctrl Pts',(9.24632610951657,5.22612794284971,-0.090421097520369));
#72172=CARTESIAN_POINT('Ctrl Pts',(9.20657078537752,4.68317650886116,-1.64044764550375));
#72173=CARTESIAN_POINT('Ctrl Pts',(9.16681546123846,4.14022507487263,-3.19047419348709));
#72174=CARTESIAN_POINT('Ctrl Pts',(9.1270601370994,2.7513351119754,-4.44418095395794));
#72175=CARTESIAN_POINT('Ctrl Pts',(9.08730481296035,1.15399500158496,-4.82612745657476));
#72176=CARTESIAN_POINT('Ctrl Pts',(9.04754948882129,-0.443345108805517,
-5.20807395919159));
#72177=CARTESIAN_POINT('Ctrl Pts',(9.00779416468224,-2.24913536668921,-4.71826020395433));
#72178=CARTESIAN_POINT('Ctrl Pts',(8.96803884054319,-3.43453379075257,-3.58150643318794));
#72179=CARTESIAN_POINT('Ctrl Pts',(8.93595546441019,-4.39117505403748,-2.66412242015528));
#72180=CARTESIAN_POINT('Ctrl Pts',(8.90387208827719,-4.94376586182561,-1.32539758072267));
#72181=CARTESIAN_POINT('Ctrl Pts',(8.87178871214419,-4.95600107193163,0.00436047568620729));
#72182=CARTESIAN_POINT('Ctrl Pts',(8.76641128785588,-4.95430821334551,0.00454960891578283));
#72183=CARTESIAN_POINT('Ctrl Pts',(8.79715615077409,-4.94249502350775,-1.2708493571334));
#72184=CARTESIAN_POINT('Ctrl Pts',(8.8279010136923,-4.43969511014743,-2.55451546117548));
#72185=CARTESIAN_POINT('Ctrl Pts',(8.85864587661051,-3.55305158563404,-3.4639624411078));
#72186=CARTESIAN_POINT('Ctrl Pts',(8.89840120074957,-2.40655759063403,-4.63994294785716));
#72187=CARTESIAN_POINT('Ctrl Pts',(8.93815652488862,-0.618263478597702,
-5.19021582089223));
#72188=CARTESIAN_POINT('Ctrl Pts',(8.97791184902767,0.991019347533268,-4.86221061004117));
#72189=CARTESIAN_POINT('Ctrl Pts',(9.01766717316673,2.60030217366424,-4.53420539919011));
#72190=CARTESIAN_POINT('Ctrl Pts',(9.05742249730579,4.03057371388998,-3.32792210445298));
#72191=CARTESIAN_POINT('Ctrl Pts',(9.09717782144485,4.62535180366144,-1.79703423894704));
#72192=CARTESIAN_POINT('Ctrl Pts',(9.1369331455839,5.22012989343289,-0.266146373441135));
#72193=CARTESIAN_POINT('Ctrl Pts',(9.17668846972296,4.9794145327501,1.58934606283357));
#72194=CARTESIAN_POINT('Ctrl Pts',(9.21644379386201,4.01369197305335,2.91778822210064));
#72195=CARTESIAN_POINT('Ctrl Pts',(9.25619911800106,3.04796941335657,4.24623038136774));
#72196=CARTESIAN_POINT('Ctrl Pts',(9.29595444214012,1.35723965464579,5.04762226362717));
#72197=CARTESIAN_POINT('Ctrl Pts',(9.33570976627917,-0.282467087522345,
4.95413198330936));
#72198=CARTESIAN_POINT('Ctrl Pts',(9.37546509041823,-1.92217382969048,4.86064170299156));
#72199=CARTESIAN_POINT('Ctrl Pts',(9.41522041455728,-3.51085755531596,3.87226926009653));
#72200=CARTESIAN_POINT('Ctrl Pts',(9.45497573869634,-4.31932628815499,2.44266898699667));
#72201=CARTESIAN_POINT('Ctrl Pts',(9.47545425508285,-4.73577969538968,1.70626214708662));
#72202=CARTESIAN_POINT('Ctrl Pts',(9.49593277146937,-4.94520911289263,0.852778928698556));
#72203=CARTESIAN_POINT('Ctrl Pts',(9.51641128785588,-4.94584202552434,-0.00041315751885764));
#72204=CARTESIAN_POINT('Origin',(10.45,0.,0.));
#72205=CARTESIAN_POINT('',(10.3717887121442,-4.95413490991508,-0.00455749466325095));
#72206=CARTESIAN_POINT('',(10.2664112878559,-4.95582936423354,-0.0043891145566411));
#72207=CARTESIAN_POINT('',(10.45,-4.954,-6.06690024297599E-16));
#72208=CARTESIAN_POINT('Ctrl Pts',(10.3717887121442,-4.95413490991508,-0.00455749466325095));
#72209=CARTESIAN_POINT('Ctrl Pts',(10.3411806538068,-4.94239235035036,1.26527993119002));
#72210=CARTESIAN_POINT('Ctrl Pts',(10.3105725954694,-4.44452057764309,2.54329575077959));
#72211=CARTESIAN_POINT('Ctrl Pts',(10.279964537132,-3.56494056432348,3.45172557768268));
#72212=CARTESIAN_POINT('Ctrl Pts',(10.2402092129929,-2.42249669708122,4.63164107013291));
#72213=CARTESIAN_POINT('Ctrl Pts',(10.2004538888539,-0.636105165059572,
5.18805931624687));
#72214=CARTESIAN_POINT('Ctrl Pts',(10.1606985647148,0.974295896435707,4.86558919319915));
#72215=CARTESIAN_POINT('Ctrl Pts',(10.1209432405758,2.58469695793099,4.54311907015144));
#72216=CARTESIAN_POINT('Ctrl Pts',(10.0811879164367,4.01910754889984,3.34176057794207));
#72217=CARTESIAN_POINT('Ctrl Pts',(10.0414325922977,4.61914571659599,1.81292678827382));
#72218=CARTESIAN_POINT('Ctrl Pts',(10.0016772681586,5.2191838842921,0.28409299860565));
#72219=CARTESIAN_POINT('Ctrl Pts',(9.96192194401955,4.98484962871553,-1.57221608852144));
#72220=CARTESIAN_POINT('Ctrl Pts',(9.9221666198805,4.02370032970805,-2.90397078971107));
#72221=CARTESIAN_POINT('Ctrl Pts',(9.88241129574144,3.06255103070049,-4.23572549090081));
#72222=CARTESIAN_POINT('Ctrl Pts',(9.84265597160239,1.37458668826192,-5.04292580615308));
#72223=CARTESIAN_POINT('Ctrl Pts',(9.80290064746333,-0.265431784004649,
-4.95507382980597));
#72224=CARTESIAN_POINT('Ctrl Pts',(9.76314532332428,-1.90545025627113,-4.86722185345886));
#72225=CARTESIAN_POINT('Ctrl Pts',(9.72338999918523,-3.49752285836557,-3.88431758551248));
#72226=CARTESIAN_POINT('Ctrl Pts',(9.68363467504617,-4.31090214929706,-2.45750551372196));
#72227=CARTESIAN_POINT('Ctrl Pts',(9.66301935407884,-4.73268402414932,-1.71762502080647));
#72228=CARTESIAN_POINT('Ctrl Pts',(9.64240403311151,-4.94507584523051,-0.858378048708709));
#72229=CARTESIAN_POINT('Ctrl Pts',(9.62178871214419,-4.94585766451186,0.000506886091347358));
#72230=CARTESIAN_POINT('Ctrl Pts',(9.51641128785588,-4.94584202552434,-0.00041315751885764));
#72231=CARTESIAN_POINT('Ctrl Pts',(9.53568809560842,-4.94643779793751,-0.803538711713373));
#72232=CARTESIAN_POINT('Ctrl Pts',(9.55496490336096,-4.76202302770542,-1.60640629932515));
#72233=CARTESIAN_POINT('Ctrl Pts',(9.57424171111351,-4.39111928801005,-2.31112153770593));
#72234=CARTESIAN_POINT('Ctrl Pts',(9.61399703525256,-3.62618981497348,-3.76448368600399));
#72235=CARTESIAN_POINT('Ctrl Pts',(9.65375235939162,-2.06807712884795,-4.80037987929536));
#72236=CARTESIAN_POINT('Ctrl Pts',(9.69350768353067,-0.43194136533549,-4.94334279819782));
#72237=CARTESIAN_POINT('Ctrl Pts',(9.73326300766973,1.20419439817692,-5.08630571710027));
#72238=CARTESIAN_POINT('Ctrl Pts',(9.77301833180877,2.91835323907617,-4.33633536161367));
#72239=CARTESIAN_POINT('Ctrl Pts',(9.81277365594783,3.92375119738988,-3.03766158493069));
#72240=CARTESIAN_POINT('Ctrl Pts',(9.85252898008688,4.92914915570359,-1.7389878082477));
#72241=CARTESIAN_POINT('Ctrl Pts',(9.89228430422595,5.22578623143186,0.108389389631662));
#72242=CARTESIAN_POINT('Ctrl Pts',(9.932039628365,4.67750859358339,1.65653998458705));
#72243=CARTESIAN_POINT('Ctrl Pts',(9.97179495250406,4.12923095573491,3.20469057954244));
#72244=CARTESIAN_POINT('Ctrl Pts',(10.0115502766431,2.73603860430971,4.4536145715738));
#72245=CARTESIAN_POINT('Ctrl Pts',(10.0513056007822,1.13739467953943,4.83006673934611));
#72246=CARTESIAN_POINT('Ctrl Pts',(10.0910609249212,-0.461249245230903,
5.20651890711843));
#72247=CARTESIAN_POINT('Ctrl Pts',(10.1308162490603,-2.26534474334642,4.71049925063156));
#72248=CARTESIAN_POINT('Ctrl Pts',(10.1705715731993,-3.44682771344815,3.56967646676669));
#72249=CARTESIAN_POINT('Ctrl Pts',(10.2025181447515,-4.3962434473012,2.65293443328137));
#72250=CARTESIAN_POINT('Ctrl Pts',(10.2344647163037,-4.94361315650885,1.31981701000383));
#72251=CARTESIAN_POINT('Ctrl Pts',(10.2664112878559,-4.95582936423354,-0.0043891145566411));
#72252=CARTESIAN_POINT('Origin',(10.45,0.,0.));
#72253=CARTESIAN_POINT('',(11.1217887121442,-4.96143148149888,0.00174928188396612));
#72254=CARTESIAN_POINT('',(11.0164112878559,-4.96043743303216,0.00264048323268159));
#72255=CARTESIAN_POINT('',(10.45,-4.954,-6.06690024297599E-16));
#72256=CARTESIAN_POINT('Ctrl Pts',(11.1217887121442,-4.96143148149888,0.00174928188396612));
#72257=CARTESIAN_POINT('Ctrl Pts',(11.1194679227802,-4.96186820307519,0.097664209125269));
#72258=CARTESIAN_POINT('Ctrl Pts',(11.1171471334162,-4.95932850373442,0.193555553937918));
#72259=CARTESIAN_POINT('Ctrl Pts',(11.1148263440521,-4.95373941917952,0.289268832843753));
#72260=CARTESIAN_POINT('Ctrl Pts',(11.0750710199131,-4.85799791348065,1.92884564507605));
#72261=CARTESIAN_POINT('Ctrl Pts',(11.035315695774,-3.8674451554344,3.51617081775305));
#72262=CARTESIAN_POINT('Ctrl Pts',(10.995560371635,-2.43673622305456,4.3226759385873));
#72263=CARTESIAN_POINT('Ctrl Pts',(10.9558050474959,-1.00602729067465,5.1291810594216));
#72264=CARTESIAN_POINT('Ctrl Pts',(10.9160497233569,0.864837816038947,5.15486612841308));
#72265=CARTESIAN_POINT('Ctrl Pts',(10.8762943992178,2.31714832763268,4.38794192287648));
#72266=CARTESIAN_POINT('Ctrl Pts',(10.8365390750788,3.76945883922638,3.62101771733989));
#72267=CARTESIAN_POINT('Ctrl Pts',(10.7967837509397,4.8032147557003,2.06148423727525));
#72268=CARTESIAN_POINT('Ctrl Pts',(10.7570284268006,4.94393112606734,0.425153750413206));
#72269=CARTESIAN_POINT('Ctrl Pts',(10.7172731026616,5.08464749643438,-1.21117673644879));
#72270=CARTESIAN_POINT('Ctrl Pts',(10.6775177785225,4.3323243206947,-2.92430423010813));
#72271=CARTESIAN_POINT('Ctrl Pts',(10.6377624543835,3.03227137601965,-3.92791814998222));
#72272=CARTESIAN_POINT('Ctrl Pts',(10.5980071302444,1.73221843134455,-4.93153206985633));
#72273=CARTESIAN_POINT('Ctrl Pts',(10.5582518061054,-0.115564282265953,
-5.22563241594505));
#72274=CARTESIAN_POINT('Ctrl Pts',(10.5184964819663,-1.66296061250703,-4.67522969404051));
#72275=CARTESIAN_POINT('Ctrl Pts',(10.4787411578273,-3.2103569427481,-4.12482697213597));
#72276=CARTESIAN_POINT('Ctrl Pts',(10.4389858336882,-4.45736688961978,-2.72992118223817));
#72277=CARTESIAN_POINT('Ctrl Pts',(10.3992305095492,-4.83162376182417,-1.13076191789604));
#72278=CARTESIAN_POINT('Ctrl Pts',(10.3900832437475,-4.91773617977793,-0.762812840208963));
#72279=CARTESIAN_POINT('Ctrl Pts',(10.3809359779458,-4.95764419208994,-0.384050382814731));
#72280=CARTESIAN_POINT('Ctrl Pts',(10.3717887121442,-4.95413490991508,-0.00455749466325095));
#72281=CARTESIAN_POINT('Ctrl Pts',(10.2664112878559,-4.95582936423354,-0.0043891145566411));
#72282=CARTESIAN_POINT('Ctrl Pts',(10.2742200404428,-4.95881539181137,-0.328066977259775));
#72283=CARTESIAN_POINT('Ctrl Pts',(10.2820287930296,-4.92982769828898,-0.651212418182936));
#72284=CARTESIAN_POINT('Ctrl Pts',(10.2898375456165,-4.86692238031873,-0.967614544916926));
#72285=CARTESIAN_POINT('Ctrl Pts',(10.3295928697555,-4.54666363499955,-2.57845686149303));
#72286=CARTESIAN_POINT('Ctrl Pts',(10.3693481938946,-3.34727570227304,-4.01451558340236));
#72287=CARTESIAN_POINT('Ctrl Pts',(10.4091035180337,-1.81926718422331,-4.61665228016908));
#72288=CARTESIAN_POINT('Ctrl Pts',(10.4488588421727,-0.291258666173671,
-5.21878897693576));
#72289=CARTESIAN_POINT('Ctrl Pts',(10.4886141663118,1.56537043719918,-4.98700364855995));
#72290=CARTESIAN_POINT('Ctrl Pts',(10.5283694904508,2.8984435578328,-4.02768373952569));
#72291=CARTESIAN_POINT('Ctrl Pts',(10.5681248145899,4.23151667846645,-3.0683638304914));
#72292=CARTESIAN_POINT('Ctrl Pts',(10.6078801387289,5.04103381636084,-1.38150934079872));
#72293=CARTESIAN_POINT('Ctrl Pts',(10.647635462868,4.95543366446481,0.25862822868162));
#72294=CARTESIAN_POINT('Ctrl Pts',(10.687390787007,4.86983351256878,1.89876579816191));
#72295=CARTESIAN_POINT('Ctrl Pts',(10.7271461111461,3.88911607088231,3.49218644742981));
#72296=CARTESIAN_POINT('Ctrl Pts',(10.7669014352851,2.46342209297707,4.30752399359709));
#72297=CARTESIAN_POINT('Ctrl Pts',(10.8066567594242,1.03772811507175,5.12286153976442));
#72298=CARTESIAN_POINT('Ctrl Pts',(10.8464120835633,-0.832942399052437,
5.16011598283106));
#72299=CARTESIAN_POINT('Ctrl Pts',(10.8861674077023,-2.28996799624358,4.40218785829981));
#72300=CARTESIAN_POINT('Ctrl Pts',(10.9259227318414,-3.74699359343464,3.64425973376861));
#72301=CARTESIAN_POINT('Ctrl Pts',(10.9656780559804,-4.79037427369275,2.09114904163959));
#72302=CARTESIAN_POINT('Ctrl Pts',(11.0054333801195,-4.94120740338486,0.455720045989624));
#72303=CARTESIAN_POINT('Ctrl Pts',(11.0090926826983,-4.95509092898562,0.30518600631491));
#72304=CARTESIAN_POINT('Ctrl Pts',(11.0127519852771,-4.96141244178186,0.153954533696844));
#72305=CARTESIAN_POINT('Ctrl Pts',(11.0164112878559,-4.96043743303216,0.00264048323268159));
#72306=CARTESIAN_POINT('Origin',(10.45,0.,0.));
#72307=CARTESIAN_POINT('',(11.8717887121442,-4.94883061351211,0.0036397403582919));
#72308=CARTESIAN_POINT('',(11.7664112878559,-4.94768798497716,0.00300517406437754));
#72309=CARTESIAN_POINT('',(10.45,-4.954,-6.06690024297599E-16));
#72310=CARTESIAN_POINT('Ctrl Pts',(11.8717887121442,-4.94883061351211,0.0036397403582919));
#72311=CARTESIAN_POINT('Ctrl Pts',(11.8579998676145,-4.95272244476274,0.577253372849803));
#72312=CARTESIAN_POINT('Ctrl Pts',(11.8442110230848,-4.86065783541348,1.14965663724327));
#72313=CARTESIAN_POINT('Ctrl Pts',(11.8304221785551,-4.66717465558493,1.68543508479369));
#72314=CARTESIAN_POINT('Ctrl Pts',(11.7906668544161,-4.10933338665354,3.23016537769288));
#72315=CARTESIAN_POINT('Ctrl Pts',(11.750911530277,-2.70844405945764,4.47044964480083));
#72316=CARTESIAN_POINT('Ctrl Pts',(11.711156206138,-1.10750265898756,4.83700822318128));
#72317=CARTESIAN_POINT('Ctrl Pts',(11.6714008819989,0.493438741482567,5.20356680156174));
#72318=CARTESIAN_POINT('Ctrl Pts',(11.6316455578599,2.29443221522694,4.69639969121456));
#72319=CARTESIAN_POINT('Ctrl Pts',(11.5918902337208,3.46883746302233,3.54829217313353));
#72320=CARTESIAN_POINT('Ctrl Pts',(11.5521349095817,4.64324271081769,2.40018465505254));
#72321=CARTESIAN_POINT('Ctrl Pts',(11.5123795854427,5.19105973266421,0.611136729237761));
#72322=CARTESIAN_POINT('Ctrl Pts',(11.4726242613036,4.86084529266991,-0.99769420741862));
#72323=CARTESIAN_POINT('Ctrl Pts',(11.4328689371646,4.5306308526756,-2.606525144075));
#72324=CARTESIAN_POINT('Ctrl Pts',(11.3931136130255,3.32238495084048,-4.03513909157292));
#72325=CARTESIAN_POINT('Ctrl Pts',(11.3533582888865,1.79068191982516,-4.62781470597075));
#72326=CARTESIAN_POINT('Ctrl Pts',(11.3136029647474,0.258978888809789,-5.2204903203686));
#72327=CARTESIAN_POINT('Ctrl Pts',(11.2738476406084,-1.59618127138576,-4.97722760166629));
#72328=CARTESIAN_POINT('Ctrl Pts',(11.2340923164693,-2.92329622480781,-4.00968201642128));
#72329=CARTESIAN_POINT('Ctrl Pts',(11.1966577816943,-4.17293842871952,-3.09861866474033));
#72330=CARTESIAN_POINT('Ctrl Pts',(11.1592232469192,-4.95438712439842,-1.54536685667392));
#72331=CARTESIAN_POINT('Ctrl Pts',(11.1217887121442,-4.96143148149888,0.00174928188396612));
#72332=CARTESIAN_POINT('Ctrl Pts',(11.0164112878559,-4.96043743303216,0.00264048323268159));
#72333=CARTESIAN_POINT('Ctrl Pts',(11.0525073094161,-4.95081977062441,-1.48994864005102));
#72334=CARTESIAN_POINT('Ctrl Pts',(11.0886033309764,-4.23123553683844,-2.99057275780401));
#72335=CARTESIAN_POINT('Ctrl Pts',(11.1246993525366,-3.05650459196268,-3.90909082049691));
#72336=CARTESIAN_POINT('Ctrl Pts',(11.1644546766757,-1.76268307172244,-4.92072539216228));
#72337=CARTESIAN_POINT('Ctrl Pts',(11.2042100008148,0.0832455478841035,
-5.22624723632215));
#72338=CARTESIAN_POINT('Ctrl Pts',(11.2439653249538,1.63401612753167,-4.68542449075305));
#72339=CARTESIAN_POINT('Ctrl Pts',(11.2837206490929,3.18478670717929,-4.14460174518394));
#72340=CARTESIAN_POINT('Ctrl Pts',(11.3234759732319,4.44039924686796,-2.75743440988578));
#72341=CARTESIAN_POINT('Ctrl Pts',(11.363231297371,4.82453854021408,-1.16062019522803));
#72342=CARTESIAN_POINT('Ctrl Pts',(11.40298662151,5.20867783356018,0.436194019429668));
#72343=CARTESIAN_POINT('Ctrl Pts',(11.4427419456491,4.72134388056388,2.24265511344687));
#72344=CARTESIAN_POINT('Ctrl Pts',(11.4824972697881,3.58621871594613,3.42961319757489));
#72345=CARTESIAN_POINT('Ctrl Pts',(11.5222525939272,2.4510935513283,4.61657128170297));
#72346=CARTESIAN_POINT('Ctrl Pts',(11.5620079180662,0.668177175088912,5.18402635594168));
#72347=CARTESIAN_POINT('Ctrl Pts',(11.6017632422053,-0.944187343665765,
4.87152148960091));
#72348=CARTESIAN_POINT('Ctrl Pts',(11.6415185663444,-2.55655186242035,4.55901662326017));
#72349=CARTESIAN_POINT('Ctrl Pts',(11.6812738904834,-3.99836452369029,3.36655181634004));
#72350=CARTESIAN_POINT('Ctrl Pts',(11.7210292146225,-4.60784588900943,1.84145801655129));
#72351=CARTESIAN_POINT('Ctrl Pts',(11.7361565723669,-4.83976055330752,1.26114229776651));
#72352=CARTESIAN_POINT('Ctrl Pts',(11.7512839301114,-4.95116280464578,0.632665560951985));
#72353=CARTESIAN_POINT('Ctrl Pts',(11.7664112878559,-4.94768798497716,0.00300517406437754));
#72354=CARTESIAN_POINT('Origin',(10.45,0.,0.));
#72355=CARTESIAN_POINT('',(12.6217887121442,-4.94819583789813,-0.00332016549414282));
#72356=CARTESIAN_POINT('',(12.5164112878559,-4.9494435771879,-0.00388817816282298));
#72357=CARTESIAN_POINT('',(10.45,-4.954,-6.06690024297599E-16));
#72358=CARTESIAN_POINT('Ctrl Pts',(12.6217887121442,-4.94819583789813,-0.00332016549414282));
#72359=CARTESIAN_POINT('Ctrl Pts',(12.5965318124488,-4.94174563760587,1.04770119792139));
#72360=CARTESIAN_POINT('Ctrl Pts',(12.5712749127535,-4.61431031278361,2.1023936236481));
#72361=CARTESIAN_POINT('Ctrl Pts',(12.5460180130581,-3.99557088579909,2.94255399055693));
#72362=CARTESIAN_POINT('Ctrl Pts',(12.5062626889191,-3.02165141135531,4.26499847575186));
#72363=CARTESIAN_POINT('Ctrl Pts',(12.46650736478,-1.32599801317663,5.05591915668782));
#72364=CARTESIAN_POINT('Ctrl Pts',(12.426752040641,0.313099185600184,4.95229033789058));
#72365=CARTESIAN_POINT('Ctrl Pts',(12.3869967165019,1.95219638437709,4.84866151909333));
#72366=CARTESIAN_POINT('Ctrl Pts',(12.3472413923628,3.53473738375218,3.85048320056279));
#72367=CARTESIAN_POINT('Ctrl Pts',(12.3074860682238,4.33434966526403,2.41591052607779));
#72368=CARTESIAN_POINT('Ctrl Pts',(12.2677307440847,5.13396194677585,0.981337851592837));
#72369=CARTESIAN_POINT('Ctrl Pts',(12.2279754199457,5.15064551042452,-0.889629178846445));
#72370=CARTESIAN_POINT('Ctrl Pts',(12.1882200958066,4.3767427459812,-2.33823301368551));
#72371=CARTESIAN_POINT('Ctrl Pts',(12.1484647716676,3.60283998153789,-3.78683684852453));
#72372=CARTESIAN_POINT('Ctrl Pts',(12.1087094475285,2.03835088900258,-4.81307748776327));
#72373=CARTESIAN_POINT('Ctrl Pts',(12.0689541233895,0.40136231901543,-4.94591942713005));
#72374=CARTESIAN_POINT('Ctrl Pts',(12.0291987992504,-1.23562625097182,-5.07876136649683));
#72375=CARTESIAN_POINT('Ctrl Pts',(11.9894434751114,-2.94511429841096,-4.31820460599157));
#72376=CARTESIAN_POINT('Ctrl Pts',(11.9496881509723,-3.94246171679709,-3.01333806639369));
#72377=CARTESIAN_POINT('Ctrl Pts',(11.9237216713629,-4.59388644955471,-2.16105497910461));
#72378=CARTESIAN_POINT('Ctrl Pts',(11.8977551917536,-4.94150170668492,-1.07656148024989));
#72379=CARTESIAN_POINT('Ctrl Pts',(11.8717887121442,-4.94883061351211,0.0036397403582919));
#72380=CARTESIAN_POINT('Ctrl Pts',(11.7664112878559,-4.94768798497716,0.00300517406437754));
#72381=CARTESIAN_POINT('Ctrl Pts',(11.7910392542505,-4.94203083430539,-1.02210807507116));
#72382=CARTESIAN_POINT('Ctrl Pts',(11.815667220645,-4.63188980484689,-2.05035861141485));
#72383=CARTESIAN_POINT('Ctrl Pts',(11.8402951870396,-4.04158227195343,-2.87903179951418));
#72384=CARTESIAN_POINT('Ctrl Pts',(11.8800505111787,-3.08868722020987,-4.2167050231336));
#72385=CARTESIAN_POINT('Ctrl Pts',(11.9198058353177,-1.40574704735437,-5.03432867771487));
#72386=CARTESIAN_POINT('Ctrl Pts',(11.9595611594568,0.234783383036354,-4.95662063573885));
#72387=CARTESIAN_POINT('Ctrl Pts',(11.9993164835959,1.87531381342699,-4.87891259376283));
#72388=CARTESIAN_POINT('Ctrl Pts',(12.0390718077349,3.4734345013528,-3.90587285522962));
#72389=CARTESIAN_POINT('Ctrl Pts',(12.078827131874,4.29562198716748,-2.48411817491548));
#72390=CARTESIAN_POINT('Ctrl Pts',(12.118582456013,5.11780947298219,-1.0623634946013));
#72391=CARTESIAN_POINT('Ctrl Pts',(12.1583377801521,5.16406375668566,0.808106127493931));
#72392=CARTESIAN_POINT('Ctrl Pts',(12.1980931042911,4.41315452540982,2.26876144590765));
#72393=CARTESIAN_POINT('Ctrl Pts',(12.2378484284302,3.66224529413399,3.72941676432133));
#72394=CARTESIAN_POINT('Ctrl Pts',(12.2776037525692,2.11417254787894,4.78025777905362));
#72395=CARTESIAN_POINT('Ctrl Pts',(12.3173590767083,0.47948817749778,4.93895762800431));
#72396=CARTESIAN_POINT('Ctrl Pts',(12.3571144008473,-1.15519619288338,5.09765747695501));
#72397=CARTESIAN_POINT('Ctrl Pts',(12.3968697249864,-2.8764921873906,4.36421616012411));
#72398=CARTESIAN_POINT('Ctrl Pts',(12.4366250491254,-3.89433995478385,3.07527684609959));
#72399=CARTESIAN_POINT('Ctrl Pts',(12.4632204620356,-4.57525709581401,2.21300559023716));
#72400=CARTESIAN_POINT('Ctrl Pts',(12.4898158749457,-4.94135952703255,1.10213190132163));
#72401=CARTESIAN_POINT('Ctrl Pts',(12.5164112878559,-4.9494435771879,-0.00388817816282298));
#72402=CARTESIAN_POINT('Origin',(10.45,0.,0.));
#72403=CARTESIAN_POINT('',(13.3717887121442,-4.96094723257582,-0.00223694760002224));
#72404=CARTESIAN_POINT('',(13.2664112878559,-4.96176967234081,-0.00129340989018459));
#72405=CARTESIAN_POINT('',(10.45,-4.954,-6.06690024297599E-16));
#72406=CARTESIAN_POINT('Ctrl Pts',(13.3717887121442,-4.96094723257582,-0.00223694760002224));
#72407=CARTESIAN_POINT('Ctrl Pts',(13.3350637572832,-4.95241483308039,1.51594650197974));
#72408=CARTESIAN_POINT('Ctrl Pts',(13.2983388024221,-4.2041562175098,3.04140006639481));
#72409=CARTESIAN_POINT('Ctrl Pts',(13.2616138475611,-2.99433500310446,3.95691402231224));
#72410=CARTESIAN_POINT('Ctrl Pts',(13.2218585234221,-1.68468507403037,4.94797185230984));
#72411=CARTESIAN_POINT('Ctrl Pts',(13.182103199283,0.165842044445711,5.22427848283428));
#72412=CARTESIAN_POINT('Ctrl Pts',(13.1423478751439,1.70787054211769,4.65901157995497));
#72413=CARTESIAN_POINT('Ctrl Pts',(13.1025925510049,3.24989903978976,4.09374467707563));
#72414=CARTESIAN_POINT('Ctrl Pts',(13.0628372268658,4.48342891665779,2.68690424079239));
#72415=CARTESIAN_POINT('Ctrl Pts',(13.0230819027268,4.84228071600508,1.08421776327136));
#72416=CARTESIAN_POINT('Ctrl Pts',(12.9833265785877,5.20113251535238,-0.518468714249673));
#72417=CARTESIAN_POINT('Ctrl Pts',(12.9435712544487,4.68530623717908,-2.31700123300836));
#72418=CARTESIAN_POINT('Ctrl Pts',(12.9038159303096,3.53156164500038,-3.48586905066012));
#72419=CARTESIAN_POINT('Ctrl Pts',(12.8640606061706,2.37781705282174,-4.65473686831181));
#72420=CARTESIAN_POINT('Ctrl Pts',(12.8243052820315,0.586154146637735,-5.19393998485644));
#72421=CARTESIAN_POINT('Ctrl Pts',(12.7845499578925,-1.02106942347329,-4.8559888718196));
#72422=CARTESIAN_POINT('Ctrl Pts',(12.7447946337534,-2.62829299358441,-4.51803775878274));
#72423=CARTESIAN_POINT('Ctrl Pts',(12.7050393096143,-4.05107722762262,-3.30293241616428));
#72424=CARTESIAN_POINT('Ctrl Pts',(12.6652839854753,-4.63637656928722,-1.76839560012806));
#72425=CARTESIAN_POINT('Ctrl Pts',(12.6507855610316,-4.84983020011129,-1.20876323477365));
#72426=CARTESIAN_POINT('Ctrl Pts',(12.6362871365879,-4.95189849906051,-0.6066465440279));
#72427=CARTESIAN_POINT('Ctrl Pts',(12.6217887121442,-4.94819583789813,-0.00332016549414282));
#72428=CARTESIAN_POINT('Ctrl Pts',(12.5164112878559,-4.9494435771879,-0.00388817816282298));
#72429=CARTESIAN_POINT('Ctrl Pts',(12.5295711990848,-4.95344371746674,-0.551167745228975));
#72430=CARTESIAN_POINT('Ctrl Pts',(12.5427311103137,-4.8697846040195,-1.09725892699675));
#72431=CARTESIAN_POINT('Ctrl Pts',(12.5558910215426,-4.69323192829556,-1.61145444577539));
#72432=CARTESIAN_POINT('Ctrl Pts',(12.5956463456817,-4.15987659413477,-3.16480911240745));
#72433=CARTESIAN_POINT('Ctrl Pts',(12.6354016698207,-2.77876638553401,-4.42708113445346));
#72434=CARTESIAN_POINT('Ctrl Pts',(12.6751569939598,-1.18381884452863,-4.81889866120061));
#72435=CARTESIAN_POINT('Ctrl Pts',(12.7149123180988,0.41112869647675,-5.21071618794776));
#72436=CARTESIAN_POINT('Ctrl Pts',(12.7546676422379,2.2199135698868,-4.73207921939605));
#72437=CARTESIAN_POINT('Ctrl Pts',(12.794422966377,3.41231929197536,-3.60267795024686));
#72438=CARTESIAN_POINT('Ctrl Pts',(12.834178290516,4.60472501406402,-2.47327668109757));
#72439=CARTESIAN_POINT('Ctrl Pts',(12.8739336146551,5.1807515848311,-0.693111111350794));
#72440=CARTESIAN_POINT('Ctrl Pts',(12.9136889387941,4.87600783142616,0.920738286079608));
#72441=CARTESIAN_POINT('Ctrl Pts',(12.9534442629332,4.57126407802125,2.53458768350987));
#72442=CARTESIAN_POINT('Ctrl Pts',(12.9931995870722,3.3857500004444,3.98212090862372));
#72443=CARTESIAN_POINT('Ctrl Pts',(13.0329549112113,1.86360622225035,4.59893283403573));
#72444=CARTESIAN_POINT('Ctrl Pts',(13.0727102353503,0.341462444056204,5.21574475944778));
#72445=CARTESIAN_POINT('Ctrl Pts',(13.1124655594894,-1.51731103475523,5.00183538515791));
#72446=CARTESIAN_POINT('Ctrl Pts',(13.1522208836284,-2.85955339649474,4.05538724860864));
#72447=CARTESIAN_POINT('Ctrl Pts',(13.1902843517043,-4.14467433041966,3.14921683719545));
#72448=CARTESIAN_POINT('Ctrl Pts',(13.2283478197801,-4.9562924078719,1.57152987054922));
#72449=CARTESIAN_POINT('Ctrl Pts',(13.2664112878559,-4.96176967234081,-0.00129340989018459));
#72450=CARTESIAN_POINT('Origin',(10.45,0.,0.));
#72451=CARTESIAN_POINT('',(14.1217887121442,-4.95503454872885,0.00449354721262798));
#72452=CARTESIAN_POINT('',(14.0164112878559,-4.95334288452853,0.00456658721771082));
#72453=CARTESIAN_POINT('',(10.45,-4.954,-6.06690024297599E-16));
#72454=CARTESIAN_POINT('Ctrl Pts',(14.1217887121442,-4.95503454872885,0.00449354721262798));
#72455=CARTESIAN_POINT('Ctrl Pts',(14.1133510262565,-4.95828270233056,0.35438528685295));
#72456=CARTESIAN_POINT('Ctrl Pts',(14.1049133403689,-4.92438729661826,0.703652274904061));
#72457=CARTESIAN_POINT('Ctrl Pts',(14.0964756544813,-4.85102004306605,1.04442100350354));
#72458=CARTESIAN_POINT('Ctrl Pts',(14.0567203303422,-4.50534007998143,2.65000000257061));
#72459=CARTESIAN_POINT('Ctrl Pts',(14.0169650062031,-3.28340342420688,4.06692158810787));
#72460=CARTESIAN_POINT('Ctrl Pts',(13.9772096820641,-1.74606834507353,4.6448311083526));
#72461=CARTESIAN_POINT('Ctrl Pts',(13.937454357925,-0.208733265940278,5.2227406285973));
#72462=CARTESIAN_POINT('Ctrl Pts',(13.897699033786,1.64400023655164,4.96163808354953));
#72463=CARTESIAN_POINT('Ctrl Pts',(13.8579437096469,2.96174364117349,3.98136726449046));
#72464=CARTESIAN_POINT('Ctrl Pts',(13.8181883855079,4.27948704579556,3.00109644543122));
#72465=CARTESIAN_POINT('Ctrl Pts',(13.7784330613688,5.06224035254725,1.30165735236046));
#72466=CARTESIAN_POINT('Ctrl Pts',(13.7386777372298,4.95072661948288,-0.336922290641983));
#72467=CARTESIAN_POINT('Ctrl Pts',(13.6989224130907,4.83921288641853,-1.97550193364414));
#72468=CARTESIAN_POINT('Ctrl Pts',(13.6591670889517,3.83343211353822,-3.55322212657819));
#72469=CARTESIAN_POINT('Ctrl Pts',(13.6194117648126,2.39502890487168,-4.34592305909999));
#72470=CARTESIAN_POINT('Ctrl Pts',(13.5796564406735,0.956625696205059,-5.13862399162183));
#72471=CARTESIAN_POINT('Ctrl Pts',(13.5399011165345,-0.914399948247869,
-5.14630566373156));
#72472=CARTESIAN_POINT('Ctrl Pts',(13.5001457923954,-2.35926357361136,-4.36544225491741));
#72473=CARTESIAN_POINT('Ctrl Pts',(13.4603904682564,-3.80412719897494,-3.58457884610321));
#72474=CARTESIAN_POINT('Ctrl Pts',(13.4206351441173,-4.82282880524895,-2.01517035636507));
#72475=CARTESIAN_POINT('Ctrl Pts',(13.3808798199783,-4.94779323854984,-0.377561596760541));
#72476=CARTESIAN_POINT('Ctrl Pts',(13.3778494507002,-4.95731871438791,-0.252734057757678));
#72477=CARTESIAN_POINT('Ctrl Pts',(13.3748190814222,-4.96165128575701,-0.127510252943251));
#72478=CARTESIAN_POINT('Ctrl Pts',(13.3717887121442,-4.96094723257582,-0.00223694760002224));
#72479=CARTESIAN_POINT('Ctrl Pts',(13.2664112878559,-4.96176967234081,-0.00129340989018459));
#72480=CARTESIAN_POINT('Ctrl Pts',(13.2681031439191,-4.96201312737973,-0.0712027150045571));
#72481=CARTESIAN_POINT('Ctrl Pts',(13.2697949999824,-4.96066392993926,-0.141102411174969));
#72482=CARTESIAN_POINT('Ctrl Pts',(13.2714868560456,-4.9576928696551,-0.210933102554134));
#72483=CARTESIAN_POINT('Ctrl Pts',(13.3112421801847,-4.88787873640841,-1.85181841835902));
#72484=CARTESIAN_POINT('Ctrl Pts',(13.3509975043237,-3.92253922524754,-3.45460215116033));
#72485=CARTESIAN_POINT('Ctrl Pts',(13.3907528284628,-2.50475675373321,-4.28362054437715));
#72486=CARTESIAN_POINT('Ctrl Pts',(13.4305081526018,-1.08697428221864,-5.11263893759411));
#72487=CARTESIAN_POINT('Ctrl Pts',(13.4702634767409,0.783251149649558,-5.16789199122628));
#72488=CARTESIAN_POINT('Ctrl Pts',(13.5100188008799,2.24750237759368,-4.4240190354804));
#72489=CARTESIAN_POINT('Ctrl Pts',(13.549774125019,3.71175360553764,-3.68014607973459));
#72490=CARTESIAN_POINT('Ctrl Pts',(13.589529449158,4.77003062955761,-2.13714711461092));
#72491=CARTESIAN_POINT('Ctrl Pts',(13.6292847732971,4.93659352413465,-0.503245209668175));
#72492=CARTESIAN_POINT('Ctrl Pts',(13.6690400974362,5.10315641871169,1.13065669527456));
#72493=CARTESIAN_POINT('Ctrl Pts',(13.7087954215752,4.3780051838458,2.85546154003637));
#72494=CARTESIAN_POINT('Ctrl Pts',(13.7485507457143,3.09397791279514,3.87949894170858));
#72495=CARTESIAN_POINT('Ctrl Pts',(13.7883060698533,1.8099506417444,4.90353634338085));
#72496=CARTESIAN_POINT('Ctrl Pts',(13.8280613939924,-0.032952665491161,
5.22680630196345));
#72497=CARTESIAN_POINT('Ctrl Pts',(13.8678167181314,-1.58885546158286,4.70093072548197));
#72498=CARTESIAN_POINT('Ctrl Pts',(13.9075720422705,-3.14475825767447,4.17505514900052));
#72499=CARTESIAN_POINT('Ctrl Pts',(13.9473273664095,-4.41366054262224,2.8000340374551));
#72500=CARTESIAN_POINT('Ctrl Pts',(13.9870826905486,-4.81314723285944,1.20699009043144));
#72501=CARTESIAN_POINT('Ctrl Pts',(13.996858889651,-4.91138467670136,0.815245962008683));
#72502=CARTESIAN_POINT('Ctrl Pts',(14.0066350887534,-4.95704740833786,0.410317704040501));
#72503=CARTESIAN_POINT('Ctrl Pts',(14.0164112878559,-4.95334288452853,0.00456658721771082));
#72504=CARTESIAN_POINT('Origin',(10.45,0.,0.));
#72505=CARTESIAN_POINT('',(14.8717887121442,-4.94581096318579,-1.93332609692235E-5));
#72506=CARTESIAN_POINT('',(14.7664112878559,-4.9459710090011,-0.000934506679922751));
#72507=CARTESIAN_POINT('',(10.45,-4.954,-6.06690024297599E-16));
#72508=CARTESIAN_POINT('Ctrl Pts',(14.8717887121442,-4.94581103525318,-1.93330908274114E-5));
#72509=CARTESIAN_POINT('Ctrl Pts',(14.8518829710909,-4.94578225734086,0.829322250681016));
#72510=CARTESIAN_POINT('Ctrl Pts',(14.8319772300376,-4.74850012339904,1.65867670117964));
#72511=CARTESIAN_POINT('Ctrl Pts',(14.8120714889842,-4.35404071127217,2.38023952058872));
#72512=CARTESIAN_POINT('Ctrl Pts',(14.7723161648452,-3.56623473375009,3.82132949033526));
#72513=CARTESIAN_POINT('Ctrl Pts',(14.7325608407061,-1.99194317595282,4.83246848243075));
#72514=CARTESIAN_POINT('Ctrl Pts',(14.6928055165671,-0.353752134595302,
4.94955251695112));
#72515=CARTESIAN_POINT('Ctrl Pts',(14.653050192428,1.28443890676203,5.06663655147147));
#72516=CARTESIAN_POINT('Ctrl Pts',(14.613294868289,2.9865294316797,4.28966562841695));
#72517=CARTESIAN_POINT('Ctrl Pts',(14.5735395441499,3.97127473198152,2.97526262604042));
#72518=CARTESIAN_POINT('Ctrl Pts',(14.5337842200109,4.95602003228346,1.66085962366375));
#72519=CARTESIAN_POINT('Ctrl Pts',(14.4940288958718,5.22342010796947,-0.19097545803513));
#72520=CARTESIAN_POINT('Ctrl Pts',(14.4542735717327,4.65074065611181,-1.73026646513667));
#72521=CARTESIAN_POINT('Ctrl Pts',(14.4145182475937,4.07806120425415,-3.2695574722382));
#72522=CARTESIAN_POINT('Ctrl Pts',(14.3747629234546,2.66530222485308,-4.49630440474226));
#72523=CARTESIAN_POINT('Ctrl Pts',(14.3350075993156,1.06090776975382,-4.84744111824618));
#72524=CARTESIAN_POINT('Ctrl Pts',(14.2952522751765,-0.543486685345351,
-5.19857783175009));
#72525=CARTESIAN_POINT('Ctrl Pts',(14.2554969510375,-2.33951661614259,-4.67410432625374));
#72526=CARTESIAN_POINT('Ctrl Pts',(14.2157416268984,-3.50281994634389,-3.51474936720718));
#72527=CARTESIAN_POINT('Ctrl Pts',(14.184423988647,-4.41922331270755,-2.601456368126));
#72528=CARTESIAN_POINT('Ctrl Pts',(14.1531063503956,-4.94297857735968,-1.29417804060499));
#72529=CARTESIAN_POINT('Ctrl Pts',(14.1217887121442,-4.95503454872885,0.00449354721262798));
#72530=CARTESIAN_POINT('Ctrl Pts',(14.0164112878559,-4.95334288452853,0.00456658721771082));
#72531=CARTESIAN_POINT('Ctrl Pts',(14.0463904128925,-4.9419828067194,-1.23968624944593));
#72532=CARTESIAN_POINT('Ctrl Pts',(14.0763695379291,-4.46638886767634,-2.4916769872725));
#72533=CARTESIAN_POINT('Ctrl Pts',(14.1063486629658,-3.61905378866574,-3.39494639697394));
#72534=CARTESIAN_POINT('Ctrl Pts',(14.1461039871048,-2.49540255870816,-4.59277215485382));
#72535=CARTESIAN_POINT('Ctrl Pts',(14.1858593112439,-0.718029003266378,
-5.17735688811155));
#72536=CARTESIAN_POINT('Ctrl Pts',(14.2256146353829,0.897267914964357,-4.88038130194328));
#72537=CARTESIAN_POINT('Ctrl Pts',(14.265369959522,2.512564833195,-4.58340571577504));
#72538=CARTESIAN_POINT('Ctrl Pts',(14.305125283661,3.96578511421461,-3.40486981018091));
#72539=CARTESIAN_POINT('Ctrl Pts',(14.3448806078001,4.58991332156997,-1.88571128862735));
#72540=CARTESIAN_POINT('Ctrl Pts',(14.3846359319391,5.21404152892534,-0.366552767073803));
#72541=CARTESIAN_POINT('Ctrl Pts',(14.4243912560782,5.00907766261646,1.49322837043917));
#72542=CARTESIAN_POINT('Ctrl Pts',(14.4641465802172,4.06909834993017,2.84000879966555));
#72543=CARTESIAN_POINT('Ctrl Pts',(14.5039019043563,3.12911903724383,4.186789228892));
#72544=CARTESIAN_POINT('Ctrl Pts',(14.5436572284954,1.45412427817999,5.02056894983181));
#72545=CARTESIAN_POINT('Ctrl Pts',(14.5834125526344,-0.18707793932848,4.95865034139318));
#72546=CARTESIAN_POINT('Ctrl Pts',(14.6231678767735,-1.82828015683685,4.89673173295456));
#72547=CARTESIAN_POINT('Ctrl Pts',(14.6629232009125,-3.43568983278986,3.93911479513759));
#72548=CARTESIAN_POINT('Ctrl Pts',(14.7026785250516,-4.27151994303955,2.52533735168145));
#72549=CARTESIAN_POINT('Ctrl Pts',(14.7239227793197,-4.7181667198327,1.76984992609218));
#72550=CARTESIAN_POINT('Ctrl Pts',(14.7451670335878,-4.94448376706638,0.884102802980237));
#72551=CARTESIAN_POINT('Ctrl Pts',(14.7664112878559,-4.9459710090011,-0.000934506679922751));
#72552=CARTESIAN_POINT('Origin',(10.45,0.,0.));
#72553=CARTESIAN_POINT('',(15.6217887121442,-4.95510573438616,-0.00448604574660338));
#72554=CARTESIAN_POINT('',(15.5164112878559,-4.95678235276575,-0.00420182901399404));
#72555=CARTESIAN_POINT('',(10.45,-4.954,-6.06690024297599E-16));
#72556=CARTESIAN_POINT('Ctrl Pts',(15.6217887121442,-4.95510573438616,-0.00448604574660338));
#72557=CARTESIAN_POINT('Ctrl Pts',(15.5904149159252,-4.94303076991488,1.29646632009306));
#72558=CARTESIAN_POINT('Ctrl Pts',(15.5590411197062,-4.41719278747976,2.60605571081289));
#72559=CARTESIAN_POINT('Ctrl Pts',(15.5276673234872,-3.49785572892943,3.51968975768936));
#72560=CARTESIAN_POINT('Ctrl Pts',(15.4879119993482,-2.33291724011508,4.67740167194192));
#72561=CARTESIAN_POINT('Ctrl Pts',(15.4481566752091,-0.536148854634113,
5.199339732657));
#72562=CARTESIAN_POINT('Ctrl Pts',(15.4084013510701,1.06774840695936,4.84593892142932));
#72563=CARTESIAN_POINT('Ctrl Pts',(15.368646026931,2.67164566855283,4.49253811020164));
#72564=CARTESIAN_POINT('Ctrl Pts',(15.328890702792,4.08267180625871,3.26379842703124));
#72565=CARTESIAN_POINT('Ctrl Pts',(15.2891353786529,4.65317812745874,1.72370067149939));
#72566=CARTESIAN_POINT('Ctrl Pts',(15.2493800545139,5.22368444865877,0.183602915967541));
#72567=CARTESIAN_POINT('Ctrl Pts',(15.2096247303748,4.95367095335283,-1.66785291192591));
#72568=CARTESIAN_POINT('Ctrl Pts',(15.1698694062357,3.96707148128438,-2.98086473245064));
#72569=CARTESIAN_POINT('Ctrl Pts',(15.1301140820967,2.98047200921587,-4.29387655297545));
#72570=CARTESIAN_POINT('Ctrl Pts',(15.0903587579576,1.27728656038484,-5.06844436613168));
#72571=CARTESIAN_POINT('Ctrl Pts',(15.0506034338186,-0.360737596504414,
-4.94904830015389));
#72572=CARTESIAN_POINT('Ctrl Pts',(15.0108481096795,-1.99876175339348,-4.82965223417611));
#72573=CARTESIAN_POINT('Ctrl Pts',(14.9710927855405,-3.5716246183407,-3.81629228906456));
#72574=CARTESIAN_POINT('Ctrl Pts',(14.9313374614014,-4.3573958521909,-2.37409184281009));
#72575=CARTESIAN_POINT('Ctrl Pts',(14.9114878783157,-4.74972648287934,-1.6540102385425));
#72576=CARTESIAN_POINT('Ctrl Pts',(14.8916382952299,-4.94583973197741,-0.827021182931719));
#72577=CARTESIAN_POINT('Ctrl Pts',(14.8717887121442,-4.94581103525318,-1.93330908274114E-5));
#72578=CARTESIAN_POINT('Ctrl Pts',(14.7664112878559,-4.9459710090011,-0.000934506679922751));
#72579=CARTESIAN_POINT('Ctrl Pts',(14.7849223577268,-4.94726690948417,-0.772107138619626));
#72580=CARTESIAN_POINT('Ctrl Pts',(14.8034334275978,-4.77786264413242,-1.54274085058044));
#72581=CARTESIAN_POINT('Ctrl Pts',(14.8219444974687,-4.4347811370167,-2.22619128341277));
#72582=CARTESIAN_POINT('Ctrl Pts',(14.8616998216078,-3.69796167619771,-3.69400452595569));
#72583=CARTESIAN_POINT('Ctrl Pts',(14.9014551457469,-2.16007221001321,-4.75969306194599));
#72584=CARTESIAN_POINT('Ctrl Pts',(14.9412104698859,-0.526990592565549,
-4.9341151465009));
#72585=CARTESIAN_POINT('Ctrl Pts',(14.980965794025,1.10609102488183,-5.10853723105577));
#72586=CARTESIAN_POINT('Ctrl Pts',(15.020721118164,2.83436479359242,-4.3916928641756));
#72587=CARTESIAN_POINT('Ctrl Pts',(15.0604764423031,3.86456812481518,-3.11260735915159));
#72588=CARTESIAN_POINT('Ctrl Pts',(15.1002317664421,4.89477145603799,-1.8335218541275));
#72589=CARTESIAN_POINT('Ctrl Pts',(15.1399870905812,5.22690434977295,0.00780478904030796));
#72590=CARTESIAN_POINT('Ctrl Pts',(15.1797424147202,4.70852070409838,1.56621969808168));
#72591=CARTESIAN_POINT('Ctrl Pts',(15.2194977388593,4.19013705842374,3.12463460712323));
#72592=CARTESIAN_POINT('Ctrl Pts',(15.2592530629984,2.8212368733392,4.40013778203812));
#72593=CARTESIAN_POINT('Ctrl Pts',(15.2990083871374,1.23013339656155,4.80728438832633));
#72594=CARTESIAN_POINT('Ctrl Pts',(15.3387637112765,-0.360970080215911,
5.2144309946145));
#72595=CARTESIAN_POINT('Ctrl Pts',(15.3785190354155,-2.17427684868653,4.75322103227624));
#72596=CARTESIAN_POINT('Ctrl Pts',(15.4182743595546,-3.37749491472365,3.63534585212989));
#72597=CARTESIAN_POINT('Ctrl Pts',(15.4509866689883,-4.36755203398721,2.71551235578195));
#72598=CARTESIAN_POINT('Ctrl Pts',(15.4836989784221,-4.9445380670697,1.35107233960266));
#72599=CARTESIAN_POINT('Ctrl Pts',(15.5164112878559,-4.95678235276575,-0.00420182901399404));
#72600=CARTESIAN_POINT('Origin',(10.45,0.,0.));
#72601=CARTESIAN_POINT('',(16.3717887121442,-4.96090463397887,0.00227414672534738));
#72602=CARTESIAN_POINT('',(16.2664112878559,-4.95972825749042,0.00308940621307957));
#72603=CARTESIAN_POINT('',(10.45,-4.954,-6.06690024297599E-16));
#72604=CARTESIAN_POINT('Ctrl Pts',(16.3717887121442,-4.96090463397887,0.00227414672534738));
#72605=CARTESIAN_POINT('Ctrl Pts',(16.3687021848986,-4.96163172276262,0.129871883079575));
#72606=CARTESIAN_POINT('Ctrl Pts',(16.365615657653,-4.95713685536309,0.257417563448558));
#72607=CARTESIAN_POINT('Ctrl Pts',(16.3625291304074,-4.94725541875388,0.384544551902995));
#72608=CARTESIAN_POINT('Ctrl Pts',(16.3227738062683,-4.81997978367921,2.02197530519914));
#72609=CARTESIAN_POINT('Ctrl Pts',(16.2830184821293,-3.7990641238995,3.5899444330534));
#72610=CARTESIAN_POINT('Ctrl Pts',(16.2432631579902,-2.35309982455023,4.36876777896119));
#72611=CARTESIAN_POINT('Ctrl Pts',(16.2035078338512,-0.907135525201033,
5.14759112486893));
#72612=CARTESIAN_POINT('Ctrl Pts',(16.1637525097121,0.963877413717682,5.13726868883029));
#72613=CARTESIAN_POINT('Ctrl Pts',(16.1239971855731,2.4011603690595,4.34253837897213));
#72614=CARTESIAN_POINT('Ctrl Pts',(16.084241861434,3.83844332440131,3.54780806911397));
#72615=CARTESIAN_POINT('Ctrl Pts',(16.044486537295,4.84199629616623,1.96866988543629));
#72616=CARTESIAN_POINT('Ctrl Pts',(16.0047312131559,4.95119722160954,0.329934483668917));
#72617=CARTESIAN_POINT('Ctrl Pts',(15.9649758890168,5.06039814705285,-1.30880091809855));
#72618=CARTESIAN_POINT('Ctrl Pts',(15.9252205648778,4.27524702617445,-3.00713353795571));
#72619=CARTESIAN_POINT('Ctrl Pts',(15.8854652407387,2.95612137669453,-3.98554351337901));
#72620=CARTESIAN_POINT('Ctrl Pts',(15.8457099165997,1.63699572721468,-4.96395348880225));
#72621=CARTESIAN_POINT('Ctrl Pts',(15.8059545924606,-0.216104450866626,
-5.22244081979172));
#72622=CARTESIAN_POINT('Ctrl Pts',(15.7661992683216,-1.75262233542247,-4.64236207551351));
#72623=CARTESIAN_POINT('Ctrl Pts',(15.7264439441825,-3.28914021997823,-4.06228333123534));
#72624=CARTESIAN_POINT('Ctrl Pts',(15.6866886200435,-4.50907581100856,-2.64363851168958));
#72625=CARTESIAN_POINT('Ctrl Pts',(15.6469332959044,-4.85248931045004,-1.03757321802173));
#72626=CARTESIAN_POINT('Ctrl Pts',(15.6385517679843,-4.92489042642715,-0.698969989602403));
#72627=CARTESIAN_POINT('Ctrl Pts',(15.6301702400643,-4.95833156817253,-0.352036227460802));
#72628=CARTESIAN_POINT('Ctrl Pts',(15.6217887121442,-4.95510573438616,-0.00448604574660338));
#72629=CARTESIAN_POINT('Ctrl Pts',(15.5164112878559,-4.95678235276575,-0.00420182901399404));
#72630=CARTESIAN_POINT('Ctrl Pts',(15.5234543025612,-4.95941856786966,-0.295994614802925));
#72631=CARTESIAN_POINT('Ctrl Pts',(15.5304973172665,-4.93587628816053,-0.587362519495321));
#72632=CARTESIAN_POINT('Ctrl Pts',(15.5375403319717,-4.8846417999139,-0.873776773618994));
#72633=CARTESIAN_POINT('Ctrl Pts',(15.5772956561108,-4.59544125546334,-2.49048382126709));
#72634=CARTESIAN_POINT('Ctrl Pts',(15.6170509802498,-3.42391080295839,-3.94935751860888));
#72635=CARTESIAN_POINT('Ctrl Pts',(15.6568063043889,-1.90777270398753,-4.58078756039857));
#72636=CARTESIAN_POINT('Ctrl Pts',(15.6965616285279,-0.39163460501667,-5.21221760218826));
#72637=CARTESIAN_POINT('Ctrl Pts',(15.736316952667,1.46911114042006,-5.01620398842604));
#72638=CARTESIAN_POINT('Ctrl Pts',(15.7760722768061,2.82039846145153,-4.08271525852881));
#72639=CARTESIAN_POINT('Ctrl Pts',(15.8158276009451,4.17168578248299,-3.14922652863158));
#72640=CARTESIAN_POINT('Ctrl Pts',(15.8555829250842,5.0135146791091,-1.47826268259919));
#72641=CARTESIAN_POINT('Ctrl Pts',(15.8953382492232,4.95949302878925,0.163218445565945));
#72642=CARTESIAN_POINT('Ctrl Pts',(15.9350935733623,4.9054713784694,1.80469957373108));
#72643=CARTESIAN_POINT('Ctrl Pts',(15.9748488975013,3.95559918120381,3.41669798402893));
#72644=CARTESIAN_POINT('Ctrl Pts',(16.0146042216404,2.545859492355,4.25932046326266));
#72645=CARTESIAN_POINT('Ctrl Pts',(16.0543595457795,1.13611980350619,5.10194294249639));
#72646=CARTESIAN_POINT('Ctrl Pts',(16.0941148699185,-0.733487376925646,
5.17518949066586));
#72647=CARTESIAN_POINT('Ctrl Pts',(16.1338701940576,-2.2048286566811,4.44544058089409));
#72648=CARTESIAN_POINT('Ctrl Pts',(16.1736255181966,-3.67616993643647,3.71569167112235));
#72649=CARTESIAN_POINT('Ctrl Pts',(16.2133808423357,-4.74924531551546,2.18294730340928));
#72650=CARTESIAN_POINT('Ctrl Pts',(16.2531361664747,-4.93152255247316,0.550723776525695));
#72651=CARTESIAN_POINT('Ctrl Pts',(16.2575612069351,-4.95181126011202,0.36904609427131));
#72652=CARTESIAN_POINT('Ctrl Pts',(16.2619862473955,-4.96106367538195,0.18613594302839));
#72653=CARTESIAN_POINT('Ctrl Pts',(16.2664112878559,-4.95972825749042,0.00308940621307957));
#72654=CARTESIAN_POINT('Origin',(10.45,0.,0.));
#72655=CARTESIAN_POINT('',(17.1217887121442,-4.94814833252334,0.00329320459974858));
#72656=CARTESIAN_POINT('',(17.0164112878559,-4.94714433343639,0.00258591176320991));
#72657=CARTESIAN_POINT('',(10.45,-4.954,-6.06690024297599E-16));
#72658=CARTESIAN_POINT('Ctrl Pts',(17.1217887121442,-4.94814833252334,0.00329320459974858));
#72659=CARTESIAN_POINT('Ctrl Pts',(17.1072341297329,-4.95183295583228,0.608971087556108));
#72660=CARTESIAN_POINT('Ctrl Pts',(17.0926795473216,-4.84894916378528,1.2134405946199));
#72661=CARTESIAN_POINT('Ctrl Pts',(17.0781249649104,-4.6338760321099,1.7749376354749));
#72662=CARTESIAN_POINT('Ctrl Pts',(17.0383696407713,-4.04641142324979,3.3086468297032));
#72663=CARTESIAN_POINT('Ctrl Pts',(16.9986143166323,-2.62191360277959,4.52174283982081));
#72664=CARTESIAN_POINT('Ctrl Pts',(16.9588589924932,-1.01421464822929,4.85742517575979));
#72665=CARTESIAN_POINT('Ctrl Pts',(16.9191036683542,0.593484306321018,5.19310751169876));
#72666=CARTESIAN_POINT('Ctrl Pts',(16.8793483442151,2.38438439495152,4.65137617345912));
#72667=CARTESIAN_POINT('Ctrl Pts',(16.839593020076,3.53647809418883,3.4808811212264));
#72668=CARTESIAN_POINT('Ctrl Pts',(16.799837695937,4.68857179342601,2.31038606899382));
#72669=CARTESIAN_POINT('Ctrl Pts',(16.7600823717979,5.20185910327026,0.511127302768274));
#72670=CARTESIAN_POINT('Ctrl Pts',(16.7203270476589,4.84074562452872,-1.09105109385122));
#72671=CARTESIAN_POINT('Ctrl Pts',(16.6805717235198,4.47963214578711,-2.69322949047098));
#72672=CARTESIAN_POINT('Ctrl Pts',(16.6408163993808,3.24411787845962,-4.09832751748447));
#72673=CARTESIAN_POINT('Ctrl Pts',(16.6010610752417,1.70129309717905,-4.66141743338641));
#72674=CARTESIAN_POINT('Ctrl Pts',(16.5613057511027,0.158468315898662,-5.22450734928829));
#72675=CARTESIAN_POINT('Ctrl Pts',(16.5215504269636,-1.69166697933467,-4.9455891540786));
#72676=CARTESIAN_POINT('Ctrl Pts',(16.4817951028245,-2.99991682176645,-3.9526838671048));
#72677=CARTESIAN_POINT('Ctrl Pts',(16.4451263059311,-4.206596651372,-3.03686584546993));
#72678=CARTESIAN_POINT('Ctrl Pts',(16.4084575090376,-4.95226661823711,-1.51362223329568));
#72679=CARTESIAN_POINT('Ctrl Pts',(16.3717887121442,-4.96090463397887,0.00227414672534738));
#72680=CARTESIAN_POINT('Ctrl Pts',(16.2664112878559,-4.95972825749042,0.00308940621307957));
#72681=CARTESIAN_POINT('Ctrl Pts',(16.3017415715346,-4.94906605149262,-1.45838560853021));
#72682=CARTESIAN_POINT('Ctrl Pts',(16.3370718552132,-4.26346123593968,-2.92855479447191));
#72683=CARTESIAN_POINT('Ctrl Pts',(16.3724021388919,-3.13116475392864,-3.84954784972692));
#72684=CARTESIAN_POINT('Ctrl Pts',(16.4121574630309,-1.85705062359026,-4.8858932630411));
#72685=CARTESIAN_POINT('Ctrl Pts',(16.45191278717,-0.0173432680774013,-5.22688140361534));
#72686=CARTESIAN_POINT('Ctrl Pts',(16.491668111309,1.54354767925271,-4.7160016884492));
#72687=CARTESIAN_POINT('Ctrl Pts',(16.5314234354481,3.10443862658291,-4.20512197328303));
#72688=CARTESIAN_POINT('Ctrl Pts',(16.5711787595872,4.38651316573016,-2.84237440237626));
#72689=CARTESIAN_POINT('Ctrl Pts',(16.6109340837262,4.8013102633162,-1.25324822719073));
#72690=CARTESIAN_POINT('Ctrl Pts',(16.6506894078653,5.21610736090221,0.335877947994718));
#72691=CARTESIAN_POINT('Ctrl Pts',(16.6904447320043,4.76362701692717,2.15138272745901));
#72692=CARTESIAN_POINT('Ctrl Pts',(16.7302000561434,3.65155376350569,3.35996524919672));
#72693=CARTESIAN_POINT('Ctrl Pts',(16.7699553802824,2.53948051008421,4.56854777093442));
#72694=CARTESIAN_POINT('Ctrl Pts',(16.8097107044215,0.76781434721649,5.17020803494558));
#72695=CARTESIAN_POINT('Ctrl Pts',(16.8494660285605,-0.850265405823871,
4.88878922671466));
#72696=CARTESIAN_POINT('Ctrl Pts',(16.8892213526996,-2.46834515886432,4.60737041848372));
#72697=CARTESIAN_POINT('Ctrl Pts',(16.9289766768386,-3.93283850207731,3.44287253801038));
#72698=CARTESIAN_POINT('Ctrl Pts',(16.9687320009777,-4.57155576176729,1.9297899576468));
#72699=CARTESIAN_POINT('Ctrl Pts',(16.9846250966038,-4.82689752305581,1.32490075951781));
#72700=CARTESIAN_POINT('Ctrl Pts',(17.0005181922298,-4.95026518831848,0.664301361524176));
#72701=CARTESIAN_POINT('Ctrl Pts',(17.0164112878559,-4.94714433343639,0.00258591176320991));
#72702=CARTESIAN_POINT('Origin',(10.45,0.,0.));
#72703=CARTESIAN_POINT('',(17.8717887121442,-4.94888348879255,-0.00366329764976359));
#72704=CARTESIAN_POINT('',(17.7664112878558,-4.95024685397467,-0.00414268332982216));
#72705=CARTESIAN_POINT('',(10.45,-4.954,-6.06690024297599E-16));
#72706=CARTESIAN_POINT('Ctrl Pts',(17.8717887121442,-4.94888348879255,-0.00366329764976359));
#72707=CARTESIAN_POINT('Ctrl Pts',(17.8457660745672,-4.94148610429648,1.07884500791139));
#72708=CARTESIAN_POINT('Ctrl Pts',(17.8197434369903,-4.59224319699392,2.16569540170491));
#72709=CARTESIAN_POINT('Ctrl Pts',(17.7937207994134,-3.93820475500025,3.01889946809781));
#72710=CARTESIAN_POINT('Ctrl Pts',(17.7539654752743,-2.93901663719373,4.32235704867263));
#72711=CARTESIAN_POINT('Ctrl Pts',(17.7142101511353,-1.22845684021116,5.08050027474164));
#72712=CARTESIAN_POINT('Ctrl Pts',(17.6744548269962,0.408342605748216,4.94534801678492));
#72713=CARTESIAN_POINT('Ctrl Pts',(17.6346995028571,2.0451420517074,4.81019575882822));
#72714=CARTESIAN_POINT('Ctrl Pts',(17.5949441787181,3.60818114664354,3.78174801684578));
#72715=CARTESIAN_POINT('Ctrl Pts',(17.555188854579,4.3800385761698,2.3320533360222));
#72716=CARTESIAN_POINT('Ctrl Pts',(17.51543353044,5.1518960056961,0.882358655198545));
#72717=CARTESIAN_POINT('Ctrl Pts',(17.4756782063009,5.13257176981269,-0.988582964466396));
#72718=CARTESIAN_POINT('Ctrl Pts',(17.4359228821619,4.33093552427665,-2.42202563474181));
#72719=CARTESIAN_POINT('Ctrl Pts',(17.3961675580228,3.52929927874056,-3.8554683050173));
#72720=CARTESIAN_POINT('Ctrl Pts',(17.3564122338838,1.94535102355181,-4.85141202590312));
#72721=CARTESIAN_POINT('Ctrl Pts',(17.3166569097447,0.30610919531848,-4.95272731445305));
#72722=CARTESIAN_POINT('Ctrl Pts',(17.2769015856056,-1.33313263291476,-5.05404260300297));
#72723=CARTESIAN_POINT('Ctrl Pts',(17.2371462614666,-3.02766803419248,-4.26072945921708));
#72724=CARTESIAN_POINT('Ctrl Pts',(17.1973909373275,-3.9997200362063,-2.93691169815466));
#72725=CARTESIAN_POINT('Ctrl Pts',(17.1721901955998,-4.61589993108146,-2.09774888880353));
#72726=CARTESIAN_POINT('Ctrl Pts',(17.146989453872,-4.94176853832871,-1.04541650532658));
#72727=CARTESIAN_POINT('Ctrl Pts',(17.1217887121442,-4.94814833252334,0.00329320459974858));
#72728=CARTESIAN_POINT('Ctrl Pts',(17.0164112878559,-4.94714433343639,0.00258591176320991));
#72729=CARTESIAN_POINT('Ctrl Pts',(17.0402735163689,-4.94245861618504,-0.990927601544862));
#72730=CARTESIAN_POINT('Ctrl Pts',(17.0641357448819,-4.65263422909462,-1.98695699151951));
#72731=CARTESIAN_POINT('Ctrl Pts',(17.0879979733949,-4.09623765919655,-2.8007228357983));
#72732=CARTESIAN_POINT('Ctrl Pts',(17.1277532975339,-3.16926112076872,-4.15648576862615));
#72733=CARTESIAN_POINT('Ctrl Pts',(17.167508621673,-1.50236686774581,-5.00634435402793));
#72734=CARTESIAN_POINT('Ctrl Pts',(17.207263945812,0.139355173573051,-4.96022091233652));
#72735=CARTESIAN_POINT('Ctrl Pts',(17.2470192699511,1.78107721489191,-4.9140974706451));
#72736=CARTESIAN_POINT('Ctrl Pts',(17.2867745940901,3.39762704450684,-3.97199200186048));
#72737=CARTESIAN_POINT('Ctrl Pts',(17.3265299182292,4.24702238744387,-2.56632270070089));
#72738=CARTESIAN_POINT('Ctrl Pts',(17.3662852423683,5.0964177303809,-1.1606533995413));
#72739=CARTESIAN_POINT('Ctrl Pts',(17.4060405665073,5.17865858664018,0.708579733993037));
#72740=CARTESIAN_POINT('Ctrl Pts',(17.4457958906464,4.45599712036464,2.18341499190698));
#72741=CARTESIAN_POINT('Ctrl Pts',(17.4855512147854,3.73333565408914,3.65825024982084));
#72742=CARTESIAN_POINT('Ctrl Pts',(17.5253065389245,2.20577186527881,4.73868763211418));
#72743=CARTESIAN_POINT('Ctrl Pts',(17.5650618630635,0.57444421216427,4.92881580206575));
#72744=CARTESIAN_POINT('Ctrl Pts',(17.6048171872026,-1.05688344095027,5.11894397201733));
#72745=CARTESIAN_POINT('Ctrl Pts',(17.6445725113416,-2.79197495836912,4.41876292962717));
#72746=CARTESIAN_POINT('Ctrl Pts',(17.6843278354807,-3.83443846413696,3.14964966755497));
#72747=CARTESIAN_POINT('Ctrl Pts',(17.7116889862724,-4.55190214463446,2.27619686375266));
#72748=CARTESIAN_POINT('Ctrl Pts',(17.7390501370641,-4.94128702106912,1.13325654416073));
#72749=CARTESIAN_POINT('Ctrl Pts',(17.7664112878558,-4.95024685397467,-0.00414268332982216));
#72750=CARTESIAN_POINT('Origin',(10.45,0.,0.));
#72751=CARTESIAN_POINT('',(18.6217887121442,-4.96146530959486,-0.00170939900883904));
#72752=CARTESIAN_POINT('',(18.5164112878559,-4.96205143092805,-0.000716217698562718));
#72753=CARTESIAN_POINT('',(10.45,-4.954,-6.06690024297599E-16));
#72754=CARTESIAN_POINT('Ctrl Pts',(18.6217887121442,-4.96146530959486,-0.00170939900883904));
#72755=CARTESIAN_POINT('Ctrl Pts',(18.5842980194016,-4.95455118100335,1.54769955531428));
#72756=CARTESIAN_POINT('Ctrl Pts',(18.546807326659,-4.17043746833274,3.103141179268));
#72757=CARTESIAN_POINT('Ctrl Pts',(18.5093166339163,-2.91763403509206,4.01380397230112));
#72758=CARTESIAN_POINT('Ctrl Pts',(18.4695613097773,-1.58915480658206,4.979475499551));
#72759=CARTESIAN_POINT('Ctrl Pts',(18.4298059856382,0.266346847597793,5.22011959697153));
#72760=CARTESIAN_POINT('Ctrl Pts',(18.3900506614992,1.79721184873288,4.62528272233839));
#72761=CARTESIAN_POINT('Ctrl Pts',(18.3502953373601,3.32807684986788,4.03044584770528));
#72762=CARTESIAN_POINT('Ctrl Pts',(18.3105400132211,4.53430519795815,2.60012800101859));
#72763=CARTESIAN_POINT('Ctrl Pts',(18.270784689082,4.86224859991823,0.990832601089107));
#72764=CARTESIAN_POINT('Ctrl Pts',(18.231029364943,5.19019200187832,-0.618462798840377));
#72765=CARTESIAN_POINT('Ctrl Pts',(18.1912740408039,4.63985045770823,-2.40673575201266));
#72766=CARTESIAN_POINT('Ctrl Pts',(18.1515187166649,3.46382593703186,-3.5531845672204));
#72767=CARTESIAN_POINT('Ctrl Pts',(18.1117633925258,2.28780141635541,-4.69963338242821));
#72768=CARTESIAN_POINT('Ctrl Pts',(18.0720080683867,0.486093919172618,-5.20425805967141));
#72769=CARTESIAN_POINT('Ctrl Pts',(18.0322527442477,-1.11432852476172,-4.83544027258017));
#72770=CARTESIAN_POINT('Ctrl Pts',(17.9924974201086,-2.71475096869597,-4.46662248548895));
#72771=CARTESIAN_POINT('Ctrl Pts',(17.9527420959696,-4.11388835938179,-3.22436223406338));
#72772=CARTESIAN_POINT('Ctrl Pts',(17.9129867718305,-4.66954883540947,-1.67884614081038));
#72773=CARTESIAN_POINT('Ctrl Pts',(17.8992540852684,-4.8614907027567,-1.14497832448687));
#72774=CARTESIAN_POINT('Ctrl Pts',(17.8855213987063,-4.95278724229807,-0.574925423451077));
#72775=CARTESIAN_POINT('Ctrl Pts',(17.8717887121442,-4.94888348879255,-0.00366329764976359));
#72776=CARTESIAN_POINT('Ctrl Pts',(17.7664112878558,-4.95024685397467,-0.00414268332982216));
#72777=CARTESIAN_POINT('Ctrl Pts',(17.7788054612032,-4.95430551813832,-0.519366743091031));
#72778=CARTESIAN_POINT('Ctrl Pts',(17.7911996345505,-4.88030293042791,-1.03345379940426));
#72779=CARTESIAN_POINT('Ctrl Pts',(17.8035938078979,-4.72337350536271,-1.52083992991365));
#72780=CARTESIAN_POINT('Ctrl Pts',(17.8433491320369,-4.22000954670368,-3.08417078355551));
#72781=CARTESIAN_POINT('Ctrl Pts',(17.883104456176,-2.86344613526889,-4.37278700908486));
#72782=CARTESIAN_POINT('Ctrl Pts',(17.922859780315,-1.2763340472501,-4.79522499611982));
#72783=CARTESIAN_POINT('Ctrl Pts',(17.9626151044541,0.310778040768601,-5.21766298315475));
#72784=CARTESIAN_POINT('Ctrl Pts',(18.0023704285931,2.12843880537138,-4.77392273169524));
#72785=CARTESIAN_POINT('Ctrl Pts',(18.0421257527322,3.34235780617494,-3.66767714760767));
#72786=CARTESIAN_POINT('Ctrl Pts',(18.0818810768712,4.55627680697864,-2.56143156351998));
#72787=CARTESIAN_POINT('Ctrl Pts',(18.1216364010103,5.16645404398317,-0.792680646804141));
#72788=CARTESIAN_POINT('Ctrl Pts',(18.1613917251494,4.89282348633957,0.826734355827807));
#72789=CARTESIAN_POINT('Ctrl Pts',(18.2011470492884,4.61919292869599,2.44614935845966));
#72790=CARTESIAN_POINT('Ctrl Pts',(18.2409023734275,3.46175457640439,3.91622844700751));
#72791=CARTESIAN_POINT('Ctrl Pts',(18.2806576975665,1.95176253994259,4.56221813937683));
#72792=CARTESIAN_POINT('Ctrl Pts',(18.3204130217056,0.441770503480876,5.20820783174611));
#72793=CARTESIAN_POINT('Ctrl Pts',(18.3601683458446,-1.42077521715118,5.03010812793685));
#72794=CARTESIAN_POINT('Ctrl Pts',(18.3999236699837,-2.78098237816365,4.10966523891245));
#72795=CARTESIAN_POINT('Ctrl Pts',(18.4387528759411,-4.10950290072166,3.21066448155629));
#72796=CARTESIAN_POINT('Ctrl Pts',(18.4775820818985,-4.95881666157094,1.60350412336648));
#72797=CARTESIAN_POINT('Ctrl Pts',(18.5164112878559,-4.96205143092805,-0.000716217698562718));
#72798=CARTESIAN_POINT('Origin',(10.45,0.,0.));
#72799=CARTESIAN_POINT('',(19.3717887121442,-4.95406386564724,0.00456011872589132));
#72800=CARTESIAN_POINT('',(19.2664112878559,-4.9523954629479,0.00451814608447948));
#72801=CARTESIAN_POINT('',(10.45,-4.954,-6.06690024297599E-16));
#72802=CARTESIAN_POINT('Ctrl Pts',(19.3717887121442,-4.95406386564724,0.00456011872589132));
#72803=CARTESIAN_POINT('Ctrl Pts',(19.3625852883749,-4.95759204267437,0.386396835530268));
#72804=CARTESIAN_POINT('Ctrl Pts',(19.3533818646057,-4.91718650431454,0.767494781265623));
#72805=CARTESIAN_POINT('Ctrl Pts',(19.3441784408365,-4.83002298839371,1.13758016085729));
#72806=CARTESIAN_POINT('Ctrl Pts',(19.3044231166974,-4.45350943045892,2.73620960504211));
#72807=CARTESIAN_POINT('Ctrl Pts',(19.2646677925584,-3.20453195115239,4.12935397174361));
#72808=CARTESIAN_POINT('Ctrl Pts',(19.2249124684193,-1.65636032200206,4.67757214529986));
#72809=CARTESIAN_POINT('Ctrl Pts',(19.1851571442803,-0.108188692851636,
5.22579031885614));
#72810=CARTESIAN_POINT('Ctrl Pts',(19.1454018201412,1.73917708614262,4.92908229926707));
#72811=CARTESIAN_POINT('Ctrl Pts',(19.1056464960022,3.03781223202891,3.92363448013744));
#72812=CARTESIAN_POINT('Ctrl Pts',(19.0658911718631,4.33644737791506,2.91818666100792));
#72813=CARTESIAN_POINT('Ctrl Pts',(19.0261358477241,5.08635189069337,1.203999042338));
#72814=CARTESIAN_POINT('Ctrl Pts',(18.986380523585,4.94332613840025,-0.432131207154393));
#72815=CARTESIAN_POINT('Ctrl Pts',(18.946625199446,4.80030038610712,-2.06826145664697));
#72816=CARTESIAN_POINT('Ctrl Pts',(18.9068698753069,3.76434436874231,-3.626334336962));
#72817=CARTESIAN_POINT('Ctrl Pts',(18.8671145511678,2.31095286441626,-4.39120798291701));
#72818=CARTESIAN_POINT('Ctrl Pts',(18.8273592270288,0.8575613600903,-5.15608162887199));
#72819=CARTESIAN_POINT('Ctrl Pts',(18.7876039028897,-1.01326563119685,-5.12775604046705));
#72820=CARTESIAN_POINT('Ctrl Pts',(18.7478485787507,-2.44283483464014,-4.31923241577211));
#72821=CARTESIAN_POINT('Ctrl Pts',(18.7080932546116,-3.87240403808351,-3.51070879107711));
#72822=CARTESIAN_POINT('Ctrl Pts',(18.6683379304726,-4.86071545368295,-1.92198713009198));
#72823=CARTESIAN_POINT('Ctrl Pts',(18.6285826063335,-4.95414276006255,-0.282276821059833));
#72824=CARTESIAN_POINT('Ctrl Pts',(18.6263179749371,-4.95946477455733,-0.188871987183443));
#72825=CARTESIAN_POINT('Ctrl Pts',(18.6240533435406,-4.96188295865765,-0.0953016990494065));
#72826=CARTESIAN_POINT('Ctrl Pts',(18.6217887121442,-4.96146530959486,-0.00170939900883904));
#72827=CARTESIAN_POINT('Ctrl Pts',(18.5164112878559,-4.96205143092805,-0.000716217698562718));
#72828=CARTESIAN_POINT('Ctrl Pts',(18.5173374060375,-4.96212858364445,-0.0389785923369267));
#72829=CARTESIAN_POINT('Ctrl Pts',(18.5182635242192,-4.96172442433453,-0.0772392944770803));
#72830=CARTESIAN_POINT('Ctrl Pts',(18.5191896424009,-4.96083397518572,-0.115488675744613));
#72831=CARTESIAN_POINT('Ctrl Pts',(18.5589449665399,-4.92260980980206,-1.75741362713735));
#72832=CARTESIAN_POINT('Ctrl Pts',(18.598700290679,-3.9882928776417,-3.37847745568325));
#72833=CARTESIAN_POINT('Ctrl Pts',(18.638455614818,-2.58672650303079,-4.23462600026262));
#72834=CARTESIAN_POINT('Ctrl Pts',(18.6782109389571,-1.18516012841989,-5.090774544842));
#72835=CARTESIAN_POINT('Ctrl Pts',(18.7179662630961,0.68365568864165,-5.18200780545489));
#72836=CARTESIAN_POINT('Ctrl Pts',(18.7577215872352,2.16195078478016,-4.46645051106252));
#72837=CARTESIAN_POINT('Ctrl Pts',(18.7974769113742,3.64024588091884,-3.75089321667006));
#72838=CARTESIAN_POINT('Ctrl Pts',(18.8372322355133,4.72802025613451,-2.22854536727209));
#72839=CARTESIAN_POINT('Ctrl Pts',(18.8769875596524,4.92599495793533,-0.598151350393721));
#72840=CARTESIAN_POINT('Ctrl Pts',(18.9167428837914,5.12396965973613,1.03224266648446));
#72841=CARTESIAN_POINT('Ctrl Pts',(18.9564982079305,4.43214468812251,2.77068285084289));
#72842=CARTESIAN_POINT('Ctrl Pts',(18.9962535320695,3.16806167213509,3.81924031780284));
#72843=CARTESIAN_POINT('Ctrl Pts',(19.0360088562086,1.90397865614767,4.86779778476279));
#72844=CARTESIAN_POINT('Ctrl Pts',(19.0757641803476,0.0676375957864397,
5.22647253432405));
#72845=CARTESIAN_POINT('Ctrl Pts',(19.1155195044867,-1.49809697571037,4.73063598419384));
#72846=CARTESIAN_POINT('Ctrl Pts',(19.1552748286257,-3.06383154720717,4.23479943406362));
#72847=CARTESIAN_POINT('Ctrl Pts',(19.1950301527648,-4.35895962983965,2.8844515842419));
#72848=CARTESIAN_POINT('Ctrl Pts',(19.2347854769038,-4.78902872760088,1.29939032234185));
#72849=CARTESIAN_POINT('Ctrl Pts',(19.2453274138878,-4.90307034153692,0.879078922532937));
#72850=CARTESIAN_POINT('Ctrl Pts',(19.2558693508718,-4.95628501739502,0.442263563534826));
#72851=CARTESIAN_POINT('Ctrl Pts',(19.2664112878559,-4.9523954629479,0.00451814608447948));
#72852=CARTESIAN_POINT('Origin',(10.45,0.,0.));
#72853=CARTESIAN_POINT('',(20.1217887121442,-4.94586503871743,-0.000545303237105832));
#72854=CARTESIAN_POINT('',(20.0164112878559,-4.94619904628785,-0.00144379608614997));
#72855=CARTESIAN_POINT('',(10.45,-4.954,-6.06690024297599E-16));
#72856=CARTESIAN_POINT('Ctrl Pts',(20.1217887121442,-4.94586503871743,-0.000545303237105832));
#72857=CARTESIAN_POINT('Ctrl Pts',(20.1011172332093,-4.9450216042098,0.8606761091776));
#72858=CARTESIAN_POINT('Ctrl Pts',(20.0804457542744,-4.73140686367877,1.7222891587838));
#72859=CARTESIAN_POINT('Ctrl Pts',(20.0597742753395,-4.30742932436548,2.46358748705707));
#72860=CARTESIAN_POINT('Ctrl Pts',(20.0200189512004,-3.49203703646159,3.88925013156671));
#72861=CARTESIAN_POINT('Ctrl Pts',(19.9802636270614,-1.89857874589106,4.86990636414725));
#72862=CARTESIAN_POINT('Ctrl Pts',(19.9405083029223,-0.258437912571716,
4.9554435256729));
#72863=CARTESIAN_POINT('Ctrl Pts',(19.9007529787833,1.38170292074772,5.04098068719854));
#72864=CARTESIAN_POINT('Ctrl Pts',(19.8609976546442,3.06852629681598,4.23139877766919));
#72865=CARTESIAN_POINT('Ctrl Pts',(19.8212423305052,4.0277949956444,2.8982888337517));
#72866=CARTESIAN_POINT('Ctrl Pts',(19.7814870063661,4.98706369447276,1.56517888983429));
#72867=CARTESIAN_POINT('Ctrl Pts',(19.741731682227,5.21877771606137,-0.291459088471185));
#72868=CARTESIAN_POINT('Ctrl Pts',(19.701976358088,4.61658234511971,-1.81944445958564));
#72869=CARTESIAN_POINT('Ctrl Pts',(19.6622210339489,4.01438697417804,-3.3474298307001));
#72870=CARTESIAN_POINT('Ctrl Pts',(19.6224657098099,2.5782822107061,-4.54676259462353));
#72871=CARTESIAN_POINT('Ctrl Pts',(19.5827103856708,0.967427617855369,-4.86695947127142));
#72872=CARTESIAN_POINT('Ctrl Pts',(19.5429550615318,-0.64342697499545,-5.18715634791932));
#72873=CARTESIAN_POINT('Ctrl Pts',(19.5031997373927,-2.42903139722507,-4.62821733729157));
#72874=CARTESIAN_POINT('Ctrl Pts',(19.4634444132537,-3.56980879005835,-3.44669057114357));
#72875=CARTESIAN_POINT('Ctrl Pts',(19.4328925128838,-4.44649431595391,-2.53868921974274));
#72876=CARTESIAN_POINT('Ctrl Pts',(19.402340612514,-4.94235164683355,-1.26299395917723));
#72877=CARTESIAN_POINT('Ctrl Pts',(19.3717887121442,-4.95406386564724,0.00456011872589132));
#72878=CARTESIAN_POINT('Ctrl Pts',(19.2664112878559,-4.9523954629479,0.00451814608447948));
#72879=CARTESIAN_POINT('Ctrl Pts',(19.2956246750109,-4.9416168878059,-1.20854415686073));
#72880=CARTESIAN_POINT('Ctrl Pts',(19.324838062166,-4.49231642076917,-2.42874868009104));
#72881=CARTESIAN_POINT('Ctrl Pts',(19.354051449321,-3.68371563120667,-3.32467299324095));
#72882=CARTESIAN_POINT('Ctrl Pts',(19.39380677346,-2.58332332416117,-4.54390037294535));
#72883=CARTESIAN_POINT('Ctrl Pts',(19.4335620975991,-0.817528597180191,
-5.16258045837549));
#72884=CARTESIAN_POINT('Ctrl Pts',(19.4733174217382,0.803184168333579,-4.89674448540256));
#72885=CARTESIAN_POINT('Ctrl Pts',(19.5130727458772,2.42389693384726,-4.63090851242965));
#72886=CARTESIAN_POINT('Ctrl Pts',(19.5528280700163,3.89952773789364,-3.4805564810538));
#72887=CARTESIAN_POINT('Ctrl Pts',(19.5925833941553,4.55277490937709,-1.97368994224741));
#72888=CARTESIAN_POINT('Ctrl Pts',(19.6323387182944,5.20602208086054,-0.46682340344102));
#72889=CARTESIAN_POINT('Ctrl Pts',(19.6720940424334,5.03688561978088,1.39655764279609));
#72890=CARTESIAN_POINT('Ctrl Pts',(19.7118493665725,4.12299768685097,2.76117754550548));
#72891=CARTESIAN_POINT('Ctrl Pts',(19.7516046907115,3.20910975392107,4.12579744821486));
#72892=CARTESIAN_POINT('Ctrl Pts',(19.7913600148506,1.55047034914099,4.99165620739672));
#72893=CARTESIAN_POINT('Ctrl Pts',(19.8311153389897,-0.091619504549001,
4.96133220314547));
#72894=CARTESIAN_POINT('Ctrl Pts',(19.8708706631287,-1.73370935823909,4.93100819889422));
#72895=CARTESIAN_POINT('Ctrl Pts',(19.9106259872678,-3.35924966083898,4.00450143120977));
#72896=CARTESIAN_POINT('Ctrl Pts',(19.9503813114068,-4.22213158867454,2.60707042703084));
#72897=CARTESIAN_POINT('Ctrl Pts',(19.9723913035565,-4.69985438100614,1.83340184055148));
#72898=CARTESIAN_POINT('Ctrl Pts',(19.9944012957062,-4.94381231674025,0.915388760842907));
#72899=CARTESIAN_POINT('Ctrl Pts',(20.0164112878559,-4.94619904628785,-0.00144379608614997));
#72900=CARTESIAN_POINT('Origin',(10.45,0.,0.));
#72901=CARTESIAN_POINT('',(20.8717887121442,-4.95607142653195,-0.00434810948939879));
#72902=CARTESIAN_POINT('',(20.7664112878559,-4.95770599871256,-0.00394983957152954));
#72903=CARTESIAN_POINT('',(10.45,-4.954,-6.06690024297599E-16));
#72904=CARTESIAN_POINT('Ctrl Pts',(20.8717887121442,-4.95607142653195,-0.00434810948939879));
#72905=CARTESIAN_POINT('Ctrl Pts',(20.8396491780436,-4.94383012710083,1.32768880656287));
#72906=CARTESIAN_POINT('Ctrl Pts',(20.807509643943,-4.38908727589373,2.66871408325221));
#72907=CARTESIAN_POINT('Ctrl Pts',(20.7753701098425,-3.42947542021679,3.58635037787954));
#72908=CARTESIAN_POINT('Ctrl Pts',(20.7356147857034,-2.2424737589373,4.7214299412772));
#72909=CARTESIAN_POINT('Ctrl Pts',(20.6958594615644,-0.43599397497383,5.20869451049855));
#72910=CARTESIAN_POINT('Ctrl Pts',(20.6561041374253,1.16080546390229,4.82449389737022));
#72911=CARTESIAN_POINT('Ctrl Pts',(20.6163488132863,2.7576049027785,4.44029328424187));
#72912=CARTESIAN_POINT('Ctrl Pts',(20.5765934891472,4.14472399656744,3.1846274887637));
#72913=CARTESIAN_POINT('Ctrl Pts',(20.5368381650081,4.68548717733165,1.63383616126237));
#72914=CARTESIAN_POINT('Ctrl Pts',(20.4970828408691,5.22625035809582,0.0830448337611306));
#72915=CARTESIAN_POINT('Ctrl Pts',(20.45732751673,4.92065762583549,-1.76287202576309));
#72916=CARTESIAN_POINT('Ctrl Pts',(20.417572192591,3.90897337979402,-3.05665467576067));
#72917=CARTESIAN_POINT('Ctrl Pts',(20.377816868452,2.89728913375249,-4.35043732575833));
#72918=CARTESIAN_POINT('Ctrl Pts',(20.3380615443129,1.17951337392963,-5.09208576622906));
#72919=CARTESIAN_POINT('Ctrl Pts',(20.2983062201738,-0.455909805456886,
-4.94118983040281));
#72920=CARTESIAN_POINT('Ctrl Pts',(20.2585508960348,-2.0913329848434,-4.79029389457655));
#72921=CARTESIAN_POINT('Ctrl Pts',(20.2187955718957,-3.64440358379368,-3.74685358245331));
#72922=CARTESIAN_POINT('Ctrl Pts',(20.1790402477566,-4.40227574065016,-2.28979889817227));
#72923=CARTESIAN_POINT('Ctrl Pts',(20.1599564025525,-4.76607896045046,-1.59036538452368));
#72924=CARTESIAN_POINT('Ctrl Pts',(20.1408725573483,-4.9466436948375,-0.795622238602891));
#72925=CARTESIAN_POINT('Ctrl Pts',(20.1217887121442,-4.94586503871743,-0.000545303237105832));
#72926=CARTESIAN_POINT('Ctrl Pts',(20.0164112878559,-4.94619904628785,-0.00144379608614997));
#72927=CARTESIAN_POINT('Ctrl Pts',(20.0341566198452,-4.94812332267574,-0.740630706773701));
#72928=CARTESIAN_POINT('Ctrl Pts',(20.0519019518346,-4.79302084621013,-1.47905025092917));
#72929=CARTESIAN_POINT('Ctrl Pts',(20.069647283824,-4.47680051100919,-2.14043653216113));
#72930=CARTESIAN_POINT('Ctrl Pts',(20.109402607963,-3.76836395243713,-3.62215724650104));
#72931=CARTESIAN_POINT('Ctrl Pts',(20.1491579321021,-2.25126728222178,-4.71724343450763));
#72932=CARTESIAN_POINT('Ctrl Pts',(20.1889132562412,-0.621844642435137,
-4.9230600853795));
#72933=CARTESIAN_POINT('Ctrl Pts',(20.2286685803802,1.00757799735169,-5.1288767362514));
#72934=CARTESIAN_POINT('Ctrl Pts',(20.2684239045193,2.74932660670983,-4.44542384998839));
#72935=CARTESIAN_POINT('Ctrl Pts',(20.3081792286583,3.80395376253568,-3.18640034146257));
#72936=CARTESIAN_POINT('Ctrl Pts',(20.3479345527974,4.85858091836135,-1.92737683293696));
#72937=CARTESIAN_POINT('Ctrl Pts',(20.3876898769364,5.226086620655,-0.0927827021487665));
#72938=CARTESIAN_POINT('Ctrl Pts',(20.4274452010755,4.73778895682836,1.4753193431042));
#72939=CARTESIAN_POINT('Ctrl Pts',(20.4672005252145,4.24949129300169,3.04342138835725));
#72940=CARTESIAN_POINT('Ctrl Pts',(20.5069558493536,2.90539026305463,4.34503134807505));
#72941=CARTESIAN_POINT('Ctrl Pts',(20.5467111734926,1.32241651875205,4.78272160119255));
#72942=CARTESIAN_POINT('Ctrl Pts',(20.5864664976317,-0.260557225550523,
5.22041185431005));
#72943=CARTESIAN_POINT('Ctrl Pts',(20.6262218217707,-2.08240368420862,4.79418240082726));
#72944=CARTESIAN_POINT('Ctrl Pts',(20.6659771459098,-3.30691121976839,3.69966884303881));
#72945=CARTESIAN_POINT('Ctrl Pts',(20.6994551932251,-4.33807175238249,2.77797652965785));
#72946=CARTESIAN_POINT('Ctrl Pts',(20.7329332405405,-4.94563764625562,1.38237978314307));
#72947=CARTESIAN_POINT('Ctrl Pts',(20.7664112878559,-4.95770599871256,-0.00394983957152954));
#72948=CARTESIAN_POINT('Origin',(10.45,0.,0.));
#72949=CARTESIAN_POINT('',(21.6217887121442,-4.96026724855995,0.00275821796382324));
#72950=CARTESIAN_POINT('',(21.5164112878558,-4.95893736719177,0.00348609211932242));
#72951=CARTESIAN_POINT('',(10.45,-4.954,-6.06690024297599E-16));
#72952=CARTESIAN_POINT('Ctrl Pts',(21.6217887121442,-4.96026724855995,0.00275821796382324));
#72953=CARTESIAN_POINT('Ctrl Pts',(21.617936447017,-4.96133041918326,0.162065765024171));
#72954=CARTESIAN_POINT('Ctrl Pts',(21.6140841818898,-4.9543231377804,0.321278587713524));
#72955=CARTESIAN_POINT('Ctrl Pts',(21.6102319167626,-4.93893914224454,0.479677850220928));
#72956=CARTESIAN_POINT('Ctrl Pts',(21.5704765926236,-4.78017651587008,2.11435610222958));
#72957=CARTESIAN_POINT('Ctrl Pts',(21.5307212684845,-3.72927606286137,3.6623884688657));
#72958=CARTESIAN_POINT('Ctrl Pts',(21.4909659443455,-2.26859192696917,4.41324159316915));
#72959=CARTESIAN_POINT('Ctrl Pts',(21.4512106202064,-0.807907791077042,
5.16409471747255));
#72960=CARTESIAN_POINT('Ctrl Pts',(21.4114552960674,1.06256002769845,5.11776859944335));
#72961=CARTESIAN_POINT('Ctrl Pts',(21.3716999719283,2.48428311160319,4.29552652327873));
#72962=CARTESIAN_POINT('Ctrl Pts',(21.3319446477892,3.90600619550817,3.47328444711397));
#72963=CARTESIAN_POINT('Ctrl Pts',(21.2921893236502,4.87898454454212,1.87512641281354));
#72964=CARTESIAN_POINT('Ctrl Pts',(21.2524339995111,4.95662958117358,0.234593021684137));
#72965=CARTESIAN_POINT('Ctrl Pts',(21.2126786753721,5.03427461780502,-1.40594036944508));
#72966=CARTESIAN_POINT('Ctrl Pts',(21.172923351233,4.21658634203401,-3.08884911740338));
#72967=CARTESIAN_POINT('Ctrl Pts',(21.133168027094,2.87887654194239,-4.04169278236751));
#72968=CARTESIAN_POINT('Ctrl Pts',(21.0934127029549,1.54116674185078,-4.99453644733165));
#72969=CARTESIAN_POINT('Ctrl Pts',(21.0536573788158,-0.316564582561406,
-5.21731502930186));
#72970=CARTESIAN_POINT('Ctrl Pts',(21.0139020546768,-1.8416349533865,-4.60777510185263));
#72971=CARTESIAN_POINT('Ctrl Pts',(20.9741467305377,-3.36670532421159,-3.99823517440339));
#72972=CARTESIAN_POINT('Ctrl Pts',(20.9343914063987,-4.55911474144951,-2.55637673753478));
#72973=CARTESIAN_POINT('Ctrl Pts',(20.8946360822596,-4.8715576807707,-0.944000240313443));
#72974=CARTESIAN_POINT('Ctrl Pts',(20.8870202922212,-4.931411294756,-0.635122847617899));
#72975=CARTESIAN_POINT('Ctrl Pts',(20.8794045021827,-4.95897212714491,-0.319987827365635));
#72976=CARTESIAN_POINT('Ctrl Pts',(20.8717887121442,-4.95607142653195,-0.00434810948939879));
#72977=CARTESIAN_POINT('Ctrl Pts',(20.7664112878559,-4.95770599871256,-0.00394983957152954));
#72978=CARTESIAN_POINT('Ctrl Pts',(20.7726885646796,-4.9599688663304,-0.263892563491772));
#72979=CARTESIAN_POINT('Ctrl Pts',(20.7789658415033,-4.94129531995109,-0.52350947525168));
#72980=CARTESIAN_POINT('Ctrl Pts',(20.785243118327,-4.90055213313902,-0.779615388488902));
#72981=CARTESIAN_POINT('Ctrl Pts',(20.824998442466,-4.64251689848844,-2.40158840013364));
#72982=CARTESIAN_POINT('Ctrl Pts',(20.8647537666051,-3.49927781672605,-3.88273676132907));
#72983=CARTESIAN_POINT('Ctrl Pts',(20.9045090907441,-1.99557165697884,-4.54322629036293));
#72984=CARTESIAN_POINT('Ctrl Pts',(20.9442644148832,-0.49186549723137,-5.2037158193969));
#72985=CARTESIAN_POINT('Ctrl Pts',(20.9840197390222,1.37230774050106,-5.04354651626898));
#72986=CARTESIAN_POINT('Ctrl Pts',(21.0237750631613,2.74130879627203,-4.13623469438857));
#72987=CARTESIAN_POINT('Ctrl Pts',(21.0635303873004,4.11030985204285,-3.22892287250826));
#72988=CARTESIAN_POINT('Ctrl Pts',(21.1032857114394,4.98413872585233,-1.57446853187563));
#72989=CARTESIAN_POINT('Ctrl Pts',(21.1430410355785,4.96171558468266,0.0677482125175924));
#72990=CARTESIAN_POINT('Ctrl Pts',(21.1827963597175,4.93929244351299,1.70996495691082));
#72991=CARTESIAN_POINT('Ctrl Pts',(21.2225516838566,4.02061728736416,3.33994410506463));
#72992=CARTESIAN_POINT('Ctrl Pts',(21.2623070079956,2.62735400177417,4.20953944190376));
#72993=CARTESIAN_POINT('Ctrl Pts',(21.3020623321347,1.23409071618409,5.07913477874293));
#72994=CARTESIAN_POINT('Ctrl Pts',(21.3418176562737,-0.633760698847205,
5.18834630426734));
#72995=CARTESIAN_POINT('Ctrl Pts',(21.3815729804128,-2.11887273206807,4.48704688061987));
#72996=CARTESIAN_POINT('Ctrl Pts',(21.4213283045518,-3.60398476528886,3.78574745697245));
#72997=CARTESIAN_POINT('Ctrl Pts',(21.4610836286909,-4.70635741669926,2.27393708415325));
#72998=CARTESIAN_POINT('Ctrl Pts',(21.50083895283,-4.92001125233576,0.645523539827611));
#72999=CARTESIAN_POINT('Ctrl Pts',(21.5060297311719,-4.94790763418439,0.432904628003932));
#73000=CARTESIAN_POINT('Ctrl Pts',(21.5112205095139,-4.96065310509214,0.218297861039164));
#73001=CARTESIAN_POINT('Ctrl Pts',(21.5164112878558,-4.95893736719177,0.00348609211932242));
#73002=CARTESIAN_POINT('Origin',(10.45,0.,0.));
#73003=CARTESIAN_POINT('',(22.3717887121441,-4.9475429831306,0.00290303294213062));
#73004=CARTESIAN_POINT('',(22.2664112878559,-4.94668796515972,0.00213281205902905));
#73005=CARTESIAN_POINT('',(10.45,-4.954,-6.06690024297599E-16));
#73006=CARTESIAN_POINT('Ctrl Pts',(22.3717887121441,-4.9475429831306,0.00290303294213062));
#73007=CARTESIAN_POINT('Ctrl Pts',(22.3564683918513,-4.95093651841198,0.640642072587425));
#73008=CARTESIAN_POINT('Ctrl Pts',(22.3411480715585,-4.83658160029764,1.27721064111222));
#73009=CARTESIAN_POINT('Ctrl Pts',(22.3258277512656,-4.59886119640998,1.8637828164629));
#73010=CARTESIAN_POINT('Ctrl Pts',(22.2860724271265,-3.98199082226831,3.38590288420711));
#73011=CARTESIAN_POINT('Ctrl Pts',(22.2463171029875,-2.53441208857938,4.57136135250474));
#73012=CARTESIAN_POINT('Ctrl Pts',(22.2065617788484,-0.920551010767648,
4.87604312197529));
#73013=CARTESIAN_POINT('Ctrl Pts',(22.1668064547094,0.693310067043993,5.18072489144581));
#73014=CARTESIAN_POINT('Ctrl Pts',(22.1270511305703,2.47345348897841,4.6046299620894));
#73015=CARTESIAN_POINT('Ctrl Pts',(22.0872958064313,3.60280894777447,3.41218088275286));
#73016=CARTESIAN_POINT('Ctrl Pts',(22.0475404822922,4.73216440657066,2.21973180341618));
#73017=CARTESIAN_POINT('Ctrl Pts',(22.0077851581532,5.21073190222835,0.410928574099224));
#73018=CARTESIAN_POINT('Ctrl Pts',(21.9680298340141,4.81885312749869,-1.18400389627061));
#73019=CARTESIAN_POINT('Ctrl Pts',(21.9282745098751,4.42697435276905,-2.77893636664036));
#73020=CARTESIAN_POINT('Ctrl Pts',(21.888519185736,3.16464930765215,-4.15999807806301));
#73021=CARTESIAN_POINT('Ctrl Pts',(21.848763861597,1.61127417998797,-4.69329374828509));
#73022=CARTESIAN_POINT('Ctrl Pts',(21.8090085374579,0.057899052323781,-5.22658941850718));
#73023=CARTESIAN_POINT('Ctrl Pts',(21.7692532133189,-1.7865261578877,-4.91211904752869));
#73024=CARTESIAN_POINT('Ctrl Pts',(21.7294978891798,-3.07542636312338,-3.8942217933489));
#73025=CARTESIAN_POINT('Ctrl Pts',(21.6935948301679,-4.23943297434202,-2.97495812297814));
#73026=CARTESIAN_POINT('Ctrl Pts',(21.657691771156,-4.95035851269461,-1.48198597131669));
#73027=CARTESIAN_POINT('Ctrl Pts',(21.6217887121442,-4.96026724855995,0.00275821796382324));
#73028=CARTESIAN_POINT('Ctrl Pts',(21.5164112878558,-4.95893736719177,0.00348609211932242));
#73029=CARTESIAN_POINT('Ctrl Pts',(21.5509758336529,-4.94751254853715,-1.42691041789185));
#73030=CARTESIAN_POINT('Ctrl Pts',(21.58554037945,-4.29487617807464,-2.86639673660996));
#73031=CARTESIAN_POINT('Ctrl Pts',(21.6201049252471,-3.20466525102918,-3.78857915219258));
#73032=CARTESIAN_POINT('Ctrl Pts',(21.6598602493862,-1.95073039422339,-4.84925158405509));
#73033=CARTESIAN_POINT('Ctrl Pts',(21.6996155735252,-0.117925660749211,
-5.2255797319479));
#73034=CARTESIAN_POINT('Ctrl Pts',(21.7393708976643,1.45250755935842,-4.74483225768718));
#73035=CARTESIAN_POINT('Ctrl Pts',(21.7791262218033,3.02294077946596,-4.26408478342648));
#73036=CARTESIAN_POINT('Ctrl Pts',(21.8188815459424,4.33100248620699,-2.92626168701236));
#73037=CARTESIAN_POINT('Ctrl Pts',(21.8586368700815,4.77630376289404,-1.3454121034636));
#73038=CARTESIAN_POINT('Ctrl Pts',(21.8983921942205,5.22160503958109,0.235437480085154));
#73039=CARTESIAN_POINT('Ctrl Pts',(21.9381475183596,4.80414588621417,2.05931355076854));
#73040=CARTESIAN_POINT('Ctrl Pts',(21.9779028424986,3.71553641381448,3.28907289691194));
#73041=CARTESIAN_POINT('Ctrl Pts',(22.0176581666377,2.62692694141473,4.51883224305541));
#73042=CARTESIAN_POINT('Ctrl Pts',(22.0574134907767,0.867167149982128,5.15447486465883));
#73043=CARTESIAN_POINT('Ctrl Pts',(22.0971688149158,-0.756028561870759,
4.90424634140841));
#73044=CARTESIAN_POINT('Ctrl Pts',(22.1369241390548,-2.37922427372355,4.654017818158));
#73045=CARTESIAN_POINT('Ctrl Pts',(22.1766794631939,-3.86585590599665,3.51791815005386));
#73046=CARTESIAN_POINT('Ctrl Pts',(22.216434787333,-4.5335725033689,2.0174071776118));
#73047=CARTESIAN_POINT('Ctrl Pts',(22.2330936208406,-4.81336847703526,1.38864202457572));
#73048=CARTESIAN_POINT('Ctrl Pts',(22.2497524543482,-4.94937155730909,0.695890067533741));
#73049=CARTESIAN_POINT('Ctrl Pts',(22.2664112878559,-4.94668796515972,0.00213281205902905));
#73050=CARTESIAN_POINT('Origin',(10.45,0.,0.));
#73051=CARTESIAN_POINT('',(23.1217887121442,-4.9496403119333,-0.00395742179621961));
#73052=CARTESIAN_POINT('',(23.0164112878558,-4.95110446228237,-0.0043407105877043));
#73053=CARTESIAN_POINT('',(10.45,-4.954,-6.06690024297599E-16));
#73054=CARTESIAN_POINT('Ctrl Pts',(23.1217887121442,-4.9496403119333,-0.00395742179621961));
#73055=CARTESIAN_POINT('Ctrl Pts',(23.0950003366856,-4.94133049104857,1.1099757704877));
#73056=CARTESIAN_POINT('Ctrl Pts',(23.0682119612271,-4.56944157248637,2.22893581023816));
#73057=CARTESIAN_POINT('Ctrl Pts',(23.0414235857686,-3.87938006227662,3.09412685958389));
#73058=CARTESIAN_POINT('Ctrl Pts',(23.0016682616295,-2.8552933625529,4.37811478420478));
#73059=CARTESIAN_POINT('Ctrl Pts',(22.9619129374905,-1.13046069334654,5.10319976786228));
#73060=CARTESIAN_POINT('Ctrl Pts',(22.9221576133514,0.503434791256329,4.93657412602511));
#73061=CARTESIAN_POINT('Ctrl Pts',(22.8824022892124,2.1373302758592,4.76994848418793));
#73062=CARTESIAN_POINT('Ctrl Pts',(22.8426469650733,3.68028857585867,3.71161221685608));
#73063=CARTESIAN_POINT('Ctrl Pts',(22.8028916409343,4.42410528663325,2.24733244171209));
#73064=CARTESIAN_POINT('Ctrl Pts',(22.7631363167952,5.16792199740791,0.783052666567929));
#73065=CARTESIAN_POINT('Ctrl Pts',(22.7233809926562,5.11259711895761,-1.08717061638829));
#73066=CARTESIAN_POINT('Ctrl Pts',(22.6836256685171,4.2835242880408,-2.5049212292111));
#73067=CARTESIAN_POINT('Ctrl Pts',(22.643870344378,3.45445145712413,-3.92267184203367));
#73068=CARTESIAN_POINT('Ctrl Pts',(22.604115020239,1.85163067374112,-4.8879497847228));
#73069=CARTESIAN_POINT('Ctrl Pts',(22.5643596960999,0.210742700366703,-4.95770089910938));
#73070=CARTESIAN_POINT('Ctrl Pts',(22.5246043719609,-1.4301452730079,-5.02745201349597));
#73071=CARTESIAN_POINT('Ctrl Pts',(22.4848490478218,-3.10910043637404,-4.20167629957976));
#73072=CARTESIAN_POINT('Ctrl Pts',(22.4450937236828,-4.05549701075997,-2.8593976090262));
#73073=CARTESIAN_POINT('Ctrl Pts',(22.4206587198366,-4.63718523582063,-2.03438647714267));
#73074=CARTESIAN_POINT('Ctrl Pts',(22.3962237159904,-4.94213049526692,-1.01425297872966));
#73075=CARTESIAN_POINT('Ctrl Pts',(22.3717887121441,-4.9475429831306,0.00290303294213062));
#73076=CARTESIAN_POINT('Ctrl Pts',(22.2664112878559,-4.94668796515972,0.00213281205902905));
#73077=CARTESIAN_POINT('Ctrl Pts',(22.2895077784873,-4.94296732284056,-0.959720726137945));
#73078=CARTESIAN_POINT('Ctrl Pts',(22.3126042691187,-4.67266055328166,-1.92350666786889));
#73079=CARTESIAN_POINT('Ctrl Pts',(22.3357007597501,-4.14937595511098,-2.72137659039115));
#73080=CARTESIAN_POINT('Ctrl Pts',(22.3754560838892,-3.24866124700948,-4.09472710917176));
#73081=CARTESIAN_POINT('Ctrl Pts',(22.4152114080282,-1.59843026833517,-4.97650586995307));
#73082=CARTESIAN_POINT('Ctrl Pts',(22.4549667321673,0.043875352230013,-4.96198411092265));
#73083=CARTESIAN_POINT('Ctrl Pts',(22.4947220563063,1.68618097279528,-4.94746235189222));
#73084=CARTESIAN_POINT('Ctrl Pts',(22.5344773804454,3.32056123525127,-4.03664007305015));
#73085=CARTESIAN_POINT('Ctrl Pts',(22.5742327045844,4.1968498514374,-2.64757675772997));
#73086=CARTESIAN_POINT('Ctrl Pts',(22.6139880287235,5.07313846762344,-1.25851344240995));
#73087=CARTESIAN_POINT('Ctrl Pts',(22.6537433528625,5.19133543753951,0.608790909388));
#73088=CARTESIAN_POINT('Ctrl Pts',(22.6934986770016,4.49718938270871,2.09725988366587));
#73089=CARTESIAN_POINT('Ctrl Pts',(22.7332540011406,3.80304332787779,3.585728857944));
#73090=CARTESIAN_POINT('Ctrl Pts',(22.7730093252797,2.2965542482996,4.69536245470199));
#73091=CARTESIAN_POINT('Ctrl Pts',(22.8127646494188,0.669187494445402,4.91684852937937));
#73092=CARTESIAN_POINT('Ctrl Pts',(22.8525199735578,-0.958179259408607,
5.13833460405671));
#73093=CARTESIAN_POINT('Ctrl Pts',(22.8922752976969,-2.7064236875387,4.47167315665366));
#73094=CARTESIAN_POINT('Ctrl Pts',(22.9320306218359,-3.77311684267058,3.22285597803218));
#73095=CARTESIAN_POINT('Ctrl Pts',(22.9601575105092,-4.52780216527098,2.33931792326669));
#73096=CARTESIAN_POINT('Ctrl Pts',(22.9882843991825,-4.94133281501348,1.16437824414132));
#73097=CARTESIAN_POINT('Ctrl Pts',(23.0164112878558,-4.95110446228237,-0.0043407105877043));
#73098=CARTESIAN_POINT('Origin',(10.45,0.,0.));
#73099=CARTESIAN_POINT('',(23.8717887121442,-4.96185463563362,-0.00114991572043255));
#73100=CARTESIAN_POINT('',(23.7664112878558,-4.96217415958626,-0.000124643869615789));
#73101=CARTESIAN_POINT('',(10.45,-4.954,-6.06690024297599E-16));
#73102=CARTESIAN_POINT('Ctrl Pts',(23.8717887121442,-4.96185463563362,-0.00114991572043255));
#73103=CARTESIAN_POINT('Ctrl Pts',(23.83353228152,-4.95690705322659,1.57957432325722));
#73104=CARTESIAN_POINT('Ctrl Pts',(23.7952758508957,-4.13589002242756,3.16471783957375));
#73105=CARTESIAN_POINT('Ctrl Pts',(23.7570194202716,-2.83985248590647,4.06920736127795));
#73106=CARTESIAN_POINT('Ctrl Pts',(23.7172640961325,-1.49303597636527,5.00913493761048));
#73107=CARTESIAN_POINT('Ctrl Pts',(23.6775087719935,0.366753005962177,5.2140273764652));
#73108=CARTESIAN_POINT('Ctrl Pts',(23.6377534478545,1.88588753612861,4.58984083513389));
#73109=CARTESIAN_POINT('Ctrl Pts',(23.5979981237154,3.40502206629521,3.96565429380252));
#73110=CARTESIAN_POINT('Ctrl Pts',(23.5582427995763,4.5835021443006,2.51238877228494));
#73111=CARTESIAN_POINT('Ctrl Pts',(23.5184874754372,4.88041569105472,0.897080472028412));
#73112=CARTESIAN_POINT('Ctrl Pts',(23.4787321512982,5.17732923780883,-0.718227828228022));
#73113=CARTESIAN_POINT('Ctrl Pts',(23.4389768271592,4.59267625331161,-2.49557890722352));
#73114=CARTESIAN_POINT('Ctrl Pts',(23.3992215030201,3.39480735909076,-3.61918411875537));
#73115=CARTESIAN_POINT('Ctrl Pts',(23.3594661788811,2.19693846486984,-4.74278933028729));
#73116=CARTESIAN_POINT('Ctrl Pts',(23.319710854742,0.385853660925542,-5.21264867435566));
#73117=CARTESIAN_POINT('Ctrl Pts',(23.2799555306029,-1.20717492095737,-4.81310080935351));
#73118=CARTESIAN_POINT('Ctrl Pts',(23.2402002064639,-2.8002035028401,-4.4135529443514));
#73119=CARTESIAN_POINT('Ctrl Pts',(23.2004448823248,-4.17517586266139,-3.14459787027861));
#73120=CARTESIAN_POINT('Ctrl Pts',(23.1606895581858,-4.70099167745142,-1.58867490045016));
#73121=CARTESIAN_POINT('Ctrl Pts',(23.1477226095052,-4.87249642136824,-1.08118128198365));
#73122=CARTESIAN_POINT('Ctrl Pts',(23.1347556608247,-4.9536626917571,-0.54315826136416));
#73123=CARTESIAN_POINT('Ctrl Pts',(23.1217887121442,-4.9496403119333,-0.00395742179621961));
#73124=CARTESIAN_POINT('Ctrl Pts',(23.0164112878558,-4.95110446228237,-0.0043407105877043));
#73125=CARTESIAN_POINT('Ctrl Pts',(23.0280397233216,-4.95514433213716,-0.487521523813275));
#73126=CARTESIAN_POINT('Ctrl Pts',(23.0396681587874,-4.89017271197347,-0.969639075397733));
#73127=CARTESIAN_POINT('Ctrl Pts',(23.0512965942531,-4.75176572372991,-1.42966215252686));
#73128=CARTESIAN_POINT('Ctrl Pts',(23.0910519183922,-4.27857956752358,-3.00239019462453));
#73129=CARTESIAN_POINT('Ctrl Pts',(23.1308072425312,-2.94706537297713,-4.3168733689798));
#73130=CARTESIAN_POINT('Ctrl Pts',(23.1705625666703,-1.36837654416773,-4.76977536126742));
#73131=CARTESIAN_POINT('Ctrl Pts',(23.2103178908093,0.210312284641578,-5.22267735355501));
#73132=CARTESIAN_POINT('Ctrl Pts',(23.2500732149484,2.03617574771381,-4.81399816377506));
#73133=CARTESIAN_POINT('Ctrl Pts',(23.2898285390874,3.27115843759854,-3.73131797622636));
#73134=CARTESIAN_POINT('Ctrl Pts',(23.3295838632265,4.50614112748327,-2.64863778867767));
#73135=CARTESIAN_POINT('Ctrl Pts',(23.3693391873655,5.1502430441805,-0.89195660336024));
#73136=CARTESIAN_POINT('Ctrl Pts',(23.4090945115046,4.90782702469611,0.732424234473895));
#73137=CARTESIAN_POINT('Ctrl Pts',(23.4488498356436,4.66541100521171,2.35680507230812));
#73138=CARTESIAN_POINT('Ctrl Pts',(23.4886051597827,3.53647704954558,3.84888556265903));
#73139=CARTESIAN_POINT('Ctrl Pts',(23.5283604839218,2.0391959986918,4.52381377186346));
#73140=CARTESIAN_POINT('Ctrl Pts',(23.5681158080608,0.541914947838193,5.1987419810678));
#73141=CARTESIAN_POINT('Ctrl Pts',(23.6078711321999,-1.32371319820299,5.05651790912584));
#73142=CARTESIAN_POINT('Ctrl Pts',(23.6476264563389,-2.70138138925913,4.16242116482061));
#73143=CARTESIAN_POINT('Ctrl Pts',(23.6872214001779,-4.07349181308097,3.27193137146485));
#73144=CARTESIAN_POINT('Ctrl Pts',(23.7268163440169,-4.96157138121483,1.6356230549814));
#73145=CARTESIAN_POINT('Ctrl Pts',(23.7664112878558,-4.96217415958626,-0.000124643869615789));
#73146=CARTESIAN_POINT('Origin',(10.45,0.,0.));
#73147=CARTESIAN_POINT('',(24.6217887121442,-4.95310191319871,0.00456049067516617));
#73148=CARTESIAN_POINT('',(24.5164112878558,-4.95147756391153,0.00440602753503367));
#73149=CARTESIAN_POINT('',(10.45,-4.954,-6.06690024297599E-16));
#73150=CARTESIAN_POINT('Ctrl Pts',(24.6217887121442,-4.95310191319871,0.00456049067516617));
#73151=CARTESIAN_POINT('Ctrl Pts',(24.6118195504934,-4.95685877086284,0.418371613716965));
#73152=CARTESIAN_POINT('Ctrl Pts',(24.6018503888425,-4.90934967455833,0.831332155126853));
#73153=CARTESIAN_POINT('Ctrl Pts',(24.5918812271917,-4.80723707609103,1.23031800159294));
#73154=CARTESIAN_POINT('Ctrl Pts',(24.5521259030527,-4.40002936967154,2.82140581908015));
#73155=CARTESIAN_POINT('Ctrl Pts',(24.5123705789136,-3.12447364079982,4.19025699902268));
#73156=CARTESIAN_POINT('Ctrl Pts',(24.4726152547746,-1.56603884578366,4.70858078663671));
#73157=CARTESIAN_POINT('Ctrl Pts',(24.4328599306355,-0.00760405076757592,
5.22690457425072));
#73158=CARTESIAN_POINT('Ctrl Pts',(24.3931046064965,1.83370981039292,4.89470096953634));
#73159=CARTESIAN_POINT('Ctrl Pts',(24.3533492823574,3.11275573225721,3.86444853013826));
#73160=CARTESIAN_POINT('Ctrl Pts',(24.3135939582184,4.39180165412149,2.83419609074018));
#73161=CARTESIAN_POINT('Ctrl Pts',(24.2738386340793,5.10857963668957,1.1058948166584));
#73162=CARTESIAN_POINT('Ctrl Pts',(24.2340833099402,4.93409483649058,-0.527180078630499));
#73163=CARTESIAN_POINT('Ctrl Pts',(24.1943279858012,4.75961003629158,-2.16025497391949));
#73164=CARTESIAN_POINT('Ctrl Pts',(24.1545726616621,3.69386245332543,-3.69810349041561));
#73165=CARTESIAN_POINT('Ctrl Pts',(24.1148173375231,2.2260209345218,-4.4348665695665));
#73166=CARTESIAN_POINT('Ctrl Pts',(24.075062013384,0.758179415718254,-5.17162964871735));
#73167=CARTESIAN_POINT('Ctrl Pts',(24.035306689245,-1.11175603892272,-5.10730729052307));
#73168=CARTESIAN_POINT('Ctrl Pts',(23.9955513651059,-2.52550136214219,-4.27142289648377));
#73169=CARTESIAN_POINT('Ctrl Pts',(23.9557960409669,-3.93924668536173,-3.43553850244443));
#73170=CARTESIAN_POINT('Ctrl Pts',(23.9160407168278,-4.89680187715972,-1.82809207255998));
#73171=CARTESIAN_POINT('Ctrl Pts',(23.8762853926888,-4.95865745468119,-0.186887500712485));
#73172=CARTESIAN_POINT('Ctrl Pts',(23.8747864991739,-4.96098959323151,-0.125009225473019));
#73173=CARTESIAN_POINT('Ctrl Pts',(23.873287605659,-4.9620484827611,-0.0630829625817651));
#73174=CARTESIAN_POINT('Ctrl Pts',(23.8717887121442,-4.96185463563362,-0.00114991572043255));
#73175=CARTESIAN_POINT('Ctrl Pts',(23.7664112878558,-4.96217415958626,-0.000124643869615789));
#73176=CARTESIAN_POINT('Ctrl Pts',(23.7665716681559,-4.96217660115497,-0.0067502804120735));
#73177=CARTESIAN_POINT('Ctrl Pts',(23.766732048456,-4.96216448211318,-0.0133759077566162));
#73178=CARTESIAN_POINT('Ctrl Pts',(23.7668924287561,-4.96213777564951,-0.0200014763019115));
#73179=CARTESIAN_POINT('Ctrl Pts',(23.8066477528951,-4.9555177349126,-1.66235795645061));
#73180=CARTESIAN_POINT('Ctrl Pts',(23.8464030770342,-4.05256941736739,-3.30110150007939));
#73181=CARTESIAN_POINT('Ctrl Pts',(23.8861584011732,-2.66773822677601,-4.18406311101782));
#73182=CARTESIAN_POINT('Ctrl Pts',(23.9259137253123,-1.2829070361847,-5.06702472195621));
#73183=CARTESIAN_POINT('Ctrl Pts',(23.9656690494514,0.583807027452744,-5.19420440020456));
#73184=CARTESIAN_POINT('Ctrl Pts',(24.0054243735904,2.07559848725656,-4.5072277824934));
#73185=CARTESIAN_POINT('Ctrl Pts',(24.0451796977295,3.56738994706038,-3.82025116478225));
#73186=CARTESIAN_POINT('Ctrl Pts',(24.0849350218685,4.68425880303048,-2.31911825111164));
#73187=CARTESIAN_POINT('Ctrl Pts',(24.1246903460076,4.91357198972193,-0.692835958508393));
#73188=CARTESIAN_POINT('Ctrl Pts',(24.1644456701466,5.14288517641339,0.933446334094952));
#73189=CARTESIAN_POINT('Ctrl Pts',(24.2042009942857,4.48464269382609,2.68487800563082));
#73190=CARTESIAN_POINT('Ctrl Pts',(24.2439563184248,3.24097210138753,3.75756719189555));
#73191=CARTESIAN_POINT('Ctrl Pts',(24.2837116425638,1.99730150894912,4.83025637816016));
#73192=CARTESIAN_POINT('Ctrl Pts',(24.3234669667029,0.168202806659376,5.22420307915372));
#73193=CARTESIAN_POINT('Ctrl Pts',(24.3632222908419,-1.40678365144245,4.75858919445841));
#73194=CARTESIAN_POINT('Ctrl Pts',(24.402977614981,-2.98177010954438,4.29297530976307));
#73195=CARTESIAN_POINT('Ctrl Pts',(24.44273293912,-4.30264432345847,2.96780083937893));
#73196=CARTESIAN_POINT('Ctrl Pts',(24.4824882632591,-4.76313654743402,1.39130930927687));
#73197=CARTESIAN_POINT('Ctrl Pts',(24.4937959381246,-4.89411513859417,0.942905126018314));
#73198=CARTESIAN_POINT('Ctrl Pts',(24.5051036129902,-4.95548762377079,0.474169041233779));
#73199=CARTESIAN_POINT('Ctrl Pts',(24.5164112878558,-4.95147756391153,0.00440602753503367));
#73200=CARTESIAN_POINT('Origin',(10.45,0.,0.));
#73201=CARTESIAN_POINT('',(25.3717887121441,-4.94601914232448,-0.00106424482321954));
#73202=CARTESIAN_POINT('',(25.2664112878558,-4.94652387558086,-0.00193440418662929));
#73203=CARTESIAN_POINT('',(10.45,-4.954,-6.06690024297599E-16));
#73204=CARTESIAN_POINT('Ctrl Pts',(25.3717887121441,-4.94601914232448,-0.00106424482321954));
#73205=CARTESIAN_POINT('Ctrl Pts',(25.3503514953277,-4.94430911377561,0.891990181583246));
#73206=CARTESIAN_POINT('Ctrl Pts',(25.3289142785112,-4.71361814782464,1.78586821550294));
#73207=CARTESIAN_POINT('Ctrl Pts',(25.3074770616947,-4.25922262873376,2.54602303400226));
#73208=CARTESIAN_POINT('Ctrl Pts',(25.2677217375557,-3.41654602087722,3.95573034181289));
#73209=CARTESIAN_POINT('Ctrl Pts',(25.2279664134166,-1.80451115414936,4.90554061694139));
#73210=CARTESIAN_POINT('Ctrl Pts',(25.1882110892775,-0.163027974930276,
4.95949922574628));
#73211=CARTESIAN_POINT('Ctrl Pts',(25.1484557651385,1.47845520428881,5.01345783455117));
#73212=CARTESIAN_POINT('Ctrl Pts',(25.1087004409995,3.14938669599915,4.17156477703208));
#73213=CARTESIAN_POINT('Ctrl Pts',(25.0689451168604,4.08282351654977,2.82024162502009));
#73214=CARTESIAN_POINT('Ctrl Pts',(25.0291897927214,5.01626033710039,1.46891847300811));
#73215=CARTESIAN_POINT('Ctrl Pts',(24.9894344685823,5.21220248649166,-0.391834773496653));
#73216=CARTESIAN_POINT('Ctrl Pts',(24.9496791444432,4.58071422682977,-1.90794860069844));
#73217=CARTESIAN_POINT('Ctrl Pts',(24.9099238203042,3.94922596716785,-3.42406242790032));
#73218=CARTESIAN_POINT('Ctrl Pts',(24.8701684961651,2.49030729845252,-4.595536835799));
#73219=CARTESIAN_POINT('Ctrl Pts',(24.8304131720261,0.873589167397777,-4.88467528679165));
#73220=CARTESIAN_POINT('Ctrl Pts',(24.790657847887,-0.743128963656787,-5.17381373778427));
#73221=CARTESIAN_POINT('Ctrl Pts',(24.750902523748,-2.51764655705084,-4.58061623187108));
#73222=CARTESIAN_POINT('Ctrl Pts',(24.7111471996089,-3.63547551176423,-3.3773552513987));
#73223=CARTESIAN_POINT('Ctrl Pts',(24.6813610371207,-4.47299440012012,-2.47582752256508));
#73224=CARTESIAN_POINT('Ctrl Pts',(24.6515748746324,-4.94187706032252,-1.23183688977808));
#73225=CARTESIAN_POINT('Ctrl Pts',(24.6217887121442,-4.95310191319871,0.00456049067516617));
#73226=CARTESIAN_POINT('Ctrl Pts',(24.5164112878558,-4.95147756391153,0.00440602753503367));
#73227=CARTESIAN_POINT('Ctrl Pts',(24.5448589371293,-4.94138912594368,-1.1774154887533));
#73228=CARTESIAN_POINT('Ctrl Pts',(24.5733065864028,-4.51748403237577,-2.36573660349833));
#73229=CARTESIAN_POINT('Ctrl Pts',(24.6017542356762,-3.74701316495806,-3.2531682565175));
#73230=CARTESIAN_POINT('Ctrl Pts',(24.6415095598153,-2.67028732446968,-4.49334570238973));
#73231=CARTESIAN_POINT('Ctrl Pts',(24.6812648839543,-0.916725409456256,
-5.14589200431422));
#73232=CARTESIAN_POINT('Ctrl Pts',(24.7210202080934,0.708802952698988,-4.9112941001153));
#73233=CARTESIAN_POINT('Ctrl Pts',(24.7607755322324,2.33433131485405,-4.6766961959164));
#73234=CARTESIAN_POINT('Ctrl Pts',(24.8005308563715,3.83182612415081,-3.55495408559414));
#73235=CARTESIAN_POINT('Ctrl Pts',(24.8402861805106,4.51395032174456,-2.06093761584487));
#73236=CARTESIAN_POINT('Ctrl Pts',(24.8800415046496,5.19607451933846,-0.566921146095265));
#73237=CARTESIAN_POINT('Ctrl Pts',(24.9197968287887,5.062828105229,1.29936968308167));
#73238=CARTESIAN_POINT('Ctrl Pts',(24.9595521529278,4.17537002154208,2.68132365573233));
#73239=CARTESIAN_POINT('Ctrl Pts',(24.9993074770668,3.28791193785532,4.06327762838277));
#73240=CARTESIAN_POINT('Ctrl Pts',(25.0390628012058,1.64624218459133,4.96089474450724));
#73241=CARTESIAN_POINT('Ctrl Pts',(25.0788181253449,0.0038728626253081,
4.96217657530616));
#73242=CARTESIAN_POINT('Ctrl Pts',(25.1185734494839,-1.63849645934071,4.96345840610509));
#73243=CARTESIAN_POINT('Ctrl Pts',(25.158328773623,-3.28156535000864,4.0684049515787));
#73244=CARTESIAN_POINT('Ctrl Pts',(25.1980840977621,-4.1711795166362,2.6878379422087));
#73245=CARTESIAN_POINT('Ctrl Pts',(25.2208598277933,-4.68083734310046,1.89691440740134));
#73246=CARTESIAN_POINT('Ctrl Pts',(25.2436355578246,-4.94320253847257,0.946639659339477));
#73247=CARTESIAN_POINT('Ctrl Pts',(25.2664112878558,-4.94652387558086,-0.00193440418662929));
#73248=CARTESIAN_POINT('Origin',(10.45,0.,0.));
#73249=CARTESIAN_POINT('',(26.1217887121441,-4.95701837283973,-0.00414435129742319));
#73250=CARTESIAN_POINT('',(26.0164112878558,-4.95858561828336,-0.00363551008735497));
#73251=CARTESIAN_POINT('',(10.45,-4.954,-6.06690024297599E-16));
#73252=CARTESIAN_POINT('Ctrl Pts',(26.1217887121441,-4.95701837283973,-0.00414435129742319));
#73253=CARTESIAN_POINT('Ctrl Pts',(26.088883440162,-4.94479832228077,1.35895636761934));
#73254=CARTESIAN_POINT('Ctrl Pts',(26.0559781681799,-4.36019767419945,2.73126401776642));
#73255=CARTESIAN_POINT('Ctrl Pts',(26.0230728961977,-3.35982496366235,3.65168274968392));
#73256=CARTESIAN_POINT('Ctrl Pts',(25.9833175720587,-2.15119975038825,4.76370957173509));
#73257=CARTESIAN_POINT('Ctrl Pts',(25.9435622479196,-0.33567761965343,5.21612018511601));
#73258=CARTESIAN_POINT('Ctrl Pts',(25.9038069237805,1.25343260245453,4.80126206344664));
#73259=CARTESIAN_POINT('Ctrl Pts',(25.8640515996415,2.84254282456258,4.38640394177725));
#73260=CARTESIAN_POINT('Ctrl Pts',(25.8242962755024,4.20524113804382,3.10427708505783));
#73261=CARTESIAN_POINT('Ctrl Pts',(25.7845409513634,4.71606090016571,1.54336653997552));
#73262=CARTESIAN_POINT('Ctrl Pts',(25.7447856272243,5.22688066228767,-0.0175440051069695));
#73263=CARTESIAN_POINT('Ctrl Pts',(25.7050303030853,4.88582187304976,-1.85723823855216));
#73264=CARTESIAN_POINT('Ctrl Pts',(25.6652749789462,3.84942754257308,-3.13131254991698));
#73265=CARTESIAN_POINT('Ctrl Pts',(25.6255196548072,2.81303321209658,-4.40538686128159));
#73266=CARTESIAN_POINT('Ctrl Pts',(25.5857643306681,1.08130334038127,-5.11384125056608));
#73267=CARTESIAN_POINT('Ctrl Pts',(25.5460090065291,-0.550913162680595,
-4.93150133103228));
#73268=CARTESIAN_POINT('Ctrl Pts',(25.50625368239,-2.18312966574265,-4.74916141149845));
#73269=CARTESIAN_POINT('Ctrl Pts',(25.4664983582509,-3.71583280015141,-3.6760271831463));
#73270=CARTESIAN_POINT('Ctrl Pts',(25.4267430341119,-4.44552519286334,-2.20465789872378));
#73271=CARTESIAN_POINT('Ctrl Pts',(25.4084249267893,-4.78174641232606,-1.52669334814114));
#73272=CARTESIAN_POINT('Ctrl Pts',(25.3901068194667,-4.94748036216244,-0.764179483516399));
#73273=CARTESIAN_POINT('Ctrl Pts',(25.3717887121441,-4.94601914232448,-0.00106424482321954));
#73274=CARTESIAN_POINT('Ctrl Pts',(25.2664112878558,-4.94652387558086,-0.00193440418662929));
#73275=CARTESIAN_POINT('Ctrl Pts',(25.2833908819636,-4.94899997430159,-0.709108337042042));
#73276=CARTESIAN_POINT('Ctrl Pts',(25.3003704760714,-4.80750232985598,-1.41533704803351));
#73277=CARTESIAN_POINT('Ctrl Pts',(25.3173500701792,-4.5171618476025,-2.05388904426371));
#73278=CARTESIAN_POINT('Ctrl Pts',(25.3571053943183,-3.83737056935426,-3.5489684571522));
#73279=CARTESIAN_POINT('Ctrl Pts',(25.3968607184573,-2.34162857027089,-4.6730467187156));
#73280=CARTESIAN_POINT('Ctrl Pts',(25.4366160425964,-0.716468384594204,
-4.91018170920986));
#73281=CARTESIAN_POINT('Ctrl Pts',(25.4763713667355,0.908691801082482,-5.14731669970413));
#73282=CARTESIAN_POINT('Ctrl Pts',(25.5161266908745,2.66327017335248,-4.49750841912926));
#73283=CARTESIAN_POINT('Ctrl Pts',(25.5558820150136,3.74193055981534,-3.25901320173794));
#73284=CARTESIAN_POINT('Ctrl Pts',(25.5956373391526,4.82059094627832,-2.02051798434648));
#73285=CARTESIAN_POINT('Ctrl Pts',(25.6353926632917,5.22333334693401,-0.193335830138429));
#73286=CARTESIAN_POINT('Ctrl Pts',(25.6751479874307,4.76530251192093,1.38387258570369));
#73287=CARTESIAN_POINT('Ctrl Pts',(25.7149033115698,4.30727167690792,2.96108100154554));
#73288=CARTESIAN_POINT('Ctrl Pts',(25.7546586357088,2.98846760622648,4.28831567902156));
#73289=CARTESIAN_POINT('Ctrl Pts',(25.7944139598479,1.41420986793587,4.75638747507128));
#73290=CARTESIAN_POINT('Ctrl Pts',(25.8341692839869,-0.160047870354837,
5.22445927112102));
#73291=CARTESIAN_POINT('Ctrl Pts',(25.873924608126,-1.98975927625474,4.83336818574436));
#73292=CARTESIAN_POINT('Ctrl Pts',(25.9136799322651,-3.23510277011079,3.76262161669275));
#73293=CARTESIAN_POINT('Ctrl Pts',(25.947923717462,-4.3077962023373,2.84031960293728));
#73294=CARTESIAN_POINT('Ctrl Pts',(25.9821675026589,-4.94691956774523,1.4137491866956));
#73295=CARTESIAN_POINT('Ctrl Pts',(26.0164112878558,-4.95858561828336,-0.00363551008735497));
#73296=CARTESIAN_POINT('Origin',(10.45,0.,0.));
#73297=CARTESIAN_POINT('',(26.8717887121441,-4.9595359561886,0.00319450674940359));
#73298=CARTESIAN_POINT('',(26.7664112878558,-4.95808068667962,0.00382558555664219));
#73299=CARTESIAN_POINT('',(10.45,-4.954,-6.06690024297599E-16));
#73300=CARTESIAN_POINT('Ctrl Pts',(26.8717887121441,-4.9595359561886,0.00319450674940359));
#73301=CARTESIAN_POINT('Ctrl Pts',(26.8671707091353,-4.96096588983627,0.194242562984014));
#73302=CARTESIAN_POINT('Ctrl Pts',(26.8625527061266,-4.9508863525858,0.385138317086643));
#73303=CARTESIAN_POINT('Ctrl Pts',(26.8579347031178,-4.92879366968551,0.574633494025437));
#73304=CARTESIAN_POINT('Ctrl Pts',(26.8181793789788,-4.73860285167671,2.20595382181785));
#73305=CARTESIAN_POINT('Ctrl Pts',(26.7784240548398,-3.65810681917519,3.73347609466237));
#73306=CARTESIAN_POINT('Ctrl Pts',(26.7386687307007,-2.18324382883633,4.45608090979461));
#73307=CARTESIAN_POINT('Ctrl Pts',(26.6989134065617,-0.708380838497551,
5.1786857249268));
#73308=CARTESIAN_POINT('Ctrl Pts',(26.6591580824226,1.16084910967861,5.09637308234685));
#73309=CARTESIAN_POINT('Ctrl Pts',(26.6194027582835,2.56648576974824,4.24692376720699));
#73310=CARTESIAN_POINT('Ctrl Pts',(26.5796474341444,3.97212242981795,3.39747445206709));
#73311=CARTESIAN_POINT('Ctrl Pts',(26.5398921100054,4.91416580178117,1.78088846436712));
#73312=CARTESIAN_POINT('Ctrl Pts',(26.5001367858664,4.96022619281914,0.139164675326781));
#73313=CARTESIAN_POINT('Ctrl Pts',(26.4603814617273,5.0062865838571,-1.50255911371347));
#73314=CARTESIAN_POINT('Ctrl Pts',(26.4206261375882,4.15636399397013,-3.169420704094));
#73315=CARTESIAN_POINT('Ctrl Pts',(26.3808708134492,2.80056548032569,-4.09634516138423));
#73316=CARTESIAN_POINT('Ctrl Pts',(26.3411154893101,1.44476696668117,-5.02326961867452));
#73317=CARTESIAN_POINT('Ctrl Pts',(26.3013601651711,-0.416907470720896,
-5.21025694287418));
#73318=CARTESIAN_POINT('Ctrl Pts',(26.2616048410321,-1.9299654994954,-4.57148158276344));
#73319=CARTESIAN_POINT('Ctrl Pts',(26.221849516893,-3.44302352826974,-3.93270622265277));
#73320=CARTESIAN_POINT('Ctrl Pts',(26.1820941927539,-4.60746514841668,-2.46816817823187));
#73321=CARTESIAN_POINT('Ctrl Pts',(26.1423388686149,-4.88882181058346,-0.850077640660699));
#73322=CARTESIAN_POINT('Ctrl Pts',(26.135488816458,-4.93730104832772,-0.57127210160384));
#73323=CARTESIAN_POINT('Ctrl Pts',(26.128638764301,-4.95956228081091,-0.287907725894975));
#73324=CARTESIAN_POINT('Ctrl Pts',(26.1217887121441,-4.95701837283973,-0.00414435129742319));
#73325=CARTESIAN_POINT('Ctrl Pts',(26.0164112878558,-4.95858561828336,-0.00363551008735497));
#73326=CARTESIAN_POINT('Ctrl Pts',(26.021922826798,-4.96046326970163,-0.231763648006996));
#73327=CARTESIAN_POINT('Ctrl Pts',(26.0274343657401,-4.94608669044165,-0.459653830611601));
#73328=CARTESIAN_POINT('Ctrl Pts',(26.0329459046822,-4.9146474874091,-0.685165263338358));
#73329=CARTESIAN_POINT('Ctrl Pts',(26.0727012288213,-4.6878731290391,-2.31180352159104));
#73330=CARTESIAN_POINT('Ctrl Pts',(26.1124565529603,-3.57334883048701,-3.81467798536976));
#73331=CARTESIAN_POINT('Ctrl Pts',(26.1522118770994,-2.08263152578818,-4.50398238133491));
#73332=CARTESIAN_POINT('Ctrl Pts',(26.1919672012384,-0.591914221089427,
-5.19328677730003));
#73333=CARTESIAN_POINT('Ctrl Pts',(26.2317225253775,1.27499608975594,-5.06902110545165));
#73334=CARTESIAN_POINT('Ctrl Pts',(26.2714778495165,2.66120385411115,-4.1882222255327));
#73335=CARTESIAN_POINT('Ctrl Pts',(26.3112331736556,4.0474116184666,-3.3074233456136));
#73336=CARTESIAN_POINT('Ctrl Pts',(26.3509884977947,4.95291683633171,-1.67009125762339));
#73337=CARTESIAN_POINT('Ctrl Pts',(26.3907438219337,4.96210050899447,-0.0277471119028885));
#73338=CARTESIAN_POINT('Ctrl Pts',(26.4304991460728,4.97128418165723,1.61459703381733));
#73339=CARTESIAN_POINT('Ctrl Pts',(26.4702544702118,4.08414630911817,3.26195323726807));
#73340=CARTESIAN_POINT('Ctrl Pts',(26.5100097943509,2.70787543875327,4.1581993665262));
#73341=CARTESIAN_POINT('Ctrl Pts',(26.5497651184899,1.33160456838828,5.05444549578438));
#73342=CARTESIAN_POINT('Ctrl Pts',(26.589520442629,-0.53379929980252,5.19958155084983));
#73343=CARTESIAN_POINT('Ctrl Pts',(26.629275766768,-2.03213205722407,4.52699134807925));
#73344=CARTESIAN_POINT('Ctrl Pts',(26.6690310909071,-3.53046481464571,3.85440114530863));
#73345=CARTESIAN_POINT('Ctrl Pts',(26.7087864150461,-4.66172646129797,2.36408468470192));
#73346=CARTESIAN_POINT('Ctrl Pts',(26.7485417391852,-4.90667776632238,0.740084225652552));
#73347=CARTESIAN_POINT('Ctrl Pts',(26.7544982554087,-4.94337867252687,0.496761216952243));
#73348=CARTESIAN_POINT('Ctrl Pts',(26.7604547716323,-4.96018293254122,0.250437156483314));
#73349=CARTESIAN_POINT('Ctrl Pts',(26.7664112878558,-4.95808068667962,0.00382558555664219));
#73350=CARTESIAN_POINT('Origin',(10.45,0.,0.));
#73351=CARTESIAN_POINT('',(27.6217887121441,-4.94702083875962,0.0024746876873416));
#73352=CARTESIAN_POINT('',(27.5164112878558,-4.94632349813665,0.00165195671278186));
#73353=CARTESIAN_POINT('',(10.45,-4.954,-6.06690024297599E-16));
#73354=CARTESIAN_POINT('Ctrl Pts',(27.6217887121441,-4.94702083875962,0.0024746876873416));
#73355=CARTESIAN_POINT('Ctrl Pts',(27.6057026539697,-4.95003929944518,0.672266001052461));
#73356=CARTESIAN_POINT('Ctrl Pts',(27.5896165957953,-4.82355113413133,1.34096495790584));
#73357=CARTESIAN_POINT('Ctrl Pts',(27.5735305376208,-4.56214311665504,1.95193772286538));
#73358=CARTESIAN_POINT('Ctrl Pts',(27.5337752134818,-3.91609544266134,3.46190492848642));
#73359=CARTESIAN_POINT('Ctrl Pts',(27.4940198893428,-2.44597192410526,4.61928680603406));
#73360=CARTESIAN_POINT('Ctrl Pts',(27.4542645652037,-0.826546436067746,
4.89285516644541));
#73361=CARTESIAN_POINT('Ctrl Pts',(27.4145092410646,0.79287905196968,5.16642352685675));
#73362=CARTESIAN_POINT('Ctrl Pts',(27.3747539169256,2.56160650948843,4.5561783701319));
#73363=CARTESIAN_POINT('Ctrl Pts',(27.3349985927865,3.66780545734341,3.34221690167914));
#73364=CARTESIAN_POINT('Ctrl Pts',(27.2952432686474,4.77400440519833,2.12825543322646));
#73365=CARTESIAN_POINT('Ctrl Pts',(27.2554879445084,5.2176748433895,0.31057765304573));
#73366=CARTESIAN_POINT('Ctrl Pts',(27.2157326203694,4.7951759097319,-1.27651818847781));
#73367=CARTESIAN_POINT('Ctrl Pts',(27.1759772962303,4.37267697607426,-2.86361403000153));
#73368=CARTESIAN_POINT('Ctrl Pts',(27.1362219720912,3.0840086705678,-4.22012793286816));
#73369=CARTESIAN_POINT('Ctrl Pts',(27.0964666479522,1.52065850784982,-4.72343184488691));
#73370=CARTESIAN_POINT('Ctrl Pts',(27.0567113238131,-0.0426916548680703,
-5.22673575690563));
#73371=CARTESIAN_POINT('Ctrl Pts',(27.0169559996741,-1.88072367479736,-4.87682967807652));
#73372=CARTESIAN_POINT('Ctrl Pts',(26.977200675535,-3.14979688300393,-3.83431744729183));
#73373=CARTESIAN_POINT('Ctrl Pts',(26.9420633544047,-4.27145376344193,-2.91290408119225));
#73374=CARTESIAN_POINT('Ctrl Pts',(26.9069260332744,-4.94865592045064,-1.45044614495815));
#73375=CARTESIAN_POINT('Ctrl Pts',(26.8717887121441,-4.9595359561886,0.00319450674940359));
#73376=CARTESIAN_POINT('Ctrl Pts',(26.7664112878558,-4.95808068667962,0.00382558555664219));
#73377=CARTESIAN_POINT('Ctrl Pts',(26.8002100957713,-4.94615200195839,-1.3955120142548));
#73378=CARTESIAN_POINT('Ctrl Pts',(26.8340089036869,-4.32548676253793,-2.8041066458325));
#73379=CARTESIAN_POINT('Ctrl Pts',(26.8678077116024,-3.27697886146211,-3.72620730839182));
#73380=CARTESIAN_POINT('Ctrl Pts',(26.9075630357414,-2.04368768818079,-4.81081392589505));
#73381=CARTESIAN_POINT('Ctrl Pts',(26.9473183598805,-0.218464378221529,
-5.22234270340963));
#73382=CARTESIAN_POINT('Ctrl Pts',(26.9870736840195,1.36092948566179,-4.77190552071585));
#73383=CARTESIAN_POINT('Ctrl Pts',(27.0268290081586,2.9403233495451,-4.32146833802208));
#73384=CARTESIAN_POINT('Ctrl Pts',(27.0665843322976,4.27388776735247,-3.00906519511995));
#73385=CARTESIAN_POINT('Ctrl Pts',(27.1063396564367,4.74952830040862,-1.4370776900362));
#73386=CARTESIAN_POINT('Ctrl Pts',(27.1460949805758,5.22516883346478,0.134909815047647));
#73387=CARTESIAN_POINT('Ctrl Pts',(27.1858503047148,4.84288548176958,1.96648168231316));
#73388=CARTESIAN_POINT('Ctrl Pts',(27.2256056288539,3.77814297012091,3.2169623965642));
#73389=CARTESIAN_POINT('Ctrl Pts',(27.2653609529929,2.71340045847224,4.46744311081523));
#73390=CARTESIAN_POINT('Ctrl Pts',(27.305116277132,0.966198786870095,5.13683267205178));
#73391=CARTESIAN_POINT('Ctrl Pts',(27.344871601271,-0.661511713564407,4.9178871089523));
#73392=CARTESIAN_POINT('Ctrl Pts',(27.3846269254101,-2.28922221399882,4.69894154585283));
#73393=CARTESIAN_POINT('Ctrl Pts',(27.4243822495492,-3.7974415432656,3.59166085841746));
#73394=CARTESIAN_POINT('Ctrl Pts',(27.4641375736882,-4.49391018137497,2.10427722634554));
#73395=CARTESIAN_POINT('Ctrl Pts',(27.4815621450774,-4.79916910625851,1.45236398349203));
#73396=CARTESIAN_POINT('Ctrl Pts',(27.4989867164666,-4.94848848074252,0.72743191486131));
#73397=CARTESIAN_POINT('Ctrl Pts',(27.5164112878558,-4.94632349813665,0.00165195671278186));
#73398=CARTESIAN_POINT('Origin',(10.45,0.,0.));
#73399=CARTESIAN_POINT('',(28.3717887121441,-4.95045814526779,-0.00419805499302928));
#73400=CARTESIAN_POINT('',(28.2664112878558,-4.95200672834798,-0.00447880390354169));
#73401=CARTESIAN_POINT('',(10.45,-4.954,-6.06690024297599E-16));
#73402=CARTESIAN_POINT('Ctrl Pts',(28.3717887121441,-4.95045814526779,-0.00419805499302928));
#73403=CARTESIAN_POINT('Ctrl Pts',(28.344234598804,-4.9412870202373,1.14109909159698));
#73404=CARTESIAN_POINT('Ctrl Pts',(28.3166804854639,-4.54589945079795,2.29210988530882));
#73405=CARTESIAN_POINT('Ctrl Pts',(28.2891263721238,-3.81911859406739,3.16820830363733));
#73406=CARTESIAN_POINT('Ctrl Pts',(28.2493710479848,-2.77051259536383,4.43225103179432));
#73407=CARTESIAN_POINT('Ctrl Pts',(28.2096157238457,-1.03204586664494,5.12400922901711));
#73408=CARTESIAN_POINT('Ctrl Pts',(28.1698603997067,0.598340523580153,4.92597191512799));
#73409=CARTESIAN_POINT('Ctrl Pts',(28.1301050755676,2.22872691380516,4.72793460123887));
#73410=CARTESIAN_POINT('Ctrl Pts',(28.0903497514285,3.75103296553638,3.64010177623793));
#73411=CARTESIAN_POINT('Ctrl Pts',(28.0505944272895,4.46653347601348,2.16177922055856));
#73412=CARTESIAN_POINT('Ctrl Pts',(28.0108391031504,5.18203398649057,0.683456664879198));
#73413=CARTESIAN_POINT('Ctrl Pts',(27.9710837790114,5.09072895571354,-1.18535562147859));
#73414=CARTESIAN_POINT('Ctrl Pts',(27.9313284548724,4.23452659660065,-2.58688909570347));
#73415=CARTESIAN_POINT('Ctrl Pts',(27.8915731307333,3.37832423748771,-3.98842256992843));
#73416=CARTESIAN_POINT('Ctrl Pts',(27.8518178065942,1.75722455003883,-4.92267723202043));
#73417=CARTESIAN_POINT('Ctrl Pts',(27.8120624824552,0.115298154297456,-4.96083833907168));
#73418=CARTESIAN_POINT('Ctrl Pts',(27.7723071583161,-1.52662824144383,-4.99899944612293));
#73419=CARTESIAN_POINT('Ctrl Pts',(27.7325518341771,-3.18938134547761,-4.14106699813353));
#73420=CARTESIAN_POINT('Ctrl Pts',(27.692796510038,-4.10977198277882,-2.78082450729169));
#73421=CARTESIAN_POINT('Ctrl Pts',(27.6691272440734,-4.65774816603,-1.97097219217775));
#73422=CARTESIAN_POINT('Ctrl Pts',(27.6454579781088,-4.94257943067843,-0.983066242534685));
#73423=CARTESIAN_POINT('Ctrl Pts',(27.6217887121441,-4.94702083875962,0.0024746876873416));
#73424=CARTESIAN_POINT('Ctrl Pts',(27.5164112878558,-4.94632349813665,0.00165195671278186));
#73425=CARTESIAN_POINT('Ctrl Pts',(27.5387420406057,-4.94354892823764,-0.928483564797916));
#73426=CARTESIAN_POINT('Ctrl Pts',(27.5610727933555,-4.69197439851418,-1.86001167153667));
#73427=CARTESIAN_POINT('Ctrl Pts',(27.5834035461053,-4.20097747928438,-2.64102245013698));
#73428=CARTESIAN_POINT('Ctrl Pts',(27.6231588702444,-3.32685819213247,-4.03145191783911));
#73429=CARTESIAN_POINT('Ctrl Pts',(27.6629141943835,-1.69390167087667,-4.94482427653488));
#73430=CARTESIAN_POINT('Ctrl Pts',(27.7026695185225,-0.0516207188824688,
-4.96190957847522));
#73431=CARTESIAN_POINT('Ctrl Pts',(27.7424248426616,1.59066023311174,-4.97899488041556));
#73432=CARTESIAN_POINT('Ctrl Pts',(27.7821801668006,3.24226561584435,-4.09979312560047));
#73433=CARTESIAN_POINT('Ctrl Pts',(27.8219354909397,4.14512296115597,-2.72785025257614));
#73434=CARTESIAN_POINT('Ctrl Pts',(27.8616908150787,5.04798030646763,-1.35590737955174));
#73435=CARTESIAN_POINT('Ctrl Pts',(27.9014461392178,5.20208961435818,0.508776611681977));
#73436=CARTESIAN_POINT('Ctrl Pts',(27.9412014633569,4.53671605638716,2.01032802977551));
#73437=CARTESIAN_POINT('Ctrl Pts',(27.9809567874959,3.87134249841618,3.51187944786895));
#73438=CARTESIAN_POINT('Ctrl Pts',(28.020712111635,2.38648607458373,4.65029829282225));
#73439=CARTESIAN_POINT('Ctrl Pts',(28.060467435774,0.76368293501706,4.90306024216977));
#73440=CARTESIAN_POINT('Ctrl Pts',(28.1002227599131,-0.859120204549604,
5.15582219151729));
#73441=CARTESIAN_POINT('Ctrl Pts',(28.1399780840521,-2.61987005985048,4.52292724525903));
#73442=CARTESIAN_POINT('Ctrl Pts',(28.1797334081912,-3.71039780159122,3.29486866468593));
#73443=CARTESIAN_POINT('Ctrl Pts',(28.2086260347461,-4.50295103747106,2.40236335314786));
#73444=CARTESIAN_POINT('Ctrl Pts',(28.2375186613009,-4.9415051357895,1.19550342842609));
#73445=CARTESIAN_POINT('Ctrl Pts',(28.2664112878558,-4.95200672834798,-0.00447880390354169));
#73446=CARTESIAN_POINT('Origin',(10.45,0.,0.));
#73447=CARTESIAN_POINT('',(29.1217887121441,-4.9620979667096,-0.000568056217270518));
#73448=CARTESIAN_POINT('',(29.0164112878558,-4.96212320436852,0.000469511818217842));
#73449=CARTESIAN_POINT('',(10.45,-4.954,-6.06690024297599E-16));
#73450=CARTESIAN_POINT('Ctrl Pts',(29.1217887121441,-4.9620979667096,-0.000568056217270518));
#73451=CARTESIAN_POINT('Ctrl Pts',(29.0827665436384,-4.95948881461475,1.61158375926093));
#73452=CARTESIAN_POINT('Ctrl Pts',(29.0437443751326,-4.10050759025402,3.2261208355131));
#73453=CARTESIAN_POINT('Ctrl Pts',(29.0047222066268,-2.76101916288883,4.12310366992494));
#73454=CARTESIAN_POINT('Ctrl Pts',(28.9649668824878,-1.39636418215534,5.03693918175563));
#73455=CARTESIAN_POINT('Ctrl Pts',(28.9252115583487,0.467023332900544,5.20600407764322));
#73456=CARTESIAN_POINT('Ctrl Pts',(28.8854562342097,1.9738647621892,4.55269904467401));
#73457=CARTESIAN_POINT('Ctrl Pts',(28.8457009100706,3.48070619147776,3.89939401170483));
#73458=CARTESIAN_POINT('Ctrl Pts',(28.8059455859316,4.63100153499924,2.42371904987888));
#73459=CARTESIAN_POINT('Ctrl Pts',(28.7661902617925,4.89677526101191,0.802996098327756));
#73460=CARTESIAN_POINT('Ctrl Pts',(28.7264349376535,5.1625489870246,-0.817726853223465));
#73461=CARTESIAN_POINT('Ctrl Pts',(28.6866796135144,4.54380109552853,-2.58349779449976));
#73462=CARTESIAN_POINT('Ctrl Pts',(28.6469242893753,3.32453147304543,-3.68384326152976));
#73463=CARTESIAN_POINT('Ctrl Pts',(28.6071689652363,2.10526185056232,-4.78418872855976));
#73464=CARTESIAN_POINT('Ctrl Pts',(28.5674136410972,0.285470497092144,-5.21910872134327));
#73465=CARTESIAN_POINT('Ctrl Pts',(28.5276583169582,-1.29957422527118,-4.7889787558308));
#73466=CARTESIAN_POINT('Ctrl Pts',(28.4879029928191,-2.88461894763441,-4.35884879031834));
#73467=CARTESIAN_POINT('Ctrl Pts',(28.4481476686801,-4.23491703889091,-3.06366886650999));
#73468=CARTESIAN_POINT('Ctrl Pts',(28.408392344541,-4.73069345017502,-1.49791527506032));
#73469=CARTESIAN_POINT('Ctrl Pts',(28.396191133742,-4.88285099471092,-1.0173736107117));
#73470=CARTESIAN_POINT('Ctrl Pts',(28.3839899229431,-4.9545192024457,-0.511345998405597));
#73471=CARTESIAN_POINT('Ctrl Pts',(28.3717887121441,-4.95045814526779,-0.00419805499302928));
#73472=CARTESIAN_POINT('Ctrl Pts',(28.2664112878558,-4.95200672834798,-0.00447880390354169));
#73473=CARTESIAN_POINT('Ctrl Pts',(28.27727398544,-4.95595498912304,-0.455633498040154));
#73474=CARTESIAN_POINT('Ctrl Pts',(28.2881366830242,-4.89939725962342,-0.905816018007978));
#73475=CARTESIAN_POINT('Ctrl Pts',(28.2989993806083,-4.77839806799436,-1.33795488241193));
#73476=CARTESIAN_POINT('Ctrl Pts',(28.3387547047474,-4.33556496447621,-2.9194976340483));
#73477=CARTESIAN_POINT('Ctrl Pts',(28.3785100288864,-3.02959312925948,-4.25936092243318));
#73478=CARTESIAN_POINT('Ctrl Pts',(28.4182653530255,-1.4599122462263,-4.74255918222436));
#73479=CARTESIAN_POINT('Ctrl Pts',(28.4580206771646,0.109768636807045,-5.22575744201559));
#73480=CARTESIAN_POINT('Ctrl Pts',(28.4977760013036,1.94315856765701,-4.85229067321291));
#73481=CARTESIAN_POINT('Ctrl Pts',(28.5375313254427,3.19874755579615,-3.7935768659499));
#73482=CARTESIAN_POINT('Ctrl Pts',(28.5772866495817,4.4543365439353,-2.7348630586869));
#73483=CARTESIAN_POINT('Ctrl Pts',(28.6170419737208,5.13212458936373,-0.990902212963525));
#73484=CARTESIAN_POINT('Ctrl Pts',(28.6567972978598,4.92101288975318,0.637842850916404));
#73485=CARTESIAN_POINT('Ctrl Pts',(28.6965526219989,4.70990119014265,2.26658791479624));
#73486=CARTESIAN_POINT('Ctrl Pts',(28.7363079461379,3.60988974549346,3.78011719683246));
#73487=CARTESIAN_POINT('Ctrl Pts',(28.776063270277,2.12587421645596,4.48373395501895));
#73488=CARTESIAN_POINT('Ctrl Pts',(28.815818594416,0.641858687418374,5.18735071320548));
#73489=CARTESIAN_POINT('Ctrl Pts',(28.8555739185551,-1.22616092600755,5.08105494754191));
#73490=CARTESIAN_POINT('Ctrl Pts',(28.8953292426942,-2.62077991097366,4.21363548753556));
#73491=CARTESIAN_POINT('Ctrl Pts',(28.9350845668332,-4.0153988959397,3.34621602752926));
#73492=CARTESIAN_POINT('Ctrl Pts',(28.9748398909723,-4.93661725244607,1.71767287318022));
#73493=CARTESIAN_POINT('Ctrl Pts',(29.0145952151113,-4.96160378816815,0.0754931309297103));
#73494=CARTESIAN_POINT('Ctrl Pts',(29.0152005726928,-4.96198426019705,0.0504875252986975));
#73495=CARTESIAN_POINT('Ctrl Pts',(29.0158059302743,-4.96215692830693,0.0254787578334992));
#73496=CARTESIAN_POINT('Ctrl Pts',(29.0164112878558,-4.96212320436852,0.000469511818217842));
#73497=CARTESIAN_POINT('Origin',(10.45,0.,0.));
#73498=CARTESIAN_POINT('',(29.8717887121441,-4.95216086653923,0.0044958085145208));
#73499=CARTESIAN_POINT('',(29.7664112878558,-4.95060002325747,0.00423272256442855));
#73500=CARTESIAN_POINT('',(10.45,-4.954,-6.06690024297599E-16));
#73501=CARTESIAN_POINT('Ctrl Pts',(29.8717887121441,-4.95216086653923,0.0044958085145208));
#73502=CARTESIAN_POINT('Ctrl Pts',(29.8610538126118,-4.95608712658793,0.450307475266639));
#73503=CARTESIAN_POINT('Ctrl Pts',(29.8503189130794,-4.90087411902633,0.895163507848311));
#73504=CARTESIAN_POINT('Ctrl Pts',(29.839584013547,-4.78267074519706,1.32260017912596));
#73505=CARTESIAN_POINT('Ctrl Pts',(29.7998286894079,-4.34491970460876,2.90555709123284));
#73506=CARTESIAN_POINT('Ctrl Pts',(29.7600733652689,-3.04325814371637,4.24960811376942));
#73507=CARTESIAN_POINT('Ctrl Pts',(29.7203180411298,-1.47513736807399,4.73784554793628));
#73508=CARTESIAN_POINT('Ctrl Pts',(29.6805627169907,0.0929834075686548,
5.22608298210322));
#73509=CARTESIAN_POINT('Ctrl Pts',(29.6408073928517,1.9275633979613,4.85850682790008));
#73510=CARTESIAN_POINT('Ctrl Pts',(29.6010520687127,3.18654638562424,3.80383133472726));
#73511=CARTESIAN_POINT('Ctrl Pts',(29.5612967445736,4.44552937328696,2.74915584155461));
#73512=CARTESIAN_POINT('Ctrl Pts',(29.5215414204345,5.12891535822014,1.0073810094123));
#73513=CARTESIAN_POINT('Ctrl Pts',(29.4817860962955,4.92303613267859,-0.622033702566684));
#73514=CARTESIAN_POINT('Ctrl Pts',(29.4420307721564,4.71715690713703,-2.25144841454585));
#73515=CARTESIAN_POINT('Ctrl Pts',(29.4022754480174,3.62201247112069,-3.76850300636179));
#73516=CARTESIAN_POINT('Ctrl Pts',(29.3625201238783,2.1402645707595,-4.47688264956091));
#73517=CARTESIAN_POINT('Ctrl Pts',(29.3227647997393,0.658516670398306,-5.18526229276003));
#73518=CARTESIAN_POINT('Ctrl Pts',(29.2830094756002,-1.20983469430763,-5.08496698734232));
#73519=CARTESIAN_POINT('Ctrl Pts',(29.2432541514611,-2.60723253956581,-4.22203140388807));
#73520=CARTESIAN_POINT('Ctrl Pts',(29.2034988273221,-4.00463038482382,-3.35909582043393));
#73521=CARTESIAN_POINT('Ctrl Pts',(29.163743503183,-4.93107471063413,-1.73351995894351));
#73522=CARTESIAN_POINT('Ctrl Pts',(29.123988179044,-4.96133565033377,-0.0914289643114814));
#73523=CARTESIAN_POINT('Ctrl Pts',(29.1232550234107,-4.96189371340808,-0.0611460200982296));
#73524=CARTESIAN_POINT('Ctrl Pts',(29.1225218677774,-4.96214698793598,-0.0308574591512815));
#73525=CARTESIAN_POINT('Ctrl Pts',(29.1217887121441,-4.9620979667096,-0.000568056217270518));
#73526=CARTESIAN_POINT('Ctrl Pts',(29.0164112878558,-4.96212320436852,0.000469511818217842));
#73527=CARTESIAN_POINT('Ctrl Pts',(29.0555612544134,-4.95994219416689,-1.61694005742288));
#73528=CARTESIAN_POINT('Ctrl Pts',(29.0947112209709,-4.09452073852457,-3.2363511756137));
#73529=CARTESIAN_POINT('Ctrl Pts',(29.1338611875285,-2.7477619212938,-4.13195060322239));
#73530=CARTESIAN_POINT('Ctrl Pts',(29.1736165116676,-1.38017880375977,-5.04139826497171));
#73531=CARTESIAN_POINT('Ctrl Pts',(29.2133718358066,0.483742146245983,-5.20447725831835));
#73532=CARTESIAN_POINT('Ctrl Pts',(29.2531271599456,1.98847746664373,-4.54633574741596));
#73533=CARTESIAN_POINT('Ctrl Pts',(29.2928824840847,3.49321278704156,-3.88819423651354));
#73534=CARTESIAN_POINT('Ctrl Pts',(29.3326378082238,4.63876247783135,-2.408832221362));
#73535=CARTESIAN_POINT('Ctrl Pts',(29.3723931323628,4.89932922049166,-0.787263966417092));
#73536=CARTESIAN_POINT('Ctrl Pts',(29.4121484565019,5.15989596315194,0.834304288527634));
#73537=CARTESIAN_POINT('Ctrl Pts',(29.4519037806409,4.53547975768294,2.5980787832657));
#73538=CARTESIAN_POINT('Ctrl Pts',(29.49165910478,3.31268219729058,3.69450240537696));
#73539=CARTESIAN_POINT('Ctrl Pts',(29.531414428919,2.08988463689801,4.79092602748841));
#73540=CARTESIAN_POINT('Ctrl Pts',(29.5711697530581,0.268705721581839,5.21999877697279));
#73541=CARTESIAN_POINT('Ctrl Pts',(29.6109250771972,-1.31494930777667,4.78478000346513));
#73542=CARTESIAN_POINT('Ctrl Pts',(29.6506804013362,-2.89860433713499,4.34956122995753));
#73543=CARTESIAN_POINT('Ctrl Pts',(29.6904357254753,-4.24473548053571,3.05005093345812));
#73544=CARTESIAN_POINT('Ctrl Pts',(29.7301910496143,-4.73548028184195,1.48271300792442));
#73545=CARTESIAN_POINT('Ctrl Pts',(29.7422644623615,-4.88451603159391,1.00672348704749));
#73546=CARTESIAN_POINT('Ctrl Pts',(29.7543378751087,-4.95465999137664,0.506032378106856));
#73547=CARTESIAN_POINT('Ctrl Pts',(29.7664112878558,-4.95060002325747,0.00423272256442855));
#73548=CARTESIAN_POINT('Origin',(10.45,0.,0.));
#73549=CARTESIAN_POINT('',(30.6217887121441,-4.94627182265837,-0.00156944476627563));
#73550=CARTESIAN_POINT('',(30.5164112878558,-4.94694225394907,-0.00239988756266602));
#73551=CARTESIAN_POINT('',(10.45,-4.954,-6.06690024297599E-16));
#73552=CARTESIAN_POINT('Ctrl Pts',(30.6217887121441,-4.94627182265837,-0.00156944476627563));
#73553=CARTESIAN_POINT('Ctrl Pts',(30.5995857574461,-4.94365246685677,0.923267018668746));
#73554=CARTESIAN_POINT('Ctrl Pts',(30.577382802748,-4.69512873603121,1.84941055057953));
#73555=CARTESIAN_POINT('Ctrl Pts',(30.55517984805,-4.20943847831249,2.62751563041785));
#73556=CARTESIAN_POINT('Ctrl Pts',(30.5154245239109,-3.33978964601186,4.02074549932014));
#73557=CARTESIAN_POINT('Ctrl Pts',(30.4756691997719,-1.70977523980265,4.93935804323487));
#73558=CARTESIAN_POINT('Ctrl Pts',(30.4359138756328,-0.0675576579001141,
4.96171811509349));
#73559=CARTESIAN_POINT('Ctrl Pts',(30.3961585514937,1.57465992400252,4.98407818695211));
#73560=CARTESIAN_POINT('Ctrl Pts',(30.3564032273547,3.22908068159848,4.11018578675453));
#73561=CARTESIAN_POINT('Ctrl Pts',(30.3166479032156,4.13633991421696,2.74114990557676));
#73562=CARTESIAN_POINT('Ctrl Pts',(30.2768925790766,5.04359914683538,1.37211402439907));
#73563=CARTESIAN_POINT('Ctrl Pts',(30.2371372549375,5.2036968544764,-0.492065337758739));
#73564=CARTESIAN_POINT('Ctrl Pts',(30.1973819307985,4.54314958543481,-1.99574610989259));
#73565=CARTESIAN_POINT('Ctrl Pts',(30.1576266066594,3.88260231639321,-3.49942688202644));
#73566=CARTESIAN_POINT('Ctrl Pts',(30.1178712825204,2.40141007066901,-4.64260906413632));
#73567=CARTESIAN_POINT('Ctrl Pts',(30.0781159583813,0.779427172590541,-4.90058200353951));
#73568=CARTESIAN_POINT('Ctrl Pts',(30.0383606342423,-0.842555725488016,
-5.15855494294273));
#73569=CARTESIAN_POINT('Ctrl Pts',(29.9986053101032,-2.60532927592085,-4.53131863963915));
#73570=CARTESIAN_POINT('Ctrl Pts',(29.9588499859641,-3.6997957909952,-3.30676908714867));
#73571=CARTESIAN_POINT('Ctrl Pts',(29.9298295613575,-4.49872986267182,-2.41287754595835));
#73572=CARTESIAN_POINT('Ctrl Pts',(29.9008091367508,-4.9415467258679,-1.20069887679431));
#73573=CARTESIAN_POINT('Ctrl Pts',(29.8717887121441,-4.95216086653923,0.0044958085145208));
#73574=CARTESIAN_POINT('Ctrl Pts',(29.7664112878558,-4.95060002325747,0.00423272256442855));
#73575=CARTESIAN_POINT('Ctrl Pts',(29.7940931992477,-4.94129133149963,-1.14629313885498));
#73576=CARTESIAN_POINT('Ctrl Pts',(29.8217751106396,-4.54189791215148,-2.30264655026279));
#73577=CARTESIAN_POINT('Ctrl Pts',(29.8494570220315,-3.80892294691085,-3.18045866944975));
#73578=CARTESIAN_POINT('Ctrl Pts',(29.8892123461705,-2.75626235146179,-4.44112686672221));
#73579=CARTESIAN_POINT('Ctrl Pts',(29.9289676703096,-1.01558270135191,-5.12729770669915));
#73580=CARTESIAN_POINT('Ctrl Pts',(29.9687229944486,0.614159223288633,-4.92402475745519));
#73581=CARTESIAN_POINT('Ctrl Pts',(30.0084783185877,2.24390114792926,-4.72075180821122));
#73582=CARTESIAN_POINT('Ctrl Pts',(30.0482336427267,3.76270534710054,-3.62803506974627));
#73583=CARTESIAN_POINT('Ctrl Pts',(30.0879889668658,4.47345393782982,-2.1474219961845));
#73584=CARTESIAN_POINT('Ctrl Pts',(30.1277442910049,5.18420252855906,-0.666808922622812));
#73585=CARTESIAN_POINT('Ctrl Pts',(30.1674996151439,5.0868955108464,1.20170048603564));
#73586=CARTESIAN_POINT('Ctrl Pts',(30.207254939283,4.22619595727435,2.60047670520234));
#73587=CARTESIAN_POINT('Ctrl Pts',(30.247010263422,3.36549640370231,3.99925292436904));
#73588=CARTESIAN_POINT('Ctrl Pts',(30.2867655875611,1.74140431427089,4.92829595404398));
#73589=CARTESIAN_POINT('Ctrl Pts',(30.3265209117001,0.0993637954387848,
4.96118314515178));
#73590=CARTESIAN_POINT('Ctrl Pts',(30.3662762358392,-1.54267672339342,4.99407033625959));
#73591=CARTESIAN_POINT('Ctrl Pts',(30.4060315599783,-3.20266567162631,4.13080168880015));
#73592=CARTESIAN_POINT('Ctrl Pts',(30.4457868841173,-4.11868259764308,2.76760998398513));
#73593=CARTESIAN_POINT('Ctrl Pts',(30.4693283520301,-4.66111014762382,1.96038392123949));
#73594=CARTESIAN_POINT('Ctrl Pts',(30.492869819943,-4.94266232326109,0.97785877353352));
#73595=CARTESIAN_POINT('Ctrl Pts',(30.5164112878558,-4.94694225394907,-0.00239988756266602));
#73596=CARTESIAN_POINT('Origin',(10.45,0.,0.));
#73597=CARTESIAN_POINT('',(31.3717887121441,-4.95793233061953,-0.00387638962322745));
#73598=CARTESIAN_POINT('',(31.2664112878558,-4.9594059793847,-0.00326224302469192));
#73599=CARTESIAN_POINT('',(10.45,-4.954,-6.06690024297599E-16));
#73600=CARTESIAN_POINT('Ctrl Pts',(31.3717887121441,-4.95793233061953,-0.00387638962322745));
#73601=CARTESIAN_POINT('Ctrl Pts',(31.3381177022804,-4.94594313351065,1.39027847680682));
#73602=CARTESIAN_POINT('Ctrl Pts',(31.3044466924167,-4.33051759246278,2.7936983782844));
#73603=CARTESIAN_POINT('Ctrl Pts',(31.270775682553,-3.28893015515837,3.71566267646537));
#73604=CARTESIAN_POINT('Ctrl Pts',(31.2310203584139,-2.05912901890516,4.80422490454117));
#73605=CARTESIAN_POINT('Ctrl Pts',(31.1912650342748,-0.2352369420535,5.22161400632066));
#73606=CARTESIAN_POINT('Ctrl Pts',(31.1515097101358,1.34559551703039,4.77625202385045));
#73607=CARTESIAN_POINT('Ctrl Pts',(31.1117543859967,2.92642797611456,4.33089004138017));
#73608=CARTESIAN_POINT('Ctrl Pts',(31.0719990618577,4.26420081743087,3.02277697465984));
#73609=CARTESIAN_POINT('Ctrl Pts',(31.0322437377186,4.74488797261209,1.45232531415967));
#73610=CARTESIAN_POINT('Ctrl Pts',(30.9924884135796,5.22557512779325,-0.118126346340324));
#73611=CARTESIAN_POINT('Ctrl Pts',(30.9527330894405,4.84917659683952,-1.9509166006201));
#73612=CARTESIAN_POINT('Ctrl Pts',(30.9129777653015,3.78845602314589,-3.20481070446875));
#73613=CARTESIAN_POINT('Ctrl Pts',(30.8732224411624,2.72773544945226,-4.4587048083174));
#73614=CARTESIAN_POINT('Ctrl Pts',(30.8334671170233,0.982692833018733,-5.13370276173493));
#73615=CARTESIAN_POINT('Ctrl Pts',(30.7937117928843,-0.645712482528409,
-4.91998639029569));
#73616=CARTESIAN_POINT('Ctrl Pts',(30.7539564687452,-2.27411779807564,-4.70627001885644));
#73617=CARTESIAN_POINT('Ctrl Pts',(30.7142011446062,-3.78588581273648,-3.60383932256033));
#73618=CARTESIAN_POINT('Ctrl Pts',(30.6744458204671,-4.48712819087084,-2.11870037746728));
#73619=CARTESIAN_POINT('Ctrl Pts',(30.6568934510261,-4.79673364763043,-1.46299682077366));
#73620=CARTESIAN_POINT('Ctrl Pts',(30.6393410815851,-4.94834253357735,-0.73269156339755));
#73621=CARTESIAN_POINT('Ctrl Pts',(30.6217887121441,-4.94627182265837,-0.00156944476627563));
#73622=CARTESIAN_POINT('Ctrl Pts',(30.5164112878558,-4.94694225394907,-0.00239988756266602));
#73623=CARTESIAN_POINT('Ctrl Pts',(30.532625144082,-4.94988999625171,-0.67753930768575));
#73624=CARTESIAN_POINT('Ctrl Pts',(30.5488390003082,-4.82131163479957,-1.35160360341962));
#73625=CARTESIAN_POINT('Ctrl Pts',(30.5650528565345,-4.55585019848591,-1.96658087363273));
#73626=CARTESIAN_POINT('Ctrl Pts',(30.6048081806735,-3.90495596951134,-3.47446526426518));
#73627=CARTESIAN_POINT('Ctrl Pts',(30.6445635048126,-2.43112260776153,-4.62711928335961));
#73628=CARTESIAN_POINT('Ctrl Pts',(30.6843188289516,-0.810826773992338,
-4.89548478765477));
#73629=CARTESIAN_POINT('Ctrl Pts',(30.7240741530907,0.809469059776941,-5.16385029194995));
#73630=CARTESIAN_POINT('Ctrl Pts',(30.7638294772297,2.57622736556561,-4.54792728144577));
#73631=CARTESIAN_POINT('Ctrl Pts',(30.8035848013688,3.6785214877009,-3.33041904692261));
#73632=CARTESIAN_POINT('Ctrl Pts',(30.8433401255079,4.78081560983612,-2.11291081239953));
#73633=CARTESIAN_POINT('Ctrl Pts',(30.8830954496469,5.21864554831803,-0.29381735385755));
#73634=CARTESIAN_POINT('Ctrl Pts',(30.9228507737859,4.79105117939728,1.29191329429574));
#73635=CARTESIAN_POINT('Ctrl Pts',(30.962606097925,4.36345681047652,2.87764394244903));
#73636=CARTESIAN_POINT('Ctrl Pts',(31.0023614220641,3.07043813415308,4.23001178021363));
#73637=CARTESIAN_POINT('Ctrl Pts',(31.0421167462031,1.50547944733267,4.72829176312557));
#73638=CARTESIAN_POINT('Ctrl Pts',(31.0818720703422,-0.0594792394878271,
5.22657174603753));
#73639=CARTESIAN_POINT('Ctrl Pts',(31.1216273944812,-1.89637793680533,4.87076387409672));
#73640=CARTESIAN_POINT('Ctrl Pts',(31.1613827186203,-3.16209616088146,3.82418085776822));
#73641=CARTESIAN_POINT('Ctrl Pts',(31.1963922416988,-4.27671897773194,2.90253393230071));
#73642=CARTESIAN_POINT('Ctrl Pts',(31.2314017647773,-4.94839134831731,1.44519089534153));
#73643=CARTESIAN_POINT('Ctrl Pts',(31.2664112878558,-4.9594059793847,-0.00326224302469192));
#73644=CARTESIAN_POINT('Origin',(10.45,0.,0.));
#73645=CARTESIAN_POINT('',(32.1217887121441,-4.95872700410626,0.0035772032441482));
#73646=CARTESIAN_POINT('',(32.0164112878558,-4.95717366314325,0.00410403508777372));
#73647=CARTESIAN_POINT('',(10.45,-4.954,-6.06690024297599E-16));
#73648=CARTESIAN_POINT('Ctrl Pts',(32.1217887121441,-4.95872700410626,0.0035772032441482));
#73649=CARTESIAN_POINT('Ctrl Pts',(32.1164049712538,-4.96054007908593,0.226399070643231));
#73650=CARTESIAN_POINT('Ctrl Pts',(32.1110212303634,-4.94682528332486,0.448996398812498));
#73651=CARTESIAN_POINT('Ctrl Pts',(32.1056374894731,-4.9168227585756,0.669376315342024));
#73652=CARTESIAN_POINT('Ctrl Pts',(32.065882165334,-4.69527418840998,2.29673453963713));
#73653=CARTESIAN_POINT('Ctrl Pts',(32.026126841195,-3.58558275123426,3.80318098227819));
#73654=CARTESIAN_POINT('Ctrl Pts',(31.986371517056,-2.09708713985614,4.49726986277651));
#73655=CARTESIAN_POINT('Ctrl Pts',(31.9466161929169,-0.608591528478095,
5.19135874327479));
#73656=CARTESIAN_POINT('Ctrl Pts',(31.9068608687778,1.25870825710231,5.07309006163041));
#73657=CARTESIAN_POINT('Ctrl Pts',(31.8671055446388,2.64773789874118,4.19674811137832));
#73658=CARTESIAN_POINT('Ctrl Pts',(31.8273502204997,4.03676754038028,3.32040616112608));
#73659=CARTESIAN_POINT('Ctrl Pts',(31.7875948963607,4.94752703807765,1.68599094226582));
#73660=CARTESIAN_POINT('Ctrl Pts',(31.7478395722216,4.96198572449744,0.0436847876433137));
#73661=CARTESIAN_POINT('Ctrl Pts',(31.7080842480826,4.97644441091723,-1.59862136697901));
#73662=CARTESIAN_POINT('Ctrl Pts',(31.6683289239435,4.09460228605965,-3.24881845736358));
#73663=CARTESIAN_POINT('Ctrl Pts',(31.6285735998044,2.72121719529554,-4.14948040925797));
#73664=CARTESIAN_POINT('Ctrl Pts',(31.5888182756654,1.34783210453152,-5.05014236115231));
#73665=CARTESIAN_POINT('Ctrl Pts',(31.5490629515264,-0.517095952138985,
-5.20126917455656));
#73666=CARTESIAN_POINT('Ctrl Pts',(31.5093076273873,-2.01758125945948,-4.53349495999121));
#73667=CARTESIAN_POINT('Ctrl Pts',(31.4695523032482,-3.51806656678022,-3.86572074542575));
#73668=CARTESIAN_POINT('Ctrl Pts',(31.4297969791092,-4.65410912475082,-2.37904550289038));
#73669=CARTESIAN_POINT('Ctrl Pts',(31.3900416549701,-4.90427530590864,-0.755840204436467));
#73670=CARTESIAN_POINT('Ctrl Pts',(31.3839573406948,-4.94256174175555,-0.507418354456599));
#73671=CARTESIAN_POINT('Ctrl Pts',(31.3778730264194,-4.96009876528884,-0.255798633422028));
#73672=CARTESIAN_POINT('Ctrl Pts',(31.3717887121441,-4.95793233061953,-0.00387638962322745));
#73673=CARTESIAN_POINT('Ctrl Pts',(31.2664112878558,-4.9594059793847,-0.00326224302469192));
#73674=CARTESIAN_POINT('Ctrl Pts',(31.2711570889163,-4.96089909449181,-0.199610831515726));
#73675=CARTESIAN_POINT('Ctrl Pts',(31.2759028899769,-4.95025208354887,-0.395796060852635));
#73676=CARTESIAN_POINT('Ctrl Pts',(31.2806486910374,-4.92692264233869,-0.590461378916891));
#73677=CARTESIAN_POINT('Ctrl Pts',(31.3204040151765,-4.7314931488852,-2.22116243855789));
#73678=CARTESIAN_POINT('Ctrl Pts',(31.3601593393156,-3.64609641114327,-3.74520639712367));
#73679=CARTESIAN_POINT('Ctrl Pts',(31.3999146634546,-2.16892006673788,-4.46307036777193));
#73680=CARTESIAN_POINT('Ctrl Pts',(31.4396699875937,-0.691743722332493,
-5.18093433842019));
#73681=CARTESIAN_POINT('Ctrl Pts',(31.4794253117327,1.17721222873627,-5.09261832115089));
#73682=CARTESIAN_POINT('Ctrl Pts',(31.5191806358718,2.58011330280755,-4.23865859774737));
#73683=CARTESIAN_POINT('Ctrl Pts',(31.5589359600108,3.98301437687875,-3.38469887434389));
#73684=CARTESIAN_POINT('Ctrl Pts',(31.5986912841499,4.91986057395253,-1.76509544480606));
#73685=CARTESIAN_POINT('Ctrl Pts',(31.638446608289,4.96064765916329,-0.123232159844304));
#73686=CARTESIAN_POINT('Ctrl Pts',(31.678201932428,5.00143474437405,1.51863112511736));
#73687=CARTESIAN_POINT('Ctrl Pts',(31.717957256567,4.14616271772212,3.18275426550314));
#73688=CARTESIAN_POINT('Ctrl Pts',(31.7577125807061,2.7873939812014,4.10531925154967));
#73689=CARTESIAN_POINT('Ctrl Pts',(31.7974679048452,1.42862524468052,5.02788423759631));
#73690=CARTESIAN_POINT('Ctrl Pts',(31.8372232289842,-0.433640201709166,
5.20889106930347));
#73691=CARTESIAN_POINT('Ctrl Pts',(31.8769785531233,-1.94463875761121,4.56525918935371));
#73692=CARTESIAN_POINT('Ctrl Pts',(31.9167338772624,-3.45563731351326,3.92162730940394));
#73693=CARTESIAN_POINT('Ctrl Pts',(31.9564892014014,-4.61536897892758,2.45335671779726));
#73694=CARTESIAN_POINT('Ctrl Pts',(31.9962445255404,-4.89152703265136,0.834370812302948));
#73695=CARTESIAN_POINT('Ctrl Pts',(32.0029667796456,-4.93822278096961,0.560615412616595));
#73696=CARTESIAN_POINT('Ctrl Pts',(32.0096890337507,-4.95965569987392,0.282550813091737));
#73697=CARTESIAN_POINT('Ctrl Pts',(32.0164112878558,-4.95717366314325,0.00410403508777372));
#73698=CARTESIAN_POINT('Origin',(10.45,0.,0.));
#73699=CARTESIAN_POINT('',(32.8717887121441,-4.94658723177794,0.00201400887214764));
#73700=CARTESIAN_POINT('',(32.7664112878558,-4.94605458361617,0.00114969562655201));
#73701=CARTESIAN_POINT('',(10.45,-4.954,-6.06690024297599E-16));
#73702=CARTESIAN_POINT('Ctrl Pts',(32.8717887121441,-4.94658723177794,0.00201400887214764));
#73703=CARTESIAN_POINT('Ctrl Pts',(32.8549369160881,-4.94914770039353,0.70384286307377));
#73704=CARTESIAN_POINT('Ctrl Pts',(32.8380851200321,-4.80985358206998,1.4047015626472));
#73705=CARTESIAN_POINT('Ctrl Pts',(32.8212333239761,-4.52373539183098,2.03936970544422));
#73706=CARTESIAN_POINT('Ctrl Pts',(32.7814779998371,-3.84874968958156,3.53662481426251));
#73707=CARTESIAN_POINT('Ctrl Pts',(32.741722675698,-2.35662586424462,4.66550145063581));
#73708=CARTESIAN_POINT('Ctrl Pts',(32.7019673515589,-0.732235739864097,
4.90785508262556));
#73709=CARTESIAN_POINT('Ctrl Pts',(32.6622120274199,0.892154384516242,5.15020871461528));
#73710=CARTESIAN_POINT('Ctrl Pts',(32.6224567032808,2.64881080794023,4.5060393422217));
#73711=CARTESIAN_POINT('Ctrl Pts',(32.5827013791418,3.73144355064897,3.27101509001533));
#73712=CARTESIAN_POINT('Ctrl Pts',(32.5429460550027,4.81407629335783,2.03599083780882));
#73713=CARTESIAN_POINT('Ctrl Pts',(32.5031907308637,5.22268535535135,0.210111705789586));
#73714=CARTESIAN_POINT('Ctrl Pts',(32.4634354067246,4.76972274037325,-1.36855970668223));
#73715=CARTESIAN_POINT('Ctrl Pts',(32.4236800825855,4.31676012539514,-2.94723111915404));
#73716=CARTESIAN_POINT('Ctrl Pts',(32.3839247584465,3.00222583344523,-4.27869481207827));
#73717=CARTESIAN_POINT('Ctrl Pts',(32.3441694343074,1.42947964137902,-4.75182056118187));
#73718=CARTESIAN_POINT('Ctrl Pts',(32.3044141101684,-0.143266550687003,
-5.22494631028541));
#73719=CARTESIAN_POINT('Ctrl Pts',(32.2646587860293,-1.97422464286937,-4.83973411556855));
#73720=CARTESIAN_POINT('Ctrl Pts',(32.2249034618903,-3.22300083738286,-3.77299301523568));
#73721=CARTESIAN_POINT('Ctrl Pts',(32.1905318786416,-4.3026654070543,-2.85071200435332));
#73722=CARTESIAN_POINT('Ctrl Pts',(32.1561602953928,-4.9471517335148,-1.41899132688034));
#73723=CARTESIAN_POINT('Ctrl Pts',(32.1217887121441,-4.95872700410626,0.0035772032441482));
#73724=CARTESIAN_POINT('Ctrl Pts',(32.0164112878558,-4.95717366314325,0.00410403508777372));
#73725=CARTESIAN_POINT('Ctrl Pts',(32.0494443578897,-4.944976966638,-1.36417984330865));
#73726=CARTESIAN_POINT('Ctrl Pts',(32.0824774279237,-4.35529939531296,-2.74169228837345));
#73727=CARTESIAN_POINT('Ctrl Pts',(32.1155104979576,-3.34807880300487,-3.66245541849339));
#73728=CARTESIAN_POINT('Ctrl Pts',(32.1552658220967,-2.13588807760102,-4.77059452441411));
#73729=CARTESIAN_POINT('Ctrl Pts',(32.1950211462357,-0.31892218476007,-5.21717151687348));
#73730=CARTESIAN_POINT('Ctrl Pts',(32.2347764703748,1.26884737521433,-4.79721145062356));
#73731=CARTESIAN_POINT('Ctrl Pts',(32.2745317945138,2.85661693518855,-4.3772513843737));
#73732=CARTESIAN_POINT('Ctrl Pts',(32.3142871186529,4.2151901622961,-3.09075425941461));
#73733=CARTESIAN_POINT('Ctrl Pts',(32.3540424427919,4.72099379247748,-1.52821103744581));
#73734=CARTESIAN_POINT('Ctrl Pts',(32.393797766931,5.22679742265886,0.0343321845229944));
#73735=CARTESIAN_POINT('Ctrl Pts',(32.43355309107,4.87983145591409,1.87292150350164));
#73736=CARTESIAN_POINT('Ctrl Pts',(32.4733084152091,3.83935024532743,3.14366045515198));
#73737=CARTESIAN_POINT('Ctrl Pts',(32.5130637393482,2.79886903474065,4.41439940680247));
#73738=CARTESIAN_POINT('Ctrl Pts',(32.5528190634872,1.06487258031201,5.11728799112456));
#73739=CARTESIAN_POINT('Ctrl Pts',(32.5925743876263,-0.566749866366629,
4.92970647732251));
#73740=CARTESIAN_POINT('Ctrl Pts',(32.6323297117653,-2.198372313045,4.7421249635205));
#73741=CARTESIAN_POINT('Ctrl Pts',(32.6720850359044,-3.72762075197333,3.66407335159448));
#73742=CARTESIAN_POINT('Ctrl Pts',(32.7118403600434,-4.45258348520756,2.19036793047174));
#73743=CARTESIAN_POINT('Ctrl Pts',(32.7300306693142,-4.78429493802344,1.51606435064163));
#73744=CARTESIAN_POINT('Ctrl Pts',(32.748220978585,-4.94762274111771,0.758927479174985));
#73745=CARTESIAN_POINT('Ctrl Pts',(32.7664112878558,-4.94605458361617,0.00114969562655201));
#73746=CARTESIAN_POINT('Origin',(10.45,0.,0.));
#73747=CARTESIAN_POINT('',(33.6217887121441,-4.9513279518383,-0.00438127959876189));
#73748=CARTESIAN_POINT('',(33.5164112878558,-4.95294315282494,-0.00455417533769269));
#73749=CARTESIAN_POINT('',(10.45,-4.954,-6.06690024297599E-16));
#73750=CARTESIAN_POINT('Ctrl Pts',(33.6217887121441,-4.9513279518383,-0.00438127959876189));
#73751=CARTESIAN_POINT('Ctrl Pts',(33.5934688609224,-4.94136392358352,1.17222104474813));
#73752=CARTESIAN_POINT('Ctrl Pts',(33.5651490097007,-4.5216107651878,2.35521240637459));
#73753=CARTESIAN_POINT('Ctrl Pts',(33.5368291584791,-3.75744266893846,3.24111636329651));
#73754=CARTESIAN_POINT('Ctrl Pts',(33.49707383434,-2.6847057352125,4.48474574142488));
#73755=CARTESIAN_POINT('Ctrl Pts',(33.457318510201,-0.933248809232052,5.14292095116953));
#73756=CARTESIAN_POINT('Ctrl Pts',(33.4175631860619,0.693024653229394,4.9135453107511));
#73757=CARTESIAN_POINT('Ctrl Pts',(33.3778078619229,2.31929811569066,4.68416967033269));
#73758=CARTESIAN_POINT('Ctrl Pts',(33.3380525377838,3.82038811463306,3.56724317975119));
#73759=CARTESIAN_POINT('Ctrl Pts',(33.2982972136447,4.50730743051541,2.07542535823586));
#73760=CARTESIAN_POINT('Ctrl Pts',(33.2585418895057,5.19422674639788,0.583607536720267));
#73761=CARTESIAN_POINT('Ctrl Pts',(33.2187865653666,5.06697537922034,-1.28310161572913));
#73762=CARTESIAN_POINT('Ctrl Pts',(33.1790312412276,4.18396059684558,-2.6678988764253));
#73763=CARTESIAN_POINT('Ctrl Pts',(33.1392759170885,3.30094581447098,-4.05269613712124));
#73764=CARTESIAN_POINT('Ctrl Pts',(33.0995205929495,1.66216761689915,-4.95558150606392));
#73765=CARTESIAN_POINT('Ctrl Pts',(33.0597652688104,0.0198109061580776,
-4.96213847235091));
#73766=CARTESIAN_POINT('Ctrl Pts',(33.0200099446714,-1.62254580458299,-4.9686954386379));
#73767=CARTESIAN_POINT('Ctrl Pts',(32.9802546205323,-3.26848102849344,-4.07892400226939));
#73768=CARTESIAN_POINT('Ctrl Pts',(32.9404992963932,-4.16252485086781,-2.70122149345361));
#73769=CARTESIAN_POINT('Ctrl Pts',(32.9175957683102,-4.67759442297352,-1.90751024133607));
#73770=CARTESIAN_POINT('Ctrl Pts',(32.8946922402272,-4.94310726058389,-0.951852084585827));
#73771=CARTESIAN_POINT('Ctrl Pts',(32.8717887121441,-4.94658723177794,0.00201400887214764));
#73772=CARTESIAN_POINT('Ctrl Pts',(32.7664112878558,-4.94605458361617,0.00114969562655201));
#73773=CARTESIAN_POINT('Ctrl Pts',(32.7879763027241,-4.94419549813648,-0.897212664561465));
#73774=CARTESIAN_POINT('Ctrl Pts',(32.8095413175923,-4.71058127270834,-1.7964758028442));
#73775=CARTESIAN_POINT('Ctrl Pts',(32.8311063324606,-4.25102312046575,-2.55969017516725));
#73776=CARTESIAN_POINT('Ctrl Pts',(32.8708616565997,-3.40382299494956,-3.96668362936352));
#73777=CARTESIAN_POINT('Ctrl Pts',(32.9106169807387,-1.78874571637721,-4.91131130743615));
#73778=CARTESIAN_POINT('Ctrl Pts',(32.9503723048778,-0.147097671634971,
-4.95999734259825));
#73779=CARTESIAN_POINT('Ctrl Pts',(32.9901276290168,1.49455037310708,-5.00868337776036));
#73780=CARTESIAN_POINT('Ctrl Pts',(33.0298829531559,3.16276918401907,-4.16142777001195));
#73781=CARTESIAN_POINT('Ctrl Pts',(33.0696382772949,4.09186087428128,-2.80711345497616));
#73782=CARTESIAN_POINT('Ctrl Pts',(33.109393601434,5.02095256454354,-1.45279913994028));
#73783=CARTESIAN_POINT('Ctrl Pts',(33.149148925573,5.21091713415614,0.408573882383032));
#73784=CARTESIAN_POINT('Ctrl Pts',(33.1889042497121,4.57456250221729,1.92265162650169));
#73785=CARTESIAN_POINT('Ctrl Pts',(33.2286595738511,3.93820787027841,3.43672937062043));
#73786=CARTESIAN_POINT('Ctrl Pts',(33.2684148979902,2.47553403678802,4.60351183653435));
#73787=CARTESIAN_POINT('Ctrl Pts',(33.3081702221293,0.857895536345488,4.88745604709655));
#73788=CARTESIAN_POINT('Ctrl Pts',(33.3479255462683,-0.759742964096859,
5.17140025765872));
#73789=CARTESIAN_POINT('Ctrl Pts',(33.3876808704074,-2.53234613149147,4.57250621286921));
#73790=CARTESIAN_POINT('Ctrl Pts',(33.4274361945464,-3.64630456965725,3.36566105674335));
#73791=CARTESIAN_POINT('Ctrl Pts',(33.4570945589829,-4.47734257630615,2.46532747290505));
#73792=CARTESIAN_POINT('Ctrl Pts',(33.4867529234193,-4.94181218791447,1.22663900174132));
#73793=CARTESIAN_POINT('Ctrl Pts',(33.5164112878558,-4.95294315282494,-0.00455417533769269));
#73794=CARTESIAN_POINT('Origin',(10.45,0.,0.));
#73795=CARTESIAN_POINT('',(34.3717887121441,-4.96217785588676,2.53259700289598E-5));
#73796=CARTESIAN_POINT('',(34.2664112878558,-4.96190593350399,0.00105408447129014));
#73797=CARTESIAN_POINT('',(10.45,-4.954,-6.06690024297599E-16));
#73798=CARTESIAN_POINT('Ctrl Pts',(34.3717887121441,-4.96217785588676,2.53259700289598E-5));
#73799=CARTESIAN_POINT('Ctrl Pts',(34.3320008057567,-4.96230199391906,1.64374130780069));
#73800=CARTESIAN_POINT('Ctrl Pts',(34.2922128993694,-4.06428393345358,3.287340649827));
#73801=CARTESIAN_POINT('Ctrl Pts',(34.2524249929821,-2.68116326291599,4.17547293709044));
#73802=CARTESIAN_POINT('Ctrl Pts',(34.212669668843,-1.29917522752317,5.06287793434716));
#73803=CARTESIAN_POINT('Ctrl Pts',(34.172914344704,0.567120692079285,5.19605267203163));
#73804=CARTESIAN_POINT('Ctrl Pts',(34.1331590205649,2.06111094347969,4.5138711068721));
#73805=CARTESIAN_POINT('Ctrl Pts',(34.0934036964258,3.55510119487992,3.83168954171264));
#73806=CARTESIAN_POINT('Ctrl Pts',(34.0536483722868,4.67678577807796,2.33415167370907));
#73807=CARTESIAN_POINT('Ctrl Pts',(34.0138930481477,4.91132125082459,0.708614325277302));
#73808=CARTESIAN_POINT('Ctrl Pts',(33.9741377240087,5.14585672357124,-0.916923023154561));
#73809=CARTESIAN_POINT('Ctrl Pts',(33.9343823998696,4.49324308586658,-2.67045985201484));
#73810=CARTESIAN_POINT('Ctrl Pts',(33.8946270757306,3.25302430642285,-3.74713804824555));
#73811=CARTESIAN_POINT('Ctrl Pts',(33.8548717515915,2.01280552697904,-4.82381624447632));
#73812=CARTESIAN_POINT('Ctrl Pts',(33.8151164274525,0.184981605796054,-5.22363580807742));
#73813=CARTESIAN_POINT('Ctrl Pts',(33.7753611033134,-1.39149221649886,-4.76308304590743));
#73814=CARTESIAN_POINT('Ctrl Pts',(33.7356057791743,-2.96796603879368,-4.30253028373747));
#73815=CARTESIAN_POINT('Ctrl Pts',(33.6958504550353,-4.29308976220046,-2.98160519579652));
#73816=CARTESIAN_POINT('Ctrl Pts',(33.6560951308962,-4.75864315316813,-1.4066008785701));
#73817=CARTESIAN_POINT('Ctrl Pts',(33.6446596579789,-4.89255787551782,-0.953556673688374));
#73818=CARTESIAN_POINT('Ctrl Pts',(33.6332241850615,-4.95535139724285,-0.479489849529769));
#73819=CARTESIAN_POINT('Ctrl Pts',(33.6217887121441,-4.9513279518383,-0.00438127959876189));
#73820=CARTESIAN_POINT('Ctrl Pts',(33.5164112878558,-4.95294315282494,-0.00455417533769269));
#73821=CARTESIAN_POINT('Ctrl Pts',(33.5265082475584,-4.95673260333198,-0.42370432509382));
#73822=CARTESIAN_POINT('Ctrl Pts',(33.536605207261,-4.90797969150976,-0.84198576343423));
#73823=CARTESIAN_POINT('Ctrl Pts',(33.5467021669636,-4.80326067454432,-1.24575208446876));
#73824=CARTESIAN_POINT('Ctrl Pts',(33.5864574911026,-4.39094463232837,-2.83552380209275));
#73825=CARTESIAN_POINT('Ctrl Pts',(33.6262128152417,-3.11099883895928,-4.20027096987823));
#73826=CARTESIAN_POINT('Ctrl Pts',(33.6659681393807,-1.55090725206635,-4.71358653883326));
#73827=CARTESIAN_POINT('Ctrl Pts',(33.7057234635198,0.00918433482640424,
-5.22690210778824));
#73828=CARTESIAN_POINT('Ctrl Pts',(33.7454787876589,1.84942171524284,-4.88878607791293));
#73829=CARTESIAN_POINT('Ctrl Pts',(33.7852341117979,3.12515197901683,-3.85443075844271));
#73830=CARTESIAN_POINT('Ctrl Pts',(33.824989435937,4.40088224279089,-2.82007543897243));
#73831=CARTESIAN_POINT('Ctrl Pts',(33.864744760076,5.11210538992238,-1.0894808299069));
#73832=CARTESIAN_POINT('Ctrl Pts',(33.9045000842151,4.93237619796575,0.543025234518007));
#73833=CARTESIAN_POINT('Ctrl Pts',(33.9442554083541,4.7526470060091,2.17553129894301));
#73834=CARTESIAN_POINT('Ctrl Pts',(33.9840107324932,3.68196547496439,3.7099488187275));
#73835=CARTESIAN_POINT('Ctrl Pts',(34.0237660566323,2.21176509090388,4.44199353289049));
#73836=CARTESIAN_POINT('Ctrl Pts',(34.0635213807713,0.741564706843371,5.17403824705348));
#73837=CARTESIAN_POINT('Ctrl Pts',(34.1032767049103,-1.12815453023284,5.1037101555949));
#73838=CARTESIAN_POINT('Ctrl Pts',(34.1430320290494,-2.53920779504284,4.26328923921134));
#73839=CARTESIAN_POINT('Ctrl Pts',(34.1827873531884,-3.95026105985269,3.42286832282788));
#73840=CARTESIAN_POINT('Ctrl Pts',(34.2225426773275,-4.90264835239638,1.8123545815197));
#73841=CARTESIAN_POINT('Ctrl Pts',(34.2622980014666,-4.95923221051056,0.170959778364143));
#73842=CARTESIAN_POINT('Ctrl Pts',(34.2636690969297,-4.96118369431365,0.114350782802527));
#73843=CARTESIAN_POINT('Ctrl Pts',(34.2650401923928,-4.96206966815802,0.0577050558803606));
#73844=CARTESIAN_POINT('Ctrl Pts',(34.2664112878558,-4.96190593350399,0.00105408447129014));
#73845=CARTESIAN_POINT('Origin',(10.45,0.,0.));
#73846=CARTESIAN_POINT('',(35.1217887121441,-4.95125214780166,0.00436800828097772));
#73847=CARTESIAN_POINT('',(35.0164112878558,-4.94977286428982,0.00400141439014362));
#73848=CARTESIAN_POINT('',(10.45,-4.954,-6.06690024297599E-16));
#73849=CARTESIAN_POINT('Ctrl Pts',(35.1217887121441,-4.95125214780166,0.00436800828097772));
#73850=CARTESIAN_POINT('Ctrl Pts',(35.1102880747301,-4.95528165247632,0.482202489736174));
#73851=CARTESIAN_POINT('Ctrl Pts',(35.0987874373162,-4.89175694914764,0.958987841215879));
#73852=CARTESIAN_POINT('Ctrl Pts',(35.0872867999022,-4.75633309420263,1.41439251562917));
#73853=CARTESIAN_POINT('Ctrl Pts',(35.0475314757632,-4.28820084590116,2.98863225505063));
#73854=CARTESIAN_POINT('Ctrl Pts',(35.0077761516241,-2.9609155390429,4.30738533457894));
#73855=CARTESIAN_POINT('Ctrl Pts',(34.9680208274851,-1.38368955531006,4.76535559064072));
#73856=CARTESIAN_POINT('Ctrl Pts',(34.928265503346,0.193536428422955,5.22332584670255));
#73857=CARTESIAN_POINT('Ctrl Pts',(34.8885101792069,2.02070308903071,4.82051327929763));
#73858=CARTESIAN_POINT('Ctrl Pts',(34.8487548550679,3.25915686285117,3.74180534421805));
#73859=CARTESIAN_POINT('Ctrl Pts',(34.8089995309288,4.49761063667156,2.66309740913853));
#73860=CARTESIAN_POINT('Ctrl Pts',(34.7692442067898,5.14735152370474,0.908494106384621));
#73861=CARTESIAN_POINT('Ctrl Pts',(34.7294888826507,4.91015412269713,-0.716656948771265));
#73862=CARTESIAN_POINT('Ctrl Pts',(34.6897335585117,4.67295672168951,-2.34180800392724));
#73863=CARTESIAN_POINT('Ctrl Pts',(34.6499782343726,3.54882103264079,-3.83750681148506));
#73864=CARTESIAN_POINT('Ctrl Pts',(34.6102229102336,2.05371553403593,-4.51724066173508));
#73865=CARTESIAN_POINT('Ctrl Pts',(34.5704675860945,0.558610035431147,-5.19697451198506));
#73866=CARTESIAN_POINT('Ctrl Pts',(34.5307122619555,-1.30746527272985,-5.06074340492735));
#73867=CARTESIAN_POINT('Ctrl Pts',(34.4909569378164,-2.68799809677426,-4.17107623072434));
#73868=CARTESIAN_POINT('Ctrl Pts',(34.4512341959257,-4.06739947832071,-3.28213820053907));
#73869=CARTESIAN_POINT('Ctrl Pts',(34.4115114540349,-4.9620539211673,-1.64099858346418));
#73870=CARTESIAN_POINT('Ctrl Pts',(34.3717887121441,-4.96217785588676,2.53259700289598E-5));
#73871=CARTESIAN_POINT('Ctrl Pts',(34.2664112878558,-4.96190593350399,0.00105408447129014));
#73872=CARTESIAN_POINT('Ctrl Pts',(34.3047955165318,-4.95732213276104,-1.58490684956072));
#73873=CARTESIAN_POINT('Ctrl Pts',(34.3431797452078,-4.13004313544497,-3.17497808106077));
#73874=CARTESIAN_POINT('Ctrl Pts',(34.3815639738838,-2.82676794883698,-4.07830777737638));
#73875=CARTESIAN_POINT('Ctrl Pts',(34.4213192980228,-1.4769394053648,-5.01390466495807));
#73876=CARTESIAN_POINT('Ctrl Pts',(34.4610746221618,0.383498105263837,-5.21282257511845));
#73877=CARTESIAN_POINT('Ctrl Pts',(34.5008299463009,1.90061998926887,-4.58375992172047));
#73878=CARTESIAN_POINT('Ctrl Pts',(34.5405852704399,3.41774187327381,-3.95469726832253));
#73879=CARTESIAN_POINT('Ctrl Pts',(34.580340594579,4.59154813065502,-2.49765405136622));
#73880=CARTESIAN_POINT('Ctrl Pts',(34.6200959187181,4.88327192522793,-0.881400401562105));
#73881=CARTESIAN_POINT('Ctrl Pts',(34.6598512428571,5.17499571980086,0.7348532482421));
#73882=CARTESIAN_POINT('Ctrl Pts',(34.6996065669962,4.58463705156541,2.51031733089426));
#73883=CARTESIAN_POINT('Ctrl Pts',(34.7393618911352,3.38316540113682,3.63006931505732));
#73884=CARTESIAN_POINT('Ctrl Pts',(34.7791172152743,2.18169375070823,4.74982129922038));
#73885=CARTESIAN_POINT('Ctrl Pts',(34.8188725394133,0.369109118086691,5.2138611848944));
#73886=CARTESIAN_POINT('Ctrl Pts',(34.8586278635524,-1.22262795667244,4.80919871112959));
#73887=CARTESIAN_POINT('Ctrl Pts',(34.8983831876914,-2.81436503143139,4.40453623736482));
#73888=CARTESIAN_POINT('Ctrl Pts',(34.9381385118305,-4.18525454832788,3.13117140416126));
#73889=CARTESIAN_POINT('Ctrl Pts',(34.9778938359695,-4.70607017366559,1.57356756581696));
#73890=CARTESIAN_POINT('Ctrl Pts',(34.9907329865983,-4.87426978990138,1.07053279667574));
#73891=CARTESIAN_POINT('Ctrl Pts',(35.003572137227,-4.95380717245401,0.537852057524207));
#73892=CARTESIAN_POINT('Ctrl Pts',(35.0164112878558,-4.94977286428982,0.00400141439014362));
#73893=CARTESIAN_POINT('Origin',(10.45,0.,0.));
#73894=CARTESIAN_POINT('',(35.8717887121441,-4.94662056565563,-0.00205432018779872));
#73895=CARTESIAN_POINT('',(35.7664112878558,-4.94744996620173,-0.002834044534147));
#73896=CARTESIAN_POINT('',(10.45,-4.954,-6.06690024297599E-16));
#73897=CARTESIAN_POINT('Ctrl Pts',(35.8717887121441,-4.94662056565563,-0.00205432018779872));
#73898=CARTESIAN_POINT('Ctrl Pts',(35.8488200195645,-4.94305946801648,0.954509582032164));
#73899=CARTESIAN_POINT('Ctrl Pts',(35.8258513269848,-4.67593326216678,1.91291262543561));
#73900=CARTESIAN_POINT('Ctrl Pts',(35.8028826344052,-4.15809531370436,2.70803509441322));
#73901=CARTESIAN_POINT('Ctrl Pts',(35.7631273102661,-3.26179634408548,4.08427152471256));
#73902=CARTESIAN_POINT('Ctrl Pts',(35.7233719861271,-1.6144060892818,4.97134611834161));
#73903=CARTESIAN_POINT('Ctrl Pts',(35.6836166619881,0.0279376812127906,
4.96209937198498));
#73904=CARTESIAN_POINT('Ctrl Pts',(35.643861337849,1.67028145170757,4.95285262562834));
#73905=CARTESIAN_POINT('Ctrl Pts',(35.6041060137099,3.30757873789314,4.0472845392858));
#73906=CARTESIAN_POINT('Ctrl Pts',(35.5643506895709,4.18832436752257,2.66104296796643));
#73907=CARTESIAN_POINT('Ctrl Pts',(35.5245953654318,5.06906999715185,1.2748013966473));
#73908=CARTESIAN_POINT('Ctrl Pts',(35.4848400412928,5.19326397022515,-0.592113659648685));
#73909=CARTESIAN_POINT('Ctrl Pts',(35.4450847171537,4.50390233381199,-2.0828044702768));
#73910=CARTESIAN_POINT('Ctrl Pts',(35.4053293930147,3.81454069739863,-3.57349528090534));
#73911=CARTESIAN_POINT('Ctrl Pts',(35.3655740688756,2.31162345149843,-4.68796184586595));
#73912=CARTESIAN_POINT('Ctrl Pts',(35.3258187447365,0.684976507282884,-4.91467373027875));
#73913=CARTESIAN_POINT('Ctrl Pts',(35.2860634205975,-0.941670436932289,
-5.1413856146915));
#73914=CARTESIAN_POINT('Ctrl Pts',(35.2463080964584,-2.69204707946263,-4.48034281855686));
#73915=CARTESIAN_POINT('Ctrl Pts',(35.2065527723194,-3.76274580585559,-3.2349582208322));
#73916=CARTESIAN_POINT('Ctrl Pts',(35.1782980855943,-4.52370695373544,-2.34984528506821));
#73917=CARTESIAN_POINT('Ctrl Pts',(35.1500433988692,-4.9413524884922,-1.16957245205999));
#73918=CARTESIAN_POINT('Ctrl Pts',(35.1217887121441,-4.95125214780166,0.00436800828097772));
#73919=CARTESIAN_POINT('Ctrl Pts',(35.0164112878558,-4.94977286428982,0.00400141439014362));
#73920=CARTESIAN_POINT('Ctrl Pts',(35.0433274613661,-4.94131528468185,-1.11517048059559));
#73921=CARTESIAN_POINT('Ctrl Pts',(35.0702436348764,-4.56556420838047,-2.23948404641346));
#73922=CARTESIAN_POINT('Ctrl Pts',(35.0971598083867,-3.86942204801114,-3.10657116091815));
#73923=CARTESIAN_POINT('Ctrl Pts',(35.1369151325258,-2.84121656324018,-4.38726320582311));
#73924=CARTESIAN_POINT('Ctrl Pts',(35.1766704566648,-1.11406385991951,-5.10680445214766));
#73925=CARTESIAN_POINT('Ctrl Pts',(35.2164257808039,0.519288032529988,-4.93493174246518));
#73926=CARTESIAN_POINT('Ctrl Pts',(35.2561811049429,2.1526399249793,-4.76305903278271));
#73927=CARTESIAN_POINT('Ctrl Pts',(35.295936429082,3.69219100655747,-3.69977236709346));
#73928=CARTESIAN_POINT('Ctrl Pts',(35.335691753221,4.43130075601119,-2.23311105273416));
#73929=CARTESIAN_POINT('Ctrl Pts',(35.3754470773601,5.17041050546498,-0.76644973837468));
#73930=CARTESIAN_POINT('Ctrl Pts',(35.4152024014992,5.10907892279414,1.10358622465495));
#73931=CARTESIAN_POINT('Ctrl Pts',(35.4549577256382,4.27545666994702,2.51866663657865));
#73932=CARTESIAN_POINT('Ctrl Pts',(35.4947130497773,3.44183441710001,3.93374704850219));
#73933=CARTESIAN_POINT('Ctrl Pts',(35.5344683739163,1.83592149407689,4.8938719093199));
#73934=CARTESIAN_POINT('Ctrl Pts',(35.5742236980554,0.194817927850411,4.95835228058715));
#73935=CARTESIAN_POINT('Ctrl Pts',(35.6139790221944,-1.44628563837616,5.0228326518544));
#73936=CARTESIAN_POINT('Ctrl Pts',(35.6537343463335,-3.12257984780612,4.19166853357104));
#73937=CARTESIAN_POINT('Ctrl Pts',(35.6934896704725,-4.0646602749189,2.84635700786281));
#73938=CARTESIAN_POINT('Ctrl Pts',(35.717796876267,-4.64066722021841,2.02380644838001));
#73939=CARTESIAN_POINT('Ctrl Pts',(35.7421040820614,-4.94219966027112,1.00904980577044));
#73940=CARTESIAN_POINT('Ctrl Pts',(35.7664112878558,-4.94744996620173,-0.002834044534147));
#73941=CARTESIAN_POINT('Origin',(10.45,0.,0.));
#73942=CARTESIAN_POINT('',(36.6217887121441,-4.95879821043464,-0.00354683266310052));
#73943=CARTESIAN_POINT('',(36.5164112878558,-4.960151313927,-0.00283453072728394));
#73944=CARTESIAN_POINT('',(10.45,-4.954,-6.06690024297599E-16));
#73945=CARTESIAN_POINT('Ctrl Pts',(36.6217887121441,-4.95879821043464,-0.00354683266310052));
#73946=CARTESIAN_POINT('Ctrl Pts',(36.5873519643988,-4.94727189684655,1.42166512058158));
#73947=CARTESIAN_POINT('Ctrl Pts',(36.5529152166535,-4.30004065620608,2.85600973832634));
#73948=CARTESIAN_POINT('Ctrl Pts',(36.5184784689082,-3.21681736593896,3.77826645686206));
#73949=CARTESIAN_POINT('Ctrl Pts',(36.4787231447691,-1.96629587831048,4.8429609238304));
#73950=CARTESIAN_POINT('Ctrl Pts',(36.4389678206301,-0.134709133881325,
5.22517393978799));
#73951=CARTESIAN_POINT('Ctrl Pts',(36.399212496491,1.43726013425452,4.74947304431184));
#73952=CARTESIAN_POINT('Ctrl Pts',(36.359457172352,3.00922940239028,4.27377214883571));
#73953=CARTESIAN_POINT('Ctrl Pts',(36.3197018482129,4.32158119423285,2.94015734192591));
#73954=CARTESIAN_POINT('Ctrl Pts',(36.2799465240739,4.77195768647691,1.36074620048107));
#73955=CARTESIAN_POINT('Ctrl Pts',(36.2401911999348,5.222334178721,-0.218664940963859));
#73956=CARTESIAN_POINT('Ctrl Pts',(36.2004358757957,4.81073537136662,-2.04387241694371));
#73957=CARTESIAN_POINT('Ctrl Pts',(36.1606805516567,3.72608141976468,-3.27712191766261));
#73958=CARTESIAN_POINT('Ctrl Pts',(36.1209252275176,2.6414274681628,-4.51037141838145));
#73959=CARTESIAN_POINT('Ctrl Pts',(36.0811699033786,0.883718372313122,-5.15166294383926));
#73960=CARTESIAN_POINT('Ctrl Pts',(36.0414145792395,-0.740272663720714,
-4.90664927332293));
#73961=CARTESIAN_POINT('Ctrl Pts',(36.0016592551005,-2.36426369975464,-4.66163560280659));
#73962=CARTESIAN_POINT('Ctrl Pts',(35.9619039309614,-3.85453667597279,-3.53031673631638));
#73963=CARTESIAN_POINT('Ctrl Pts',(35.9221486068224,-4.52706932186502,-2.03195816958627));
#73964=CARTESIAN_POINT('Ctrl Pts',(35.905361975263,-4.81104531709985,-1.39927830221521));
#73965=CARTESIAN_POINT('Ctrl Pts',(35.8885753437035,-4.94922318806473,-0.701157490031947));
#73966=CARTESIAN_POINT('Ctrl Pts',(35.8717887121441,-4.94662056565563,-0.00205432018779872));
#73967=CARTESIAN_POINT('Ctrl Pts',(35.7664112878558,-4.94744996620173,-0.002834044534147));
#73968=CARTESIAN_POINT('Ctrl Pts',(35.7818594062004,-4.95078672765623,-0.64592324214638));
#73969=CARTESIAN_POINT('Ctrl Pts',(35.7973075245451,-4.83445313833523,-1.28785209958534));
#73970=CARTESIAN_POINT('Ctrl Pts',(35.8127556428897,-4.59285123428814,-1.87854435599614));
#73971=CARTESIAN_POINT('Ctrl Pts',(35.8525109670288,-3.97109512174899,-3.39867526101325));
#73972=CARTESIAN_POINT('Ctrl Pts',(35.8922662911678,-2.51971625187527,-4.57947813791414));
#73973=CARTESIAN_POINT('Ctrl Pts',(35.9320216153069,-0.904884865128097,
-4.8789747637326));
#73974=CARTESIAN_POINT('Ctrl Pts',(35.9717769394459,0.709946521618895,-5.17847138955102));
#73975=CARTESIAN_POINT('Ctrl Pts',(36.011532263585,2.4882304252392,-4.59666176428724));
#73976=CARTESIAN_POINT('Ctrl Pts',(36.051287587724,3.61375003293099,-3.40059143130933));
#73977=CARTESIAN_POINT('Ctrl Pts',(36.0910429118631,4.73926964062285,-2.20452109833136));
#73978=CARTESIAN_POINT('Ctrl Pts',(36.1307982360022,5.21202495238608,-0.39419005763898));
#73979=CARTESIAN_POINT('Ctrl Pts',(36.1705535601412,4.81502541832947,1.19947552771663));
#73980=CARTESIAN_POINT('Ctrl Pts',(36.2103088842803,4.41802588427284,2.79314111307233));
#73981=CARTESIAN_POINT('Ctrl Pts',(36.2500642084193,3.15127150439663,4.17014124309119));
#73982=CARTESIAN_POINT('Ctrl Pts',(36.2898195325584,1.59619146287508,4.69844486981268));
#73983=CARTESIAN_POINT('Ctrl Pts',(36.3295748566974,0.0411114213536087,
5.22674849653414));
#73984=CARTESIAN_POINT('Ctrl Pts',(36.3693301808365,-1.80229428181327,4.90635561995797));
#73985=CARTESIAN_POINT('Ctrl Pts',(36.4090855049756,-3.08791844754446,3.88432376920091));
#73986=CARTESIAN_POINT('Ctrl Pts',(36.4448607659356,-4.24483367894236,2.96461158065307));
#73987=CARTESIAN_POINT('Ctrl Pts',(36.4806360268957,-4.95006028065536,1.4767157475938));
#73988=CARTESIAN_POINT('Ctrl Pts',(36.5164112878558,-4.960151313927,-0.00283453072728394));
#73989=CARTESIAN_POINT('Origin',(10.45,0.,0.));
#73990=CARTESIAN_POINT('',(37.3717887121441,-4.95785187747778,0.00390184669589733));
#73991=CARTESIAN_POINT('',(37.2664112878558,-4.95623082790828,0.00431859730377795));
#73992=CARTESIAN_POINT('',(10.45,-4.954,-6.06690024297599E-16));
#73993=CARTESIAN_POINT('Ctrl Pts',(37.3717887121441,-4.95785187747778,0.00390184669589733));
#73994=CARTESIAN_POINT('Ctrl Pts',(37.3656392333722,-4.96004850919265,0.258532516263073));
#73995=CARTESIAN_POINT('Ctrl Pts',(37.3594897546003,-4.94212966831781,0.512852861899553));
#73996=CARTESIAN_POINT('Ctrl Pts',(37.3533402758283,-4.90302063743832,0.763871725959299));
#73997=CARTESIAN_POINT('Ctrl Pts',(37.3135849516893,-4.65018746945052,2.38666557172065));
#73998=CARTESIAN_POINT('Ctrl Pts',(37.2738296275502,-3.51173140695091,3.87147728190302));
#73999=CARTESIAN_POINT('Ctrl Pts',(37.2340743034112,-2.01015914239786,4.5367929335275));
#74000=CARTESIAN_POINT('Ctrl Pts',(37.1943189792721,-0.508586877844729,
5.20210858515201));
#74001=CARTESIAN_POINT('Ctrl Pts',(37.1545636551331,1.3561015887619,5.04792817821849));
#74002=CARTESIAN_POINT('Ctrl Pts',(37.114808330994,2.72801223498102,4.14501827783009));
#74003=CARTESIAN_POINT('Ctrl Pts',(37.075053006855,4.09992288120007,3.24210837744174));
#74004=CARTESIAN_POINT('Ctrl Pts',(37.0352976827159,4.97905570703167,1.59046898359859));
#74005=CARTESIAN_POINT('Ctrl Pts',(36.9955423585768,4.9619060349538,-0.0518113523523847));
#74006=CARTESIAN_POINT('Ctrl Pts',(36.9557870344378,4.94475636287593,-1.69409168830335));
#74007=CARTESIAN_POINT('Ctrl Pts',(36.9160317102987,4.0313241928886,-3.32701296636214));
#74008=CARTESIAN_POINT('Ctrl Pts',(36.8762763861597,2.6408618587565,-4.2010788082045));
#74009=CARTESIAN_POINT('Ctrl Pts',(36.8365210620206,1.25039952462425,-5.07514465004697));
#74010=CARTESIAN_POINT('Ctrl Pts',(36.7967657378816,-0.617092973652882,
-5.19035505567283));
#74011=CARTESIAN_POINT('Ctrl Pts',(36.7570104137425,-2.10445019667369,-4.49382932261318));
#74012=CARTESIAN_POINT('Ctrl Pts',(36.7172550896035,-3.59180741969424,-3.79730358955364));
#74013=CARTESIAN_POINT('Ctrl Pts',(36.6774997654644,-4.69902936745862,-2.28904171780891));
#74014=CARTESIAN_POINT('Ctrl Pts',(36.6377444413253,-4.91791222592692,-0.661322822947106));
#74015=CARTESIAN_POINT('Ctrl Pts',(36.6324258649316,-4.94719497557761,-0.443562121019674));
#74016=CARTESIAN_POINT('Ctrl Pts',(36.6271072885378,-4.96057838955638,-0.223663398451484));
#74017=CARTESIAN_POINT('Ctrl Pts',(36.6217887121441,-4.95879821043464,-0.00354683266310052));
#74018=CARTESIAN_POINT('Ctrl Pts',(36.5164112878558,-4.960151313927,-0.00283453072728394));
#74019=CARTESIAN_POINT('Ctrl Pts',(36.5203913510348,-4.96127395982487,-0.167437203807423));
#74020=CARTESIAN_POINT('Ctrl Pts',(36.5243714142137,-4.95379293417925,-0.331936584213332));
#74021=CARTESIAN_POINT('Ctrl Pts',(36.5283514773927,-4.93737302018323,-0.495538814038059));
#74022=CARTESIAN_POINT('Ctrl Pts',(36.5681068015317,-4.77336079879503,-2.12969872158212));
#74023=CARTESIAN_POINT('Ctrl Pts',(36.6078621256708,-3.71749372772285,-3.67434771173236));
#74024=CARTESIAN_POINT('Ctrl Pts',(36.6476174498099,-2.2544053816326,-4.42050539418716));
#74025=CARTESIAN_POINT('Ctrl Pts',(36.6873727739489,-0.791317035542348,
-5.16666307664196));
#74026=CARTESIAN_POINT('Ctrl Pts',(36.727128098088,1.07899258556597,-5.11432945140131));
#74027=CARTESIAN_POINT('Ctrl Pts',(36.766883422227,2.4980672888367,-4.28752514602669));
#74028=CARTESIAN_POINT('Ctrl Pts',(36.8066387463661,3.91714199210752,-3.46072084065203));
#74029=CARTESIAN_POINT('Ctrl Pts',(36.8463940705051,4.8849817775407,-1.8594458551433));
#74030=CARTESIAN_POINT('Ctrl Pts',(36.8861493946442,4.95735735749111,-0.218671539309196));
#74031=CARTESIAN_POINT('Ctrl Pts',(36.9259047187833,5.02973293744153,1.42210277652491));
#74032=CARTESIAN_POINT('Ctrl Pts',(36.9656600429223,4.20664431190917,3.1023764226844));
#74033=CARTESIAN_POINT('Ctrl Pts',(37.0054153670614,2.86588058829837,4.05091862867918));
#74034=CARTESIAN_POINT('Ctrl Pts',(37.0451706912004,1.52511686468772,4.99946083467385));
#74035=CARTESIAN_POINT('Ctrl Pts',(37.0849260153394,-0.333321957001219,
5.216271600504));
#74036=CARTESIAN_POINT('Ctrl Pts',(37.1246813394785,-1.85642601585715,4.601836332316));
#74037=CARTESIAN_POINT('Ctrl Pts',(37.1644366636176,-3.37953007471326,3.98740106412792));
#74038=CARTESIAN_POINT('Ctrl Pts',(37.2041919877566,-4.56729937073627,2.54171976192149));
#74039=CARTESIAN_POINT('Ctrl Pts',(37.2439473118957,-4.87456318408798,0.928348188082862));
#74040=CARTESIAN_POINT('Ctrl Pts',(37.2514353038824,-4.9324369160222,0.62446654007456));
#74041=CARTESIAN_POINT('Ctrl Pts',(37.2589232958691,-4.95907343999133,0.314635836675023));
#74042=CARTESIAN_POINT('Ctrl Pts',(37.2664112878558,-4.95623082790828,0.00431859730377795));
#74043=CARTESIAN_POINT('Origin',(10.45,0.,0.));
#74044=CARTESIAN_POINT('',(38.1217887121441,-4.94678507297176,0.00149831882859774));
#74045=CARTESIAN_POINT('',(38.0164112878558,-4.94597286168509,0.000644103793583921));
#74046=CARTESIAN_POINT('',(10.45,-4.954,-6.06690024297599E-16));
#74047=CARTESIAN_POINT('Ctrl Pts',(38.1217887121441,-4.94678507297176,0.00149831882859774));
#74048=CARTESIAN_POINT('Ctrl Pts',(38.1041711782065,-4.94843324508386,0.735362320538199));
#74049=CARTESIAN_POINT('Ctrl Pts',(38.0865536442689,-4.79519616293353,1.46843094882367));
#74050=CARTESIAN_POINT('Ctrl Pts',(38.0689361103313,-4.48317629555338,2.12606890820242));
#74051=CARTESIAN_POINT('Ctrl Pts',(38.0291807861923,-3.77907939927567,3.6100796859804));
#74052=CARTESIAN_POINT('Ctrl Pts',(37.9894254620532,-2.26643827773527,4.70998691207959));
#74053=CARTESIAN_POINT('Ctrl Pts',(37.9496701379142,-0.637905686603803,
4.92102505154708));
#74054=CARTESIAN_POINT('Ctrl Pts',(37.9099148137751,0.990626904527571,5.13206319101456));
#74055=CARTESIAN_POINT('Ctrl Pts',(37.8701594896361,2.73505096525,4.45423224385044));
#74056=CARTESIAN_POINT('Ctrl Pts',(37.830404165497,3.79383240100999,3.19860832268579));
#74057=CARTESIAN_POINT('Ctrl Pts',(37.7906488413579,4.85261383676997,1.94298440152115));
#74058=CARTESIAN_POINT('Ctrl Pts',(37.7508935172189,5.2257526475675,0.109567506355982));
#74059=CARTESIAN_POINT('Ctrl Pts',(37.7111381930798,4.74243313727792,-1.46009779252003));
#74060=CARTESIAN_POINT('Ctrl Pts',(37.6713828689408,4.25911362698833,-3.02976309139605));
#74061=CARTESIAN_POINT('Ctrl Pts',(37.6316275448017,2.91933579561142,-4.33567679398308));
#74062=CARTESIAN_POINT('Ctrl Pts',(37.5918722206627,1.33780816048755,-4.77844757626196));
#74063=CARTESIAN_POINT('Ctrl Pts',(37.5521168965236,-0.243719474636306,
-5.22121835854084));
#74064=CARTESIAN_POINT('Ctrl Pts',(37.5123615723846,-2.06699691350693,-4.80084622051189));
#74065=CARTESIAN_POINT('Ctrl Pts',(37.4726062482455,-3.29503049620446,-3.71027216082727));
#74066=CARTESIAN_POINT('Ctrl Pts',(37.4390004028784,-4.33310797587571,-2.78839153213513));
#74067=CARTESIAN_POINT('Ctrl Pts',(37.4053945575112,-4.94584766240908,-1.3876110318066));
#74068=CARTESIAN_POINT('Ctrl Pts',(37.3717887121441,-4.95785187747778,0.00390184669589733));
#74069=CARTESIAN_POINT('Ctrl Pts',(37.2664112878558,-4.95623082790828,0.00431859730377795));
#74070=CARTESIAN_POINT('Ctrl Pts',(37.2986786200082,-4.94398141465747,-1.33290364507722));
#74071=CARTESIAN_POINT('Ctrl Pts',(37.3309459521605,-4.38432527605305,-2.67916051664711));
#74072=CARTESIAN_POINT('Ctrl Pts',(37.3632132843128,-3.41794155109712,-3.59734673003167));
#74073=CARTESIAN_POINT('Ctrl Pts',(37.4029686084519,-2.22729777407411,-4.72860822883691));
#74074=CARTESIAN_POINT('Ctrl Pts',(37.4427239325909,-0.419251889347554,
-5.2100693809767));
#74075=CARTESIAN_POINT('Ctrl Pts',(37.48247925673,1.17630066541565,-4.82074136594268));
#74076=CARTESIAN_POINT('Ctrl Pts',(37.5222345808691,2.77185322017895,-4.43141335090864));
#74077=CARTESIAN_POINT('Ctrl Pts',(37.5619899050081,4.15491244497898,-3.17129616870065));
#74078=CARTESIAN_POINT('Ctrl Pts',(37.6017452291472,4.69070067672837,-1.61877708111193));
#74079=CARTESIAN_POINT('Ctrl Pts',(37.6415005532862,5.22648890847773,-0.066257993523289));
#74080=CARTESIAN_POINT('Ctrl Pts',(37.6812558774253,4.91500614717662,1.77866299944616));
#74081=CARTESIAN_POINT('Ctrl Pts',(37.7210112015643,3.89915481177568,3.06919172853735));
#74082=CARTESIAN_POINT('Ctrl Pts',(37.7607665257034,2.88330347637469,4.35972045762861));
#74083=CARTESIAN_POINT('Ctrl Pts',(37.8005218498425,1.16308356687407,5.0958569228415));
#74084=CARTESIAN_POINT('Ctrl Pts',(37.8402771739815,-0.471814661666735,
4.93970480306567));
#74085=CARTESIAN_POINT('Ctrl Pts',(37.8800324981206,-2.10671289020754,4.78355268328984));
#74086=CARTESIAN_POINT('Ctrl Pts',(37.9197878222596,-3.65628943778838,3.73511197852511));
#74087=CARTESIAN_POINT('Ctrl Pts',(37.9595431463987,-4.40953831280109,2.27563841322242));
#74088=CARTESIAN_POINT('Ctrl Pts',(37.9784991935511,-4.76870080239037,1.57973540348341));
#74089=CARTESIAN_POINT('Ctrl Pts',(37.9974552407034,-4.94681402495116,0.790381920166041));
#74090=CARTESIAN_POINT('Ctrl Pts',(38.0164112878558,-4.94597286168509,0.000644103793583921));
#74091=CARTESIAN_POINT('Origin',(-19.0048063345371,0.,0.));
#74092=CARTESIAN_POINT('',(38.3701936654629,-4.51716168224788,0.0013681913210258));
#74093=CARTESIAN_POINT('',(38.5180063345368,-4.52176644287018,-0.00146738152635217));
#74094=CARTESIAN_POINT('',(-19.0048063345371,-4.52375,5.14627461305311E-12));
#74095=CARTESIAN_POINT('',(38.546,-0.439158351705441,-4.50835702469513));
#74096=CARTESIAN_POINT('Ctrl Pts',(38.3701936654629,-4.51716168224788,0.00136819132102561));
#74097=CARTESIAN_POINT('Ctrl Pts',(38.3923314556644,-4.5152704959798,-0.84070012943849));
#74098=CARTESIAN_POINT('Ctrl Pts',(38.4509335671768,-3.91909753352112,-3.072819358561));
#74099=CARTESIAN_POINT('Ctrl Pts',(38.5095356786891,-1.80749920607627,-4.36540260482715));
#74100=CARTESIAN_POINT('Ctrl Pts',(38.546,-0.439158351705441,-4.50835702469513));
#74101=CARTESIAN_POINT('',(38.546,-4.39991769847472,-1.05120802372743));
#74102=CARTESIAN_POINT('Origin',(38.546,0.,0.));
#74103=CARTESIAN_POINT('Ctrl Pts',(38.5180063345368,-4.52176644287018,-0.00146738152635186));
#74104=CARTESIAN_POINT('Ctrl Pts',(38.5273375563579,-4.52240870358347,-0.354396659090419));
#74105=CARTESIAN_POINT('Ctrl Pts',(38.5366687781789,-4.48209384756912,-0.707252988537638));
#74106=CARTESIAN_POINT('Ctrl Pts',(38.546,-4.39991769847472,-1.05120802372743));
#74107=CARTESIAN_POINT('Origin',(-19.0048063345371,0.,0.));
#74108=CARTESIAN_POINT('',(37.6201936654629,-4.52726734572873,0.00356297517063345));
#74109=CARTESIAN_POINT('',(37.7680063345368,-4.5164200107081,0.000588164021544935));
#74110=CARTESIAN_POINT('',(-19.0048063345371,-4.52375,5.14627461305311E-12));
#74111=CARTESIAN_POINT('Ctrl Pts',(37.6201936654629,-4.52726734572873,0.0035629751706337));
#74112=CARTESIAN_POINT('Ctrl Pts',(37.6537995108301,-4.51630568486565,-1.267098386179));
#74113=CARTESIAN_POINT('Ctrl Pts',(37.7271606803363,-3.29487162736131,-4.05941141533821));
#74114=CARTESIAN_POINT('Ctrl Pts',(37.8402771739814,1.44237491738078,-5.15162394203852));
#74115=CARTESIAN_POINT('Ctrl Pts',(37.9595431463987,5.11263327306786,-1.57413477445065));
#74116=CARTESIAN_POINT('Ctrl Pts',(38.0788091188158,4.09043705061455,3.44842457930616));
#74117=CARTESIAN_POINT('Ctrl Pts',(38.198075091233,-0.688330618759455,5.30531057884261));
#74118=CARTESIAN_POINT('Ctrl Pts',(38.2952032734487,-4.0629784562643,2.8514571901215));
#74119=CARTESIAN_POINT('Ctrl Pts',(38.3525761315253,-4.51866671224215,0.671496830346738));
#74120=CARTESIAN_POINT('Ctrl Pts',(38.3701936654629,-4.51716168224788,0.00136819132102561));
#74121=CARTESIAN_POINT('Ctrl Pts',(37.7680063345368,-4.5164200107081,0.000588164021545212));
#74122=CARTESIAN_POINT('Ctrl Pts',(37.7888056115235,-4.51557721299165,-0.790684179628111));
#74123=CARTESIAN_POINT('Ctrl Pts',(37.8493602126493,-3.94034756933214,-3.09560886266219));
#74124=CARTESIAN_POINT('Ctrl Pts',(37.9496701379142,-0.260588162173769,
-5.34342727819689));
#74125=CARTESIAN_POINT('Ctrl Pts',(38.0689361103313,4.35070685430609,-3.11045822607375));
#74126=CARTESIAN_POINT('Ctrl Pts',(38.1882020827485,4.97397191480465,1.9771100447851));
#74127=CARTESIAN_POINT('Ctrl Pts',(38.3074680551657,1.01988032406546,5.25111166397229));
#74128=CARTESIAN_POINT('Ctrl Pts',(38.4068563655133,-3.03575591970712,3.96049046164289));
#74129=CARTESIAN_POINT('Ctrl Pts',(38.4770357919704,-4.36801631736721,1.54840600921283));
#74130=CARTESIAN_POINT('Ctrl Pts',(38.5074598942884,-4.52104053962122,0.397424383040628));
#74131=CARTESIAN_POINT('Ctrl Pts',(38.5180063345368,-4.52176644287018,-0.00146738152635186));
#74132=CARTESIAN_POINT('Origin',(-19.0048063345371,0.,0.));
#74133=CARTESIAN_POINT('',(36.8701936654629,-4.5281314906043,-0.00323879375352202));
#74134=CARTESIAN_POINT('',(37.0180063345368,-4.525787082711,0.00394353140479434));
#74135=CARTESIAN_POINT('',(-19.0048063345371,-4.52375,5.14627461305311E-12));
#74136=CARTESIAN_POINT('Ctrl Pts',(36.8701936654629,-4.5281314906043,-0.00323879375352231));
#74137=CARTESIAN_POINT('Ctrl Pts',(36.8755122418567,-4.52975706293013,-0.204238453520589));
#74138=CARTESIAN_POINT('Ctrl Pts',(36.9205861423895,-4.4261858061835,-1.90598563772707));
#74139=CARTESIAN_POINT('Ctrl Pts',(37.0054153670614,-2.26880168119574,-4.84478234871799));
#74140=CARTESIAN_POINT('Ctrl Pts',(37.1246813394785,2.84710618461792,-4.5291688611629));
#74141=CARTESIAN_POINT('Ctrl Pts',(37.2439473118957,5.34941065311671,-0.0558578206189876));
#74142=CARTESIAN_POINT('Ctrl Pts',(37.3632132843128,2.9410676247427,4.46873061775304));
#74143=CARTESIAN_POINT('Ctrl Pts',(37.48247925673,-2.16715872819103,4.89110059102707));
#74144=CARTESIAN_POINT('Ctrl Pts',(37.56813938378,-4.40712914903362,1.96965775200708));
#74145=CARTESIAN_POINT('Ctrl Pts',(37.614044186691,-4.5292732021518,0.236079222940852));
#74146=CARTESIAN_POINT('Ctrl Pts',(37.6201936654629,-4.52726734572873,0.0035629751706337));
#74147=CARTESIAN_POINT('Ctrl Pts',(37.0180063345368,-4.525787082711,0.0039435314047942));
#74148=CARTESIAN_POINT('Ctrl Pts',(37.0502736666892,-4.51460151888657,-1.21714228187317));
#74149=CARTESIAN_POINT('Ctrl Pts',(37.1222963229807,-3.37390546114829,-3.96109486306854));
#74150=CARTESIAN_POINT('Ctrl Pts',(37.2340743034112,1.26817861053563,-5.1972267358067));
#74151=CARTESIAN_POINT('Ctrl Pts',(37.3533402758283,5.05700430786462,-1.745194981863));
#74152=CARTESIAN_POINT('Ctrl Pts',(37.4726062482455,4.20371193315622,3.30887930675979));
#74153=CARTESIAN_POINT('Ctrl Pts',(37.5918722206627,-0.508749602332581,
5.32549053072501));
#74154=CARTESIAN_POINT('Ctrl Pts',(37.6903389160931,-4.01344027747341,2.95422312405012));
#74155=CARTESIAN_POINT('Ctrl Pts',(37.7490502873845,-4.51718811977569,0.721738032169875));
#74156=CARTESIAN_POINT('Ctrl Pts',(37.7680063345368,-4.5164200107081,0.000588164021545212));
#74157=CARTESIAN_POINT('Origin',(-19.0048063345371,0.,0.));
#74158=CARTESIAN_POINT('',(36.1201936654629,-4.51701146222944,-0.00187590450993699));
#74159=CARTESIAN_POINT('',(36.2680063345368,-4.52936707839667,-0.0025883545316796));
#74160=CARTESIAN_POINT('',(-19.0048063345371,-4.52375,5.14627461305311E-12));
#74161=CARTESIAN_POINT('Ctrl Pts',(36.1201936654629,-4.51701146222944,-0.0018759045099373));
#74162=CARTESIAN_POINT('Ctrl Pts',(36.1369802970224,-4.51938804945676,-0.64026265553622));
#74163=CARTESIAN_POINT('Ctrl Pts',(36.1935222527209,-4.09438860903943,-2.78750195261098));
#74164=CARTESIAN_POINT('Ctrl Pts',(36.2898195325583,-0.79808549366158,-5.28984210344808));
#74165=CARTESIAN_POINT('Ctrl Pts',(36.4090855049755,4.01707590461207,-3.53305413112963));
#74166=CARTESIAN_POINT('Ctrl Pts',(36.5283514773927,5.14463147875642,1.46701590488028));
#74167=CARTESIAN_POINT('Ctrl Pts',(36.6476174498098,1.54950546845328,5.12039094490375));
#74168=CARTESIAN_POINT('Ctrl Pts',(36.7615648458333,-3.24428659251404,4.12002897620758));
#74169=CARTESIAN_POINT('Ctrl Pts',(36.8357569177176,-4.51760622595037,1.29819491102844));
#74170=CARTESIAN_POINT('Ctrl Pts',(36.8701936654629,-4.5281314906043,-0.00323879375352231));
#74171=CARTESIAN_POINT('Ctrl Pts',(36.2680063345368,-4.52936707839667,-0.00258835453167952));
#74172=CARTESIAN_POINT('Ctrl Pts',(36.2719863977159,-4.53039222360893,-0.152895448264976));
#74173=CARTESIAN_POINT('Ctrl Pts',(36.3157217850339,-4.45532562316811,-1.80352596964413));
#74174=CARTESIAN_POINT('Ctrl Pts',(36.399212496491,-2.4304670141352,-4.76573200043202));
#74175=CARTESIAN_POINT('Ctrl Pts',(36.5184784689082,2.69315822717824,-4.62236649547752));
#74176=CARTESIAN_POINT('Ctrl Pts',(36.6377444413254,5.34450979925368,-0.235748984964162));
#74177=CARTESIAN_POINT('Ctrl Pts',(36.7570104137425,3.08969722168957,4.36728164088206));
#74178=CARTESIAN_POINT('Ctrl Pts',(36.8762763861597,-2.00140852293053,4.96122453667856));
#74179=CARTESIAN_POINT('Ctrl Pts',(36.9632750264245,-4.3749228334945,2.07232576585655));
#74180=CARTESIAN_POINT('Ctrl Pts',(37.0105183425502,-4.52838281674591,0.28731002546971));
#74181=CARTESIAN_POINT('Ctrl Pts',(37.0180063345368,-4.525787082711,0.0039435314047942));
#74182=CARTESIAN_POINT('Origin',(-19.0048063345371,0.,0.));
#74183=CARTESIAN_POINT('',(35.3701936654629,-4.52124079604718,0.00398865108261888));
#74184=CARTESIAN_POINT('',(35.5180063345368,-4.51776883015844,-0.00258791056364449));
#74185=CARTESIAN_POINT('',(-19.0048063345371,-4.52375,5.14627461305311E-12));
#74186=CARTESIAN_POINT('Ctrl Pts',(35.3701936654629,-4.52124079604718,0.0039886510826187));
#74187=CARTESIAN_POINT('Ctrl Pts',(35.398448352188,-4.5122009123571,-1.06799624142191));
#74188=CARTESIAN_POINT('Ctrl Pts',(35.4664583630522,-3.59422183212154,-3.66221952290216));
#74189=CARTESIAN_POINT('Ctrl Pts',(35.5742236980554,0.738470871532858,-5.29849324252636));
#74190=CARTESIAN_POINT('Ctrl Pts',(35.6934896704726,4.85564198041892,-2.24546450419021));
#74191=CARTESIAN_POINT('Ctrl Pts',(35.8127556428897,4.5154184323632,2.86886148647546));
#74192=CARTESIAN_POINT('Ctrl Pts',(35.9320216153069,0.0301195233717248,
5.34962266769844));
#74193=CARTESIAN_POINT('Ctrl Pts',(36.0345009561646,-3.84763319583539,3.2615588907316));
#74194=CARTESIAN_POINT('Ctrl Pts',(36.0972249728833,-4.51375964239769,0.87161136893887));
#74195=CARTESIAN_POINT('Ctrl Pts',(36.1201936654629,-4.51701146222944,-0.0018759045099373));
#74196=CARTESIAN_POINT('Ctrl Pts',(35.5180063345368,-4.51776883015844,-0.00258791056364442));
#74197=CARTESIAN_POINT('Ctrl Pts',(35.5334544528815,-4.52081579718175,-0.589825447444406));
#74198=CARTESIAN_POINT('Ctrl Pts',(35.5886578953653,-4.14120522846699,-2.68451692967342));
#74199=CARTESIAN_POINT('Ctrl Pts',(35.6836166619881,-0.975553337067666,
-5.26000630617043));
#74200=CARTESIAN_POINT('Ctrl Pts',(35.8028826344052,3.89597177940602,-3.66616620183877));
#74201=CARTESIAN_POINT('Ctrl Pts',(35.9221486068224,5.19106272102259,1.29315053937908));
#74202=CARTESIAN_POINT('Ctrl Pts',(36.0414145792395,1.72084867623149,5.06537763153141));
#74203=CARTESIAN_POINT('Ctrl Pts',(36.1567004884777,-3.16055193286242,4.21696646507988));
#74204=CARTESIAN_POINT('Ctrl Pts',(36.2322310735768,-4.52015244138191,1.34846444553836));
#74205=CARTESIAN_POINT('Ctrl Pts',(36.2680063345368,-4.52936707839667,-0.00258835453167952));
#74206=CARTESIAN_POINT('Origin',(-19.0048063345371,0.,0.));
#74207=CARTESIAN_POINT('',(34.620193665463,-4.53121761719171,2.31264352865476E-5));
#74208=CARTESIAN_POINT('',(34.7680063345368,-4.51988998684523,0.00365389551349821));
#74209=CARTESIAN_POINT('',(-19.0048063345371,-4.52375,5.14627461305311E-12));
#74210=CARTESIAN_POINT('Ctrl Pts',(34.620193665463,-4.53121761719171,2.31264352862156E-5));
#74211=CARTESIAN_POINT('Ctrl Pts',(34.6599164073537,-4.53110444608029,-1.49847947960086));
#74212=CARTESIAN_POINT('Ctrl Pts',(34.7393944733835,-2.89652516710536,-4.49692522971762));
#74213=CARTESIAN_POINT('Ctrl Pts',(34.8586278635524,2.21410381975605,-4.8700219861014));
#74214=CARTESIAN_POINT('Ctrl Pts',(34.9778938359695,5.29362066876786,-0.772625449552068));
#74215=CARTESIAN_POINT('Ctrl Pts',(35.0971598083868,3.51368606780953,4.03402777461097));
#74216=CARTESIAN_POINT('Ctrl Pts',(35.2164257808038,-1.49175106234197,5.13751385765428));
#74217=CARTESIAN_POINT('Ctrl Pts',(35.307437066496,-4.26639226681861,2.38070896116213));
#74218=CARTESIAN_POINT('Ctrl Pts',(35.358693028049,-4.52492034222639,0.440323680449301));
#74219=CARTESIAN_POINT('Ctrl Pts',(35.3701936654629,-4.52124079604718,0.0039886510826187));
#74220=CARTESIAN_POINT('Ctrl Pts',(34.7680063345368,-4.51988998684523,0.00365389551349841));
#74221=CARTESIAN_POINT('Ctrl Pts',(34.7949225080472,-4.51216693966198,-1.01831902736694));
#74222=CARTESIAN_POINT('Ctrl Pts',(34.8615940056966,-3.66226324200522,-3.56138095634942));
#74223=CARTESIAN_POINT('Ctrl Pts',(34.968020827485,0.559842683756944,-5.32033333739675));
#74224=CARTESIAN_POINT('Ctrl Pts',(35.0872867999022,4.7773704624956,-2.40750952598498));
#74225=CARTESIAN_POINT('Ctrl Pts',(35.2065527723194,4.60935547635934,2.71536604189249));
#74226=CARTESIAN_POINT('Ctrl Pts',(35.3258187447365,0.210032554159402,5.34558294083782));
#74227=CARTESIAN_POINT('Ctrl Pts',(35.429636598809,-3.78729362285914,3.36357162759583));
#74228=CARTESIAN_POINT('Ctrl Pts',(35.4936991287425,-4.5129745081037,0.921414828194142));
#74229=CARTESIAN_POINT('Ctrl Pts',(35.5180063345368,-4.51776883015844,-0.00258791056364442));
#74230=CARTESIAN_POINT('Origin',(-19.0048063345371,0.,0.));
#74231=CARTESIAN_POINT('',(33.8701936654629,-4.52131001657821,-0.00400076979791308));
#74232=CARTESIAN_POINT('',(34.0180063345368,-4.53096931099894,0.000962538283377275));
#74233=CARTESIAN_POINT('',(-19.0048063345371,-4.52375,5.14627461305311E-12));
#74234=CARTESIAN_POINT('Ctrl Pts',(33.8701936654629,-4.52131001657821,-0.00400076979791265));
#74235=CARTESIAN_POINT('Ctrl Pts',(33.8816291383803,-4.52498402972909,-0.437846630360423));
#74236=CARTESIAN_POINT('Ctrl Pts',(33.9328199354367,-4.26830215849308,-2.37569557039852));
#74237=CARTESIAN_POINT('Ctrl Pts',(34.0237660566323,-1.50016308523093,-5.13506383480611));
#74238=CARTESIAN_POINT('Ctrl Pts',(34.1430320290494,3.50707457935405,-4.03977694491552));
#74239=CARTESIAN_POINT('Ctrl Pts',(34.2622980014666,5.29487894566462,0.763954724174054));
#74240=CARTESIAN_POINT('Ctrl Pts',(34.3815639738838,2.22207678584961,4.86638928031932));
#74241=CARTESIAN_POINT('Ctrl Pts',(34.5008299463009,-2.89055310896428,4.5015633500008));
#74242=CARTESIAN_POINT('Ctrl Pts',(34.5803731768273,-4.53065996027806,1.50221304852085));
#74243=CARTESIAN_POINT('Ctrl Pts',(34.6201610832147,-4.53121771001937,0.00125226072096765));
#74244=CARTESIAN_POINT('Ctrl Pts',(34.620193665463,-4.53121761719171,2.31264352862156E-5));
#74245=CARTESIAN_POINT('Ctrl Pts',(34.0180063345368,-4.53096931099894,0.000962538283377154));
#74246=CARTESIAN_POINT('Ctrl Pts',(34.0563905632129,-4.52678360881868,-1.44725925730328));
#74247=CARTESIAN_POINT('Ctrl Pts',(34.134530116028,-2.98893814438493,-4.40307445317525));
#74248=CARTESIAN_POINT('Ctrl Pts',(34.252424992982,2.04905202712797,-4.94173617688352));
#74249=CARTESIAN_POINT('Ctrl Pts',(34.3716909653993,5.26463906194561,-0.95023481270979));
#74250=CARTESIAN_POINT('Ctrl Pts',(34.4909569378164,3.64737925647783,3.91356553684459));
#74251=CARTESIAN_POINT('Ctrl Pts',(34.6102229102336,-1.31811109383836,5.18478097860004));
#74252=CARTESIAN_POINT('Ctrl Pts',(34.7025727091403,-4.22605285621444,2.4837093520579));
#74253=CARTESIAN_POINT('Ctrl Pts',(34.7551671839081,-4.52357391933511,0.491140138321174));
#74254=CARTESIAN_POINT('Ctrl Pts',(34.7680063345368,-4.51988998684523,0.00365389551349841));
#74255=CARTESIAN_POINT('Origin',(-19.0048063345371,0.,0.));
#74256=CARTESIAN_POINT('',(33.1201936654629,-4.51698102336606,0.00183909419487934));
#74257=CARTESIAN_POINT('',(33.2680063345368,-4.52278493895671,-0.00415864970829849));
#74258=CARTESIAN_POINT('',(-19.0048063345371,-4.52375,5.14627461305311E-12));
#74259=CARTESIAN_POINT('Ctrl Pts',(33.1201936654629,-4.51698102336606,0.00183909419487933));
#74260=CARTESIAN_POINT('Ctrl Pts',(33.143097193546,-4.51380328422841,-0.869184672515116));
#74261=CARTESIAN_POINT('Ctrl Pts',(33.2057560457681,-3.85050608020546,-3.25658480382206));
#74262=CARTESIAN_POINT('Ctrl Pts',(33.3081702221293,0.0213580713928514,
-5.34966482152014));
#74263=CARTESIAN_POINT('Ctrl Pts',(33.4274361945464,4.51071386747616,-2.87625281843973));
#74264=CARTESIAN_POINT('Ctrl Pts',(33.5467021669636,4.85931300288409,2.23750910832247));
#74265=CARTESIAN_POINT('Ctrl Pts',(33.6659681393807,0.747147551098779,5.29727669720119));
#74266=CARTESIAN_POINT('Ctrl Pts',(33.7737986388806,-3.59084071708882,3.66711594592562));
#74267=CARTESIAN_POINT('Ctrl Pts',(33.8418738142413,-4.51221135432166,1.0704148064563));
#74268=CARTESIAN_POINT('Ctrl Pts',(33.8701936654629,-4.52131001657821,-0.00400076979791265));
#74269=CARTESIAN_POINT('Ctrl Pts',(33.2680063345368,-4.52278493895671,-0.00415864970829852));
#74270=CARTESIAN_POINT('Ctrl Pts',(33.2781032942395,-4.52624527943587,-0.386906023541205));
#74271=CARTESIAN_POINT('Ctrl Pts',(33.3279555780812,-4.3064402681918,-2.27274940851596));
#74272=CARTESIAN_POINT('Ctrl Pts',(33.417563186062,-1.67202789967526,-5.08170181676528));
#74273=CARTESIAN_POINT('Ctrl Pts',(33.536829158479,3.36921585264198,-4.15544885543223));
#74274=CARTESIAN_POINT('Ctrl Pts',(33.6560951308963,5.31757821346333,0.585433681563546));
#74275=CARTESIAN_POINT('Ctrl Pts',(33.7753611033134,2.38449651621095,4.78889830921323));
#74276=CARTESIAN_POINT('Ctrl Pts',(33.8946270757306,-2.73751139581363,4.59623781038317));
#74277=CARTESIAN_POINT('Ctrl Pts',(33.9755088194717,-4.50685179120484,1.60423335784827));
#74278=CARTESIAN_POINT('Ctrl Pts',(34.0166352390738,-4.53111882546014,0.0526934288572369));
#74279=CARTESIAN_POINT('Ctrl Pts',(34.0180063345368,-4.53096931099894,0.000962538283377154));
#74280=CARTESIAN_POINT('Origin',(-19.0048063345371,0.,0.));
#74281=CARTESIAN_POINT('',(32.3701936654629,-4.52806646847511,0.00326652668130843));
#74282=CARTESIAN_POINT('',(32.5180063345368,-4.51649463517031,0.0010498457038996));
#74283=CARTESIAN_POINT('',(-19.0048063345371,-4.52375,5.14627461305311E-12));
#74284=CARTESIAN_POINT('Ctrl Pts',(32.3701936654629,-4.52806646847511,0.00326652668130825));
#74285=CARTESIAN_POINT('Ctrl Pts',(32.4045652487117,-4.51749649868563,-1.29575333366401));
#74286=CARTESIAN_POINT('Ctrl Pts',(32.4786921560994,-3.24828895209341,-4.11528667960992));
#74287=CARTESIAN_POINT('Ctrl Pts',(32.5925743876263,1.54111720041119,-5.12292178784925));
#74288=CARTESIAN_POINT('Ctrl Pts',(32.7118403600434,5.14222206711005,-1.47543962341761));
#74289=CARTESIAN_POINT('Ctrl Pts',(32.8311063324606,4.02285675976709,3.52647038272272));
#74290=CARTESIAN_POINT('Ctrl Pts',(32.9503723048777,-0.789420891907063,
5.29114208137));
#74291=CARTESIAN_POINT('Ctrl Pts',(33.0467347492119,-4.09205124409713,2.79251416600766));
#74292=CARTESIAN_POINT('Ctrl Pts',(33.1033418694069,-4.51931911781478,0.642714806587559));
#74293=CARTESIAN_POINT('Ctrl Pts',(33.1201936654629,-4.51698102336606,0.00183909419487933));
#74294=CARTESIAN_POINT('Ctrl Pts',(32.5180063345368,-4.51649463517031,0.00104984570389918));
#74295=CARTESIAN_POINT('Ctrl Pts',(32.5395713494051,-4.51479700942663,-0.819290632073363));
#74296=CARTESIAN_POINT('Ctrl Pts',(32.6008916884125,-3.90820502976704,-3.15427603926576));
#74297=CARTESIAN_POINT('Ctrl Pts',(32.701967351559,-0.15858550575743,-5.34735647672489));
#74298=CARTESIAN_POINT('Ctrl Pts',(32.821233323976,4.41142146589973,-3.02633958801825));
#74299=CARTESIAN_POINT('Ctrl Pts',(32.9404992963933,4.93182046980722,2.07280426123612));
#74300=CARTESIAN_POINT('Ctrl Pts',(33.0597652688104,0.924894296461516,5.26914994967698));
#74301=CARTESIAN_POINT('Ctrl Pts',(33.168934281525,-3.51996685280539,3.76740329753486));
#74302=CARTESIAN_POINT('Ctrl Pts',(33.2383479701004,-4.51262068733767,1.12010661771242));
#74303=CARTESIAN_POINT('Ctrl Pts',(33.2680063345368,-4.52278493895671,-0.00415864970829852));
#74304=CARTESIAN_POINT('Origin',(-19.0048063345371,0.,0.));
#74305=CARTESIAN_POINT('',(31.6201936654629,-4.52734081159469,-0.00353972901762604));
#74306=CARTESIAN_POINT('',(31.7680063345368,-4.52664803363837,0.00374760370527943));
#74307=CARTESIAN_POINT('',(-19.0048063345371,-4.52375,5.14627461305311E-12));
#74308=CARTESIAN_POINT('Ctrl Pts',(31.6201936654629,-4.52734081159469,-0.00353972901762627));
#74309=CARTESIAN_POINT('Ctrl Pts',(31.6262779797383,-4.52931909355584,-0.233582775118892));
#74310=CARTESIAN_POINT('Ctrl Pts',(31.6721176181527,-4.40866889995517,-1.96466148405792));
#74311=CARTESIAN_POINT('Ctrl Pts',(31.7577125807061,-2.17514757970455,-4.88754569045954));
#74312=CARTESIAN_POINT('Ctrl Pts',(31.8769785531233,2.9337351189414,-4.47354089304141));
#74313=CARTESIAN_POINT('Ctrl Pts',(31.9962445255404,5.34950014457238,0.047096422840884));
#74314=CARTESIAN_POINT('Ctrl Pts',(32.1155104979576,2.85451733611025,4.52450004394633));
#74315=CARTESIAN_POINT('Ctrl Pts',(32.2347764703748,-2.26086260233548,4.84849153481623));
#74316=CARTESIAN_POINT('Ctrl Pts',(32.3196708595432,-4.42471940840208,1.91097730457275));
#74317=CARTESIAN_POINT('Ctrl Pts',(32.3648099245726,-4.52972207968608,0.206736535289742));
#74318=CARTESIAN_POINT('Ctrl Pts',(32.3701936654629,-4.52806646847511,0.00326652668130825));
#74319=CARTESIAN_POINT('Ctrl Pts',(31.7680063345368,-4.52664803363837,0.00374760370527919));
#74320=CARTESIAN_POINT('Ctrl Pts',(31.8010394045708,-4.51551060816241,-1.24570217322333));
#74321=CARTESIAN_POINT('Ctrl Pts',(31.8738277987439,-3.32900333837359,-4.01743474331935));
#74322=CARTESIAN_POINT('Ctrl Pts',(31.986371517056,1.36794009374822,-5.17185755330946));
#74323=CARTESIAN_POINT('Ctrl Pts',(32.1056374894731,5.08968755204155,-1.64755918691883));
#74324=CARTESIAN_POINT('Ctrl Pts',(32.2249034618903,4.13919060489128,3.3891697786018));
#74325=CARTESIAN_POINT('Ctrl Pts',(32.3441694343074,-0.611011127479355,
5.31469999660417));
#74326=CARTESIAN_POINT('Ctrl Pts',(32.4418703918563,-4.04282844254874,2.89542259591036));
#74327=CARTESIAN_POINT('Ctrl Pts',(32.4998160252661,-4.51792659974311,0.693015378267232));
#74328=CARTESIAN_POINT('Ctrl Pts',(32.5180063345368,-4.51649463517031,0.00104984570389918));
#74329=CARTESIAN_POINT('Origin',(-19.0048063345371,0.,0.));
#74330=CARTESIAN_POINT('',(30.8701936654629,-4.51669300721655,-0.00143314003944115));
#74331=CARTESIAN_POINT('',(31.0180063345369,-4.52868647542216,-0.00297892043936654));
#74332=CARTESIAN_POINT('',(-19.0048063345371,-4.52375,5.14627461305311E-12));
#74333=CARTESIAN_POINT('Ctrl Pts',(30.870193665463,-4.51669300721655,-0.00143314003944142));
#74334=CARTESIAN_POINT('Ctrl Pts',(30.887746034904,-4.51858387894054,-0.669058025820529));
#74335=CARTESIAN_POINT('Ctrl Pts',(30.945053728484,-4.06657764023515,-2.84638774123857));
#74336=CARTESIAN_POINT('Ctrl Pts',(31.0421167462031,-0.696140458765788,
-5.30422080342567));
#74337=CARTESIAN_POINT('Ctrl Pts',(31.1613827186203,4.08432171488679,-3.45509565701559));
#74338=CARTESIAN_POINT('Ctrl Pts',(31.2806486910375,5.11544778739555,1.56574704350808));
#74339=CARTESIAN_POINT('Ctrl Pts',(31.3999146634546,1.45068200768019,5.14926126569795));
#74340=CARTESIAN_POINT('Ctrl Pts',(31.5130963215965,-3.29089145935549,4.06417453521408));
#74341=CARTESIAN_POINT('Ctrl Pts',(31.5865226555992,-4.51639286439593,1.26953416622099));
#74342=CARTESIAN_POINT('Ctrl Pts',(31.6201936654629,-4.52734081159469,-0.00353972901762627));
#74343=CARTESIAN_POINT('Ctrl Pts',(31.0180063345369,-4.52868647542216,-0.00297892043936619));
#74344=CARTESIAN_POINT('Ctrl Pts',(31.0227521355974,-4.53004991495928,-0.182274828229998));
#74345=CARTESIAN_POINT('Ctrl Pts',(31.0672532607971,-4.43888415483644,-1.86212428583227));
#74346=CARTESIAN_POINT('Ctrl Pts',(31.1515097101358,-2.33830543955411,-4.81162117411165));
#74347=CARTESIAN_POINT('Ctrl Pts',(31.270775682553,2.78161148635255,-4.56968359854373));
#74348=CARTESIAN_POINT('Ctrl Pts',(31.3900416549701,5.34805758082949,-0.132856177649306));
#74349=CARTESIAN_POINT('Ctrl Pts',(31.5093076273873,3.00508008957021,4.42593089723243));
#74350=CARTESIAN_POINT('Ctrl Pts',(31.6285735998045,-2.09650851344057,4.92179059945456));
#74351=CARTESIAN_POINT('Ctrl Pts',(31.7148065021876,-4.39359747073332,2.01357634362355));
#74352=CARTESIAN_POINT('Ctrl Pts',(31.7612840804318,-4.52891450793364,0.258011554449596));
#74353=CARTESIAN_POINT('Ctrl Pts',(31.7680063345368,-4.52664803363837,0.00374760370527919));
#74354=CARTESIAN_POINT('Origin',(-19.0048063345371,0.,0.));
#74355=CARTESIAN_POINT('',(30.1201936654629,-4.52207059346122,0.00410535199279809));
#74356=CARTESIAN_POINT('',(30.2680063345368,-4.51730521221276,-0.00219145969648615));
#74357=CARTESIAN_POINT('',(-19.0048063345371,-4.52375,5.14627461305311E-12));
#74358=CARTESIAN_POINT('Ctrl Pts',(30.1201936654629,-4.52207059346122,0.00410535199279808));
#74359=CARTESIAN_POINT('Ctrl Pts',(30.1492140900696,-4.51237828040898,-1.09641936695486));
#74360=CARTESIAN_POINT('Ctrl Pts',(30.2179898388154,-3.55408529374172,-3.71967609856161));
#74361=CARTESIAN_POINT('Ctrl Pts',(30.3265209117001,0.840297817034937,-5.28330099923434));
#74362=CARTESIAN_POINT('Ctrl Pts',(30.4457868841173,4.89795430972499,-2.15160717829025));
#74363=CARTESIAN_POINT('Ctrl Pts',(30.5650528565345,4.45937416947051,2.95522450695096));
#74364=CARTESIAN_POINT('Ctrl Pts',(30.6843188289516,-0.0728336840866598,
5.34921163577276));
#74365=CARTESIAN_POINT('Ctrl Pts',(30.7860324319278,-3.88101638918563,3.2030683936662));
#74366=CARTESIAN_POINT('Ctrl Pts',(30.8479907107649,-4.5143011398753,0.843082191301476));
#74367=CARTESIAN_POINT('Ctrl Pts',(30.870193665463,-4.51669300721655,-0.00143314003944142));
#74368=CARTESIAN_POINT('Ctrl Pts',(30.2680063345368,-4.51730521221276,-0.00219145969648581));
#74369=CARTESIAN_POINT('Ctrl Pts',(30.2842201907631,-4.5199969460127,-0.618695688963642));
#74370=CARTESIAN_POINT('Ctrl Pts',(30.3401893711284,-4.11470020632812,-2.74343937300367));
#74371=CARTESIAN_POINT('Ctrl Pts',(30.4359138756328,-0.874149621850558,
-5.27780570790802));
#74372=CARTESIAN_POINT('Ctrl Pts',(30.55517984805,3.96580166144261,-3.59051358915504));
#74373=CARTESIAN_POINT('Ctrl Pts',(30.6744458204671,5.16521618558982,1.39280738364225));
#74374=CARTESIAN_POINT('Ctrl Pts',(30.7937117928843,1.62305233596266,5.09755546968683));
#74375=CARTESIAN_POINT('Ctrl Pts',(30.9082319642409,-3.20880931129668,4.16162230541739));
#74376=CARTESIAN_POINT('Ctrl Pts',(30.9829968114584,-4.5186284541668,1.31967749552273));
#74377=CARTESIAN_POINT('Ctrl Pts',(31.0180063345369,-4.52868647542216,-0.00297892043936619));
#74378=CARTESIAN_POINT('Origin',(-19.0048063345371,0.,0.));
#74379=CARTESIAN_POINT('',(29.3701936654629,-4.53114466631056,-0.000518721095705797));
#74380=CARTESIAN_POINT('',(29.5180063345369,-4.52064530787469,0.00386511480189006));
#74381=CARTESIAN_POINT('',(-19.0048063345371,-4.52375,5.14627461305311E-12));
#74382=CARTESIAN_POINT('Ctrl Pts',(29.3701936654629,-4.53114466631056,-0.000518721095705719));
#74383=CARTESIAN_POINT('Ctrl Pts',(29.3709268210962,-4.53118943009193,-0.0281775193443082));
#74384=CARTESIAN_POINT('Ctrl Pts',(29.4114153008686,-4.51841712149835,-1.55559068039991));
#74385=CARTESIAN_POINT('Ctrl Pts',(29.49165910478,-2.81084864442134,-4.55175787668666));
#74386=CARTESIAN_POINT('Ctrl Pts',(29.6109250771972,2.30741204557965,-4.82651214871964));
#74387=CARTESIAN_POINT('Ctrl Pts',(29.7301910496143,5.30750872044597,-0.670612445614996));
#74388=CARTESIAN_POINT('Ctrl Pts',(29.8494570220315,3.43540495621067,4.10089778666421));
#74389=CARTESIAN_POINT('Ctrl Pts',(29.9687229944486,-1.59034064221755,5.10785537300494));
#74390=CARTESIAN_POINT('Ctrl Pts',(30.0589685422591,-4.28852214464261,2.32180582197069));
#74391=CARTESIAN_POINT('Ctrl Pts',(30.1094587659306,-4.52565586170806,0.411198716439513));
#74392=CARTESIAN_POINT('Ctrl Pts',(30.1201936654629,-4.52207059346122,0.00410535199279808));
#74393=CARTESIAN_POINT('Ctrl Pts',(29.5180063345369,-4.52064530787469,0.0038651148018904));
#74394=CARTESIAN_POINT('Ctrl Pts',(29.5456882459288,-4.51214506679005,-1.04673871353975));
#74395=CARTESIAN_POINT('Ctrl Pts',(29.6131254814597,-3.62366603379782,-3.61912902093094));
#74396=CARTESIAN_POINT('Ctrl Pts',(29.7203180411298,0.662122995951101,-5.30857455349746));
#74397=CARTESIAN_POINT('Ctrl Pts',(29.839584013547,4.8228156661174,-2.31512844189271));
#74398=CARTESIAN_POINT('Ctrl Pts',(29.9588499859641,4.55624766770592,2.8035652020832));
#74399=CARTESIAN_POINT('Ctrl Pts',(30.0781159583813,0.107123774146093,5.34863488647531));
#74400=CARTESIAN_POINT('Ctrl Pts',(30.1811680745722,-3.822123913385,3.3052499950529));
#74401=CARTESIAN_POINT('Ctrl Pts',(30.2444648666241,-4.51339698927079,0.89293270625552));
#74402=CARTESIAN_POINT('Ctrl Pts',(30.2680063345368,-4.51730521221276,-0.00219145969648581));
#74403=CARTESIAN_POINT('Origin',(-19.0048063345371,0.,0.));
#74404=CARTESIAN_POINT('',(28.6201936654629,-4.52051575184804,-0.0038334580682193));
#74405=CARTESIAN_POINT('',(28.7680063345369,-4.53116771210378,0.000428735186510879));
#74406=CARTESIAN_POINT('',(-19.0048063345371,-4.52375,5.14627461305311E-12));
#74407=CARTESIAN_POINT('Ctrl Pts',(28.6201936654629,-4.52051575184804,-0.00383345806821922));
#74408=CARTESIAN_POINT('Ctrl Pts',(28.6323948762619,-4.52422411022693,-0.466936104215469));
#74409=CARTESIAN_POINT('Ctrl Pts',(28.6843514111999,-4.24554373484115,-2.43461423389684));
#74410=CARTESIAN_POINT('Ctrl Pts',(28.7760632702771,-1.4010666075983,-5.1629819127029));
#74411=CARTESIAN_POINT('Ctrl Pts',(28.8953292426941,3.58416621553077,-3.97153904793497));
#74412=CARTESIAN_POINT('Ctrl Pts',(29.0145952151114,5.27919696290035,0.865707396715219));
#74413=CARTESIAN_POINT('Ctrl Pts',(29.1338611875285,2.12801697082046,4.90824954965865));
#74414=CARTESIAN_POINT('Ctrl Pts',(29.2523940043124,-2.94526594078766,4.44795128087226));
#74415=CARTESIAN_POINT('Ctrl Pts',(29.3311714969572,-4.52876211649412,1.47161930378696));
#74416=CARTESIAN_POINT('Ctrl Pts',(29.3701936654629,-4.53114466631056,-0.000518721095705719));
#74417=CARTESIAN_POINT('Ctrl Pts',(28.7680063345369,-4.53116771210378,0.000428735186511165));
#74418=CARTESIAN_POINT('Ctrl Pts',(28.8071563010945,-4.5291761204828,-1.47651041274696));
#74419=CARTESIAN_POINT('Ctrl Pts',(28.8860615917911,-2.93643577703342,-4.45690962027768));
#74420=CARTESIAN_POINT('Ctrl Pts',(29.0047222066268,2.14377087841479,-4.90138930025648));
#74421=CARTESIAN_POINT('Ctrl Pts',(29.123988179044,5.28195037803777,-0.848746638140402));
#74422=CARTESIAN_POINT('Ctrl Pts',(29.2432541514612,3.57139155113628,3.98303063511691));
#74423=CARTESIAN_POINT('Ctrl Pts',(29.3625201238783,-1.41764243240855,5.15845525187946));
#74424=CARTESIAN_POINT('Ctrl Pts',(29.4541041849036,-4.24939018309867,2.42478002480354));
#74425=CARTESIAN_POINT('Ctrl Pts',(29.5059329217897,-4.52435267177785,0.462083966588632));
#74426=CARTESIAN_POINT('Ctrl Pts',(29.5180063345369,-4.52064530787469,0.0038651148018904));
#74427=CARTESIAN_POINT('Origin',(-19.0048063345371,0.,0.));
#74428=CARTESIAN_POINT('',(27.870193665463,-4.51737697201026,0.00225976351037011));
#74429=CARTESIAN_POINT('',(28.0180063345369,-4.52192984201937,-0.00408982420865234));
#74430=CARTESIAN_POINT('',(-19.0048063345371,-4.52375,5.14627461305311E-12));
#74431=CARTESIAN_POINT('Ctrl Pts',(27.870193665463,-4.51737697201026,0.00225976351037008));
#74432=CARTESIAN_POINT('Ctrl Pts',(27.8938629314276,-4.51332129582812,-0.8976879117203));
#74433=CARTESIAN_POINT('Ctrl Pts',(27.9572875215313,-3.81636887415937,-3.31499081853051));
#74434=CARTESIAN_POINT('Ctrl Pts',(28.060467435774,0.124302552914632,-5.34826315219841));
#74435=CARTESIAN_POINT('Ctrl Pts',(28.1797334081912,4.56522890198429,-2.78891644591795));
#74436=CARTESIAN_POINT('Ctrl Pts',(28.2989993806083,4.81535473947628,2.33060691727008));
#74437=CARTESIAN_POINT('Ctrl Pts',(28.4182653530255,0.645068908923938,5.31067377764479));
#74438=CARTESIAN_POINT('Ctrl Pts',(28.5253301146437,-3.6301684636346,3.60950202170377));
#74439=CARTESIAN_POINT('Ctrl Pts',(28.5926395521229,-4.51214112995506,1.04199576415337));
#74440=CARTESIAN_POINT('Ctrl Pts',(28.6201936654629,-4.52051575184804,-0.00383345806821922));
#74441=CARTESIAN_POINT('Ctrl Pts',(28.0180063345369,-4.52192984201937,-0.0040898242086522));
#74442=CARTESIAN_POINT('Ctrl Pts',(28.0288690321211,-4.52553520025187,-0.416062179398293));
#74443=CARTESIAN_POINT('Ctrl Pts',(28.0794870538443,-4.28487623826261,-2.3316351509503));
#74444=CARTESIAN_POINT('Ctrl Pts',(28.1698603997067,-1.57392648948877,-5.11293712629961));
#74445=CARTESIAN_POINT('Ctrl Pts',(28.2891263721238,3.44855899679427,-4.08984247831593));
#74446=CARTESIAN_POINT('Ctrl Pts',(28.408392344541,5.30532746904341,0.687656235354114));
#74447=CARTESIAN_POINT('Ctrl Pts',(28.5276583169582,2.291897852936,4.83389851812331));
#74448=CARTESIAN_POINT('Ctrl Pts',(28.6469242893753,-2.82545402003632,4.54270626746531));
#74449=CARTESIAN_POINT('Ctrl Pts',(28.7270402952349,-4.52068612267638,1.54585040122244));
#74450=CARTESIAN_POINT('Ctrl Pts',(28.7674009769554,-4.53119850715146,0.0232659529202972));
#74451=CARTESIAN_POINT('Ctrl Pts',(28.7680063345369,-4.53116771210378,0.000428735186511165));
#74452=CARTESIAN_POINT('Origin',(-19.0048063345371,0.,0.));
#74453=CARTESIAN_POINT('',(27.120193665463,-4.52880516386923,0.00291706699860573));
#74454=CARTESIAN_POINT('',(27.2680063345369,-4.51674019473067,0.00150848591183417));
#74455=CARTESIAN_POINT('',(-19.0048063345371,-4.52375,5.14627461305311E-12));
#74456=CARTESIAN_POINT('Ctrl Pts',(27.120193665463,-4.52880516386923,0.0029170669986057));
#74457=CARTESIAN_POINT('Ctrl Pts',(27.1553309865932,-4.51887004847389,-1.32447633190377));
#74458=CARTESIAN_POINT('Ctrl Pts',(27.2302236318626,-3.2008213721839,-4.17088006383837));
#74459=CARTESIAN_POINT('Ctrl Pts',(27.344871601271,1.63941683012594,-5.09231600815622));
#74460=CARTESIAN_POINT('Ctrl Pts',(27.4641375736882,5.16966304351028,-1.37620997176607));
#74461=CARTESIAN_POINT('Ctrl Pts',(27.5834035461054,3.95424874510512,3.60323281674365));
#74462=CARTESIAN_POINT('Ctrl Pts',(27.7026695185225,-0.891096936738138,
5.27497072211403));
#74463=CARTESIAN_POINT('Ctrl Pts',(27.7982662249751,-4.11917516279323,2.73360655033951));
#74464=CARTESIAN_POINT('Ctrl Pts',(27.8541076072885,-4.52013328237071,0.61388036379995));
#74465=CARTESIAN_POINT('Ctrl Pts',(27.870193665463,-4.51737697201026,0.00225976351037008));
#74466=CARTESIAN_POINT('Ctrl Pts',(27.2680063345368,-4.51674019473067,0.00150848591183396));
#74467=CARTESIAN_POINT('Ctrl Pts',(27.2903370872867,-4.51420659348407,-0.847845685554157));
#74468=CARTESIAN_POINT('Ctrl Pts',(27.3524231641757,-3.8755018834822,-3.21283625088979));
#74469=CARTESIAN_POINT('Ctrl Pts',(27.4542645652037,-0.0556521236575815,
-5.34941805180156));
#74470=CARTESIAN_POINT('Ctrl Pts',(27.5735305376208,4.46884314287686,-2.94088619571898));
#74471=CARTESIAN_POINT('Ctrl Pts',(27.692796510038,4.89101834366639,2.16732789714115));
#74472=CARTESIAN_POINT('Ctrl Pts',(27.8120624824552,0.823324007385604,5.2859727799782));
#74473=CARTESIAN_POINT('Ctrl Pts',(27.9204657572881,-3.5608457184922,3.71009937882906));
#74474=CARTESIAN_POINT('Ctrl Pts',(27.989113707982,-4.51234030238609,1.09167513814337));
#74475=CARTESIAN_POINT('Ctrl Pts',(28.0180063345369,-4.52192984201937,-0.0040898242086522));
#74476=CARTESIAN_POINT('Origin',(-19.0048063345371,0.,0.));
#74477=CARTESIAN_POINT('',(26.370193665463,-4.52650623014407,-0.00378441848545811));
#74478=CARTESIAN_POINT('',(26.5180063345369,-4.52747628307774,0.00349333724076611));
#74479=CARTESIAN_POINT('',(-19.0048063345371,-4.52375,5.14627461305311E-12));
#74480=CARTESIAN_POINT('Ctrl Pts',(26.370193665463,-4.52650623014407,-0.00378441848545744));
#74481=CARTESIAN_POINT('Ctrl Pts',(26.3770437176199,-4.52882920222418,-0.262903224669573));
#74482=CARTESIAN_POINT('Ctrl Pts',(26.4236490939158,-4.39052545737866,-2.02337872152482));
#74483=CARTESIAN_POINT('Ctrl Pts',(26.5100097943509,-2.08068932314761,-4.92849894089096));
#74484=CARTESIAN_POINT('Ctrl Pts',(26.629275766768,3.01928023853817,-4.41625596076554));
#74485=CARTESIAN_POINT('Ctrl Pts',(26.7485417391852,5.34760319937945,0.1500329690799));
#74486=CARTESIAN_POINT('Ctrl Pts',(26.8678077116024,2.76691968873083,4.57859424997864));
#74487=CARTESIAN_POINT('Ctrl Pts',(26.9870736840195,-2.35374783936478,4.80408586294104));
#74488=CARTESIAN_POINT('Ctrl Pts',(27.0712023353064,-4.4416704537898,1.85234129232427));
#74489=CARTESIAN_POINT('Ctrl Pts',(27.1155756624542,-4.53011090919392,0.177372788514735));
#74490=CARTESIAN_POINT('Ctrl Pts',(27.120193665463,-4.52880516386923,0.0029170669986057));
#74491=CARTESIAN_POINT('Ctrl Pts',(26.5180063345369,-4.52747628307774,0.00349333724076601));
#74492=CARTESIAN_POINT('Ctrl Pts',(26.5518051424524,-4.51658359282757,-1.27431317611325));
#74493=CARTESIAN_POINT('Ctrl Pts',(26.625359274507,-3.28317857968101,-4.07351566037758));
#74494=CARTESIAN_POINT('Ctrl Pts',(26.7386687307007,1.4672135077607,-5.14457531526681));
#74495=CARTESIAN_POINT('Ctrl Pts',(26.8579347031179,5.12045050920806,-1.54930863115098));
#74496=CARTESIAN_POINT('Ctrl Pts',(26.977200675535,4.073203247058,3.46819635545099));
#74497=CARTESIAN_POINT('Ctrl Pts',(27.0964666479522,-0.713173556682066,
5.30195757526005));
#74498=CARTESIAN_POINT('Ctrl Pts',(27.1934018676195,-4.0712717902843,2.83656196042909));
#74499=CARTESIAN_POINT('Ctrl Pts',(27.2505817631477,-4.51871715073782,0.664255172562189));
#74500=CARTESIAN_POINT('Ctrl Pts',(27.2680063345368,-4.51674019473067,0.00150848591183396));
#74501=CARTESIAN_POINT('Origin',(-19.0048063345371,0.,0.));
#74502=CARTESIAN_POINT('',(25.620193665463,-4.51646227191973,-0.000971816212263622));
#74503=CARTESIAN_POINT('',(25.7680063345369,-4.52793736187105,-0.0033197696265741));
#74504=CARTESIAN_POINT('',(-19.0048063345371,-4.52375,5.14627461305311E-12));
#74505=CARTESIAN_POINT('Ctrl Pts',(25.620193665463,-4.51646227191973,-0.000971816212263291));
#74506=CARTESIAN_POINT('Ctrl Pts',(25.6385117727855,-4.51779658626017,-0.697811251222172));
#74507=CARTESIAN_POINT('Ctrl Pts',(25.6965852042472,-4.038006838103,-2.90524271252507));
#74508=CARTESIAN_POINT('Ctrl Pts',(25.7944139598479,-0.593937630424711,
-5.31663502236041));
#74509=CARTESIAN_POINT('Ctrl Pts',(25.9136799322651,4.15005490520629,-3.37585754343952));
#74510=CARTESIAN_POINT('Ctrl Pts',(26.0329459046822,5.08436941740803,1.66389828329445));
#74511=CARTESIAN_POINT('Ctrl Pts',(26.1522118770994,1.35132147900805,5.17622450538955));
#74512=CARTESIAN_POINT('Ctrl Pts',(26.2646277973596,-3.3365604235817,4.00804952635544));
#74513=CARTESIAN_POINT('Ctrl Pts',(26.3372883934808,-4.51534747888903,1.24093235123574));
#74514=CARTESIAN_POINT('Ctrl Pts',(26.370193665463,-4.52650623014407,-0.00378441848545744));
#74515=CARTESIAN_POINT('Ctrl Pts',(25.7680063345369,-4.52793736187105,-0.00331976962657424));
#74516=CARTESIAN_POINT('Ctrl Pts',(25.773517873479,-4.5296519411211,-0.211635204411083));
#74517=CARTESIAN_POINT('Ctrl Pts',(25.8187847365603,-4.42183036494298,-1.92076769273718));
#74518=CARTESIAN_POINT('Ctrl Pts',(25.9038069237805,-2.24527805335948,-4.85572827852936));
#74519=CARTESIAN_POINT('Ctrl Pts',(26.0230728961977,2.86903493736783,-4.51530831505123));
#74520=CARTESIAN_POINT('Ctrl Pts',(26.1423388686148,5.34962389335311,-0.0299140681537413));
#74521=CARTESIAN_POINT('Ctrl Pts',(26.2616048410321,2.91935141602282,4.48294077158877));
#74522=CARTESIAN_POINT('Ctrl Pts',(26.3808708134492,-2.19083474590394,4.88053416830044));
#74523=CARTESIAN_POINT('Ctrl Pts',(26.4663379779508,-4.4116357972034,1.95486584720251));
#74524=CARTESIAN_POINT('Ctrl Pts',(26.5120498183134,-4.52939595096529,0.22868693715409));
#74525=CARTESIAN_POINT('Ctrl Pts',(26.5180063345369,-4.52747628307774,0.00349333724076601));
#74526=CARTESIAN_POINT('Origin',(-19.0048063345371,0.,0.));
#74527=CARTESIAN_POINT('',(24.870193665463,-4.52292991114911,0.00416441657176817));
#74528=CARTESIAN_POINT('',(25.0180063345369,-4.51692316959201,-0.00176640309098947));
#74529=CARTESIAN_POINT('',(-19.0048063345371,-4.52375,5.14627461305311E-12));
#74530=CARTESIAN_POINT('Ctrl Pts',(24.870193665463,-4.52292991114911,0.00416441657176813));
#74531=CARTESIAN_POINT('Ctrl Pts',(24.8999798279512,-4.51267992564295,-1.12485307430951));
#74532=CARTESIAN_POINT('Ctrl Pts',(24.9695213145785,-3.51305705825671,-3.77694834013157));
#74533=CARTESIAN_POINT('Ctrl Pts',(25.0788181253449,0.941813547390232,-5.2661520213317));
#74534=CARTESIAN_POINT('Ctrl Pts',(25.1980840977621,4.93845262345068,-2.05695297849937));
#74535=CARTESIAN_POINT('Ctrl Pts',(25.3173500701792,4.40167832088221,3.04049302405052));
#74536=CARTESIAN_POINT('Ctrl Pts',(25.4366160425964,-0.175759912236459,
5.34681945861972));
#74537=CARTESIAN_POINT('Ctrl Pts',(25.537563907691,-3.91358405387219,3.14449502406534));
#74538=CARTESIAN_POINT('Ctrl Pts',(25.5987564486465,-4.51490075765882,0.814521716580516));
#74539=CARTESIAN_POINT('Ctrl Pts',(25.620193665463,-4.51646227191973,-0.000971816212263291));
#74540=CARTESIAN_POINT('Ctrl Pts',(25.0180063345369,-4.51692316959201,-0.00176640309098988));
#74541=CARTESIAN_POINT('Ctrl Pts',(25.0349859286447,-4.51918422158869,-0.647522979345086));
#74542=CARTESIAN_POINT('Ctrl Pts',(25.0917208468916,-4.08745153246059,-2.80234344813435));
#74543=CARTESIAN_POINT('Ctrl Pts',(25.1882110892776,-0.772422159146575,
-5.29365040967637));
#74544=CARTESIAN_POINT('Ctrl Pts',(25.3074770616947,4.03416276912766,-3.51353118728043));
#74545=CARTESIAN_POINT('Ctrl Pts',(25.4267430341119,5.13745663366157,1.49194838686019));
#74546=CARTESIAN_POINT('Ctrl Pts',(25.546009006529,1.52465490894722,5.12784536237498));
#74547=CARTESIAN_POINT('Ctrl Pts',(25.659763440004,-3.25611918384849,4.10598031695728));
#74548=CARTESIAN_POINT('Ctrl Pts',(25.73376254934,-4.51728449628163,1.2909664681739));
#74549=CARTESIAN_POINT('Ctrl Pts',(25.7680063345369,-4.52793736187105,-0.00331976962657424));
#74550=CARTESIAN_POINT('Origin',(-19.0048063345371,0.,0.));
#74551=CARTESIAN_POINT('',(24.120193665463,-4.53092246829786,-0.00105004667653403));
#74552=CARTESIAN_POINT('',(24.2680063345369,-4.52144663499091,0.00402336840721218));
#74553=CARTESIAN_POINT('',(-19.0048063345371,-4.52375,5.14627461305311E-12));
#74554=CARTESIAN_POINT('Ctrl Pts',(24.120193665463,-4.53092246829786,-0.00105004667653446));
#74555=CARTESIAN_POINT('Ctrl Pts',(24.1216925589779,-4.53109947999406,-0.0576042696761754));
#74556=CARTESIAN_POINT('Ctrl Pts',(24.1629467766318,-4.50448666451256,-1.61398211810567));
#74557=CARTESIAN_POINT('Ctrl Pts',(24.2439563184247,-2.72273453653836,-4.60500667897073));
#74558=CARTESIAN_POINT('Ctrl Pts',(24.3632222908419,2.39986569333583,-4.78121475399025));
#74559=CARTESIAN_POINT('Ctrl Pts',(24.4824882632591,5.31943107188467,-0.568351072218813));
#74560=CARTESIAN_POINT('Ctrl Pts',(24.6017542356763,3.35585150064429,4.16624898145168));
#74561=CARTESIAN_POINT('Ctrl Pts',(24.7210202080934,-1.6883412200409,5.0763051321345));
#74562=CARTESIAN_POINT('Ctrl Pts',(24.8105000180223,-4.30997355915991,2.2629239214585));
#74563=CARTESIAN_POINT('Ctrl Pts',(24.8602245038122,-4.52636048944094,0.38203645287768));
#74564=CARTESIAN_POINT('Ctrl Pts',(24.870193665463,-4.52292991114911,0.00416441657176813));
#74565=CARTESIAN_POINT('Ctrl Pts',(24.2680063345369,-4.52144663499091,0.00402336840721242));
#74566=CARTESIAN_POINT('Ctrl Pts',(24.2964539838104,-4.51223436788339,-1.07515811813252));
#74567=CARTESIAN_POINT('Ctrl Pts',(24.364656957223,-3.58419125381158,-3.67671503401053));
#74568=CARTESIAN_POINT('Ctrl Pts',(24.4726152547746,0.764158082763927,-5.29484967457566));
#74569=CARTESIAN_POINT('Ctrl Pts',(24.5918812271917,4.86647468160752,-2.22188992190905));
#74570=CARTESIAN_POINT('Ctrl Pts',(24.7111471996089,4.50145239709396,2.89072602792189));
#74571=CARTESIAN_POINT('Ctrl Pts',(24.8304131720261,0.00417532019002488,
5.34970590018823));
#74572=CARTESIAN_POINT('Ctrl Pts',(24.9326995503354,-3.85612301657671,3.24682793721983));
#74573=CARTESIAN_POINT('Ctrl Pts',(24.9952306045057,-4.51389028732547,0.864424941250599));
#74574=CARTESIAN_POINT('Ctrl Pts',(25.0180063345369,-4.51692316959201,-0.00176640309098988));
#74575=CARTESIAN_POINT('Origin',(-19.0048063345371,0.,0.));
#74576=CARTESIAN_POINT('',(23.370193665463,-4.51976894652972,-0.00361372362653868));
#74577=CARTESIAN_POINT('',(23.5180063345369,-4.53121424191125,-0.000113818667257792));
#74578=CARTESIAN_POINT('',(-19.0048063345371,-4.52375,5.14627461305311E-12));
#74579=CARTESIAN_POINT('Ctrl Pts',(23.370193665463,-4.51976894652972,-0.00361372362653871));
#74580=CARTESIAN_POINT('Ctrl Pts',(23.3831606141435,-4.52344198664446,-0.495985503601568));
#74581=CARTESIAN_POINT('Ctrl Pts',(23.4358828869631,-4.22208968250827,-2.49354528016135));
#74582=CARTESIAN_POINT('Ctrl Pts',(23.5283604839218,-1.30145122794406,-5.1889878175909));
#74583=CARTESIAN_POINT('Ctrl Pts',(23.6476264563389,3.65993041225227,-3.90183024326985));
#74584=CARTESIAN_POINT('Ctrl Pts',(23.7668924287561,5.26155976547379,0.967139444016044));
#74585=CARTESIAN_POINT('Ctrl Pts',(23.8861584011732,2.03316901887958,4.94829198921123));
#74586=CARTESIAN_POINT('Ctrl Pts',(24.0039254800755,-2.99760568614095,4.39405292852535));
#74587=CARTESIAN_POINT('Ctrl Pts',(24.0819372348388,-4.52640457852891,1.44238985563963));
#74588=CARTESIAN_POINT('Ctrl Pts',(24.120193665463,-4.53092246829786,-0.00105004667653446));
#74589=CARTESIAN_POINT('Ctrl Pts',(23.5180063345369,-4.53121424191125,-0.000113818667257794));
#74590=CARTESIAN_POINT('Ctrl Pts',(23.518166714837,-4.53121647143214,-0.00616402523120993));
#74591=CARTESIAN_POINT('Ctrl Pts',(23.5580824192762,-4.52846221956104,-1.51194697710339));
#74592=CARTESIAN_POINT('Ctrl Pts',(23.6377534478544,-2.87607962259252,-4.51082438766087));
#74593=CARTESIAN_POINT('Ctrl Pts',(23.7570194202716,2.2376957581383,-4.85922713461897));
#74594=CARTESIAN_POINT('Ctrl Pts',(23.8762853926887,5.2973054597101,-0.746944119953741));
#74595=CARTESIAN_POINT('Ctrl Pts',(23.9955513651059,3.49408113758448,4.05102056965703));
#74596=CARTESIAN_POINT('Ctrl Pts',(24.1148173375231,-1.51664872988588,5.13021902865199));
#74597=CARTESIAN_POINT('Ctrl Pts',(24.2056356606667,-4.27203338814583,2.3658639017595));
#74598=CARTESIAN_POINT('Ctrl Pts',(24.2566986596713,-4.52510842511722,0.432987929006955));
#74599=CARTESIAN_POINT('Ctrl Pts',(24.2680063345369,-4.52144663499091,0.00402336840721242));
#74600=CARTESIAN_POINT('Origin',(-19.0048063345371,0.,0.));
#74601=CARTESIAN_POINT('',(22.620193665463,-4.51785376865908,0.00265090740345769));
#74602=CARTESIAN_POINT('',(22.7680063345369,-4.52110593686914,-0.00396372416147706));
#74603=CARTESIAN_POINT('',(-19.0048063345371,-4.52375,5.14627461305311E-12));
#74604=CARTESIAN_POINT('Ctrl Pts',(22.620193665463,-4.51785376865908,0.0026509074034578));
#74605=CARTESIAN_POINT('Ctrl Pts',(22.6446286693092,-4.51291135001306,-0.926166110723544));
#74606=CARTESIAN_POINT('Ctrl Pts',(22.7088189972944,-3.78139899895146,-3.37329467135839));
#74607=CARTESIAN_POINT('Ctrl Pts',(22.8127646494188,0.227200997477541,-5.34488068871223));
#74608=CARTESIAN_POINT('Ctrl Pts',(22.9320306218359,4.61805314856548,-2.70054716434442));
#74609=CARTESIAN_POINT('Ctrl Pts',(23.0512965942531,4.76961305100215,2.42284155766206));
#74610=CARTESIAN_POINT('Ctrl Pts',(23.1705625666702,0.542751357650036,5.32210398560502));
#74611=CARTESIAN_POINT('Ctrl Pts',(23.2768615904069,-3.6686200124915,3.55172811343481));
#74612=CARTESIAN_POINT('Ctrl Pts',(23.3434052900045,-4.51218082536938,1.01357547269836));
#74613=CARTESIAN_POINT('Ctrl Pts',(23.370193665463,-4.51976894652972,-0.00361372362653871));
#74614=CARTESIAN_POINT('Ctrl Pts',(22.7680063345369,-4.52110593686913,-0.00396372416147671));
#74615=CARTESIAN_POINT('Ctrl Pts',(22.7796347700027,-4.52479494802337,-0.445180761673963));
#74616=CARTESIAN_POINT('Ctrl Pts',(22.8310185296075,-4.26263226036918,-2.39054140945846));
#74617=CARTESIAN_POINT('Ctrl Pts',(22.9221576133515,-1.47524215652576,-5.14227879751937));
#74618=CARTESIAN_POINT('Ctrl Pts',(23.0414235857686,3.52662492527076,-4.02272137840373));
#74619=CARTESIAN_POINT('Ctrl Pts',(23.1606895581858,5.29111183221057,0.789624107312617));
#74620=CARTESIAN_POINT('Ctrl Pts',(23.2799555306029,2.19845035747676,4.87710843405375));
#74621=CARTESIAN_POINT('Ctrl Pts',(23.39906112272,-2.90547756613246,4.48801620593015));
#74622=CARTESIAN_POINT('Ctrl Pts',(23.4784113906979,-4.53066381424317,1.49357081045434));
#74623=CARTESIAN_POINT('Ctrl Pts',(23.5180063345369,-4.53121424191125,-0.000113818667257794));
#74624=CARTESIAN_POINT('Origin',(-19.0048063345371,0.,0.));
#74625=CARTESIAN_POINT('',(21.870193665463,-4.52947294422145,0.00251866946226621));
#74626=CARTESIAN_POINT('',(22.0180063345369,-4.51707300815329,0.00194757944713214));
#74627=CARTESIAN_POINT('',(-19.0048063345371,-4.52375,5.14627461305311E-12));
#74628=CARTESIAN_POINT('Ctrl Pts',(21.870193665463,-4.52947294422145,0.00251866946226618));
#74629=CARTESIAN_POINT('Ctrl Pts',(21.9060967244749,-4.52042477226542,-1.35327695553929));
#74630=CARTESIAN_POINT('Ctrl Pts',(21.9817551076258,-3.15240519488923,-4.22617295064406));
#74631=CARTESIAN_POINT('Ctrl Pts',(22.0971688149158,1.73710928192197,-5.05982422742967));
#74632=CARTESIAN_POINT('Ctrl Pts',(22.2164347873329,5.19518937246391,-1.27647062404992));
#74633=CARTESIAN_POINT('Ctrl Pts',(22.3357007597501,3.88417622643207,3.67866074976264));
#74634=CARTESIAN_POINT('Ctrl Pts',(22.4549667321673,-0.992442953004545,
5.25684571343457));
#74635=CARTESIAN_POINT('Ctrl Pts',(22.5497977007382,-4.14555697384072,2.6746816967096));
#74636=CARTESIAN_POINT('Ctrl Pts',(22.6048733451701,-4.52095257875769,0.585002942242804));
#74637=CARTESIAN_POINT('Ctrl Pts',(22.620193665463,-4.51785376865908,0.0026509074034578));
#74638=CARTESIAN_POINT('Ctrl Pts',(22.0180063345369,-4.51707300815329,0.00194757944713159));
#74639=CARTESIAN_POINT('Ctrl Pts',(22.0411028251683,-4.51367549994054,-0.87636993032822));
#74640=CARTESIAN_POINT('Ctrl Pts',(22.1039546399389,-3.84198169693815,-3.27131196429832));
#74641=CARTESIAN_POINT('Ctrl Pts',(22.2065617788485,0.0473018698816033,
-5.34949840498282));
#74642=CARTESIAN_POINT('Ctrl Pts',(22.3258277512656,4.5246097295625,-2.85434361052691));
#74643=CARTESIAN_POINT('Ctrl Pts',(22.4450937236827,4.84840476952531,2.26104883685696));
#74644=CARTESIAN_POINT('Ctrl Pts',(22.5643596961,0.72144879027182,5.30083788611039));
#74645=CARTESIAN_POINT('Ctrl Pts',(22.6719972330513,-3.60083421408175,3.65261330297864));
#74646=CARTESIAN_POINT('Ctrl Pts',(22.7398794458636,-4.51218294749925,1.0632531453274));
#74647=CARTESIAN_POINT('Ctrl Pts',(22.7680063345369,-4.52110593686913,-0.00396372416147671));
#74648=CARTESIAN_POINT('Origin',(-19.0048063345371,0.,0.));
#74649=CARTESIAN_POINT('',(21.120193665463,-4.5256415251865,-0.00397048047999635));
#74650=CARTESIAN_POINT('',(21.2680063345369,-4.52825856173475,0.00318332847191585));
#74651=CARTESIAN_POINT('',(-19.0048063345371,-4.52375,5.14627461305311E-12));
#74652=CARTESIAN_POINT('Ctrl Pts',(21.120193665463,-4.5256415251865,-0.0039704804799966));
#74653=CARTESIAN_POINT('Ctrl Pts',(21.1278094555015,-4.52829030282037,-0.292197201058006));
#74654=CARTESIAN_POINT('Ctrl Pts',(21.175180569679,-4.37174733578044,-2.08213483401641));
#74655=CARTESIAN_POINT('Ctrl Pts',(21.2623070079956,-1.98546045804875,-4.96762686192806));
#74656=CARTESIAN_POINT('Ctrl Pts',(21.3815729804128,3.10370713105701,-4.35733541449928));
#74657=CARTESIAN_POINT('Ctrl Pts',(21.50083895283,5.34372570444373,0.252913948788086));
#74658=CARTESIAN_POINT('Ctrl Pts',(21.6201049252471,2.67829727906562,4.63099271806533));
#74659=CARTESIAN_POINT('Ctrl Pts',(21.7393708976643,-2.44576133731702,4.75790093956452));
#74660=CARTESIAN_POINT('Ctrl Pts',(21.8227338110696,-4.45801051457141,1.79375067470569));
#74661=CARTESIAN_POINT('Ctrl Pts',(21.8663414003358,-4.53044377952769,0.147990513631471));
#74662=CARTESIAN_POINT('Ctrl Pts',(21.870193665463,-4.52947294422145,0.00251866946226618));
#74663=CARTESIAN_POINT('Ctrl Pts',(21.2680063345369,-4.52825856173475,0.00318332847191599));
#74664=CARTESIAN_POINT('Ctrl Pts',(21.302570880334,-4.5178259772815,-1.30298465945109));
#74665=CARTESIAN_POINT('Ctrl Pts',(21.3768907502702,-3.23641643652308,-4.12932346936464));
#74666=CARTESIAN_POINT('Ctrl Pts',(21.4909659443455,1.56594352144461,-5.11538772132217));
#74667=CARTESIAN_POINT('Ctrl Pts',(21.6102319167626,5.14931704538713,-1.45048427012945));
#74668=CARTESIAN_POINT('Ctrl Pts',(21.7294978891798,4.00570732897041,3.54593844369029));
#74669=CARTESIAN_POINT('Ctrl Pts',(21.848763861597,-0.81507185340302,5.28725150958398));
#74670=CARTESIAN_POINT('Ctrl Pts',(21.9449333433827,-4.09895685643359,2.77767174480397));
#74671=CARTESIAN_POINT('Ctrl Pts',(22.0013475010293,-4.51952353297804,0.635452703477159));
#74672=CARTESIAN_POINT('Ctrl Pts',(22.0180063345369,-4.51707300815329,0.00194757944713159));
#74673=CARTESIAN_POINT('Origin',(-19.0048063345371,0.,0.));
#74674=CARTESIAN_POINT('',(20.370193665463,-4.51632155205853,-0.000497944189619361));
#74675=CARTESIAN_POINT('',(20.5180063345369,-4.52713413638993,-0.00360679990569157));
#74676=CARTESIAN_POINT('',(-19.0048063345371,-4.52375,5.14627461305311E-12));
#74677=CARTESIAN_POINT('Ctrl Pts',(20.370193665463,-4.51632155205854,-0.000497944189619404));
#74678=CARTESIAN_POINT('Ctrl Pts',(20.3892775106672,-4.51703258266485,-0.726523234129351));
#74679=CARTESIAN_POINT('Ctrl Pts',(20.4481166800104,-4.00866695933645,-2.96405924100118));
#74680=CARTESIAN_POINT('Ctrl Pts',(20.5467111734927,-0.491514830074133,
-5.32708016099266));
#74681=CARTESIAN_POINT('Ctrl Pts',(20.6659771459098,4.21425107232707,-3.29536914005304));
#74682=CARTESIAN_POINT('Ctrl Pts',(20.785243118327,5.05140798950344,1.76143327815877));
#74683=CARTESIAN_POINT('Ctrl Pts',(20.9045090907442,1.25146047202657,5.20127066751764));
#74684=CARTESIAN_POINT('Ctrl Pts',(21.0161592731228,-3.38129990730632,3.95166908847989));
#74685=CARTESIAN_POINT('Ctrl Pts',(21.0880541313624,-4.51446337050284,1.21238034693031));
#74686=CARTESIAN_POINT('Ctrl Pts',(21.120193665463,-4.5256415251865,-0.0039704804799966));
#74687=CARTESIAN_POINT('Ctrl Pts',(20.5180063345369,-4.52713413638994,-0.00360679990569227));
#74688=CARTESIAN_POINT('Ctrl Pts',(20.5242836113606,-4.52920047619369,-0.240973755364537));
#74689=CARTESIAN_POINT('Ctrl Pts',(20.5703162123234,-4.40415625335664,-1.97945418684146));
#74690=CARTESIAN_POINT('Ctrl Pts',(20.6561041374253,-2.1514191011895,-4.89803700505059));
#74691=CARTESIAN_POINT('Ctrl Pts',(20.7753701098425,2.95539580647574,-4.45926073232701));
#74692=CARTESIAN_POINT('Ctrl Pts',(20.8946360822597,5.34920890774529,0.0730391203798664));
#74693=CARTESIAN_POINT('Ctrl Pts',(21.0139020546768,2.83254152524977,4.53829033442592));
#74694=CARTESIAN_POINT('Ctrl Pts',(21.133168027094,-2.28434957613141,4.83747017208749));
#74695=CARTESIAN_POINT('Ctrl Pts',(21.217869453714,-4.42904907663949,1.89619713950708));
#74696=CARTESIAN_POINT('Ctrl Pts',(21.262815556195,-4.52982528949528,0.199338907729788));
#74697=CARTESIAN_POINT('Ctrl Pts',(21.2680063345369,-4.52825856173475,0.00318332847191599));
#74698=CARTESIAN_POINT('Origin',(-19.0048063345371,0.,0.));
#74699=CARTESIAN_POINT('',(19.620193665463,-4.52380831897895,0.00416407692592279));
#74700=CARTESIAN_POINT('',(19.7680063345369,-4.51662655140182,-0.00131840381877635));
#74701=CARTESIAN_POINT('',(-19.0048063345371,-4.52375,5.14627461305311E-12));
#74702=CARTESIAN_POINT('Ctrl Pts',(19.620193665463,-4.52380831897895,0.00416407692592272));
#74703=CARTESIAN_POINT('Ctrl Pts',(19.6507455658328,-4.51311329478492,-1.15330418304886));
#74704=CARTESIAN_POINT('Ctrl Pts',(19.7210527903417,-3.47112927897302,-3.83402298617469));
#74705=CARTESIAN_POINT('Ctrl Pts',(19.8311153389897,1.04298046566866,-5.24705266011862));
#74706=CARTESIAN_POINT('Ctrl Pts',(19.9503813114068,4.97712192131473,-1.9615369612098));
#74707=CARTESIAN_POINT('Ctrl Pts',(20.069647283824,4.34235225730947,3.12463545765959));
#74708=CARTESIAN_POINT('Ctrl Pts',(20.1889132562412,-0.278621045569882,
5.34244702199188));
#74709=CARTESIAN_POINT('Ctrl Pts',(20.2890953834541,-3.94534524041323,3.08584830453267));
#74710=CARTESIAN_POINT('Ctrl Pts',(20.3495221865281,-4.51555136900353,0.785927240390639));
#74711=CARTESIAN_POINT('Ctrl Pts',(20.370193665463,-4.51632155205854,-0.000497944189619404));
#74712=CARTESIAN_POINT('Ctrl Pts',(19.7680063345369,-4.51662655140182,-0.00131840381877607));
#74713=CARTESIAN_POINT('Ctrl Pts',(19.7857516665263,-4.51838370628948,-0.676307662444315));
#74714=CARTESIAN_POINT('Ctrl Pts',(19.8432523226548,-4.0594499556041,-2.86122216995006));
#74715=CARTESIAN_POINT('Ctrl Pts',(19.9405083029223,-0.670408620522066,
-5.30753454377244));
#74716=CARTESIAN_POINT('Ctrl Pts',(20.0597742753395,4.10102977567299,-3.43524750649084));
#74717=CARTESIAN_POINT('Ctrl Pts',(20.1790402477567,5.10779436232139,1.59053682888681));
#74718=CARTESIAN_POINT('Ctrl Pts',(20.2983062201738,1.42569280748336,5.15623609530228));
#74719=CARTESIAN_POINT('Ctrl Pts',(20.4112949157672,-3.30248785860587,4.05005623492106));
#74720=CARTESIAN_POINT('Ctrl Pts',(20.4845282872216,-4.51611390840542,1.26232146629252));
#74721=CARTESIAN_POINT('Ctrl Pts',(20.5180063345369,-4.52713413638994,-0.00360679990569227));
#74722=CARTESIAN_POINT('Origin',(-19.0048063345371,0.,0.));
#74723=CARTESIAN_POINT('',(18.870193665463,-4.53056695484048,-0.00156093939472719));
#74724=CARTESIAN_POINT('',(19.0180063345369,-4.52228481540387,0.00412574957127501));
#74725=CARTESIAN_POINT('',(-19.0048063345371,-4.52375,5.14627461305311E-12));
#74726=CARTESIAN_POINT('Ctrl Pts',(18.870193665463,-4.53056695484048,-0.00156093939472799));
#74727=CARTESIAN_POINT('Ctrl Pts',(18.8724582968594,-4.53094833149528,-0.0870248407490605));
#74728=CARTESIAN_POINT('Ctrl Pts',(18.9144782523949,-4.48997606208692,-1.67242400599934));
#74729=CARTESIAN_POINT('Ctrl Pts',(18.9962535320695,-2.63361203087714,-4.65654996114543));
#74730=CARTESIAN_POINT('Ctrl Pts',(19.1155195044867,2.49143052170795,-4.73414657835247));
#74731=CARTESIAN_POINT('Ctrl Pts',(19.2347854769038,5.32938330746976,-0.465879203105705));
#74732=CARTESIAN_POINT('Ctrl Pts',(19.354051449321,3.27505516474859,4.23005715536775));
#74733=CARTESIAN_POINT('Ctrl Pts',(19.4733174217382,-1.78571650020385,5.04287482005294));
#74734=CARTESIAN_POINT('Ctrl Pts',(19.5620314937855,-4.3307553536982,2.20406739515846));
#74735=CARTESIAN_POINT('Ctrl Pts',(19.6109902416938,-4.52703007732092,0.352838652550256));
#74736=CARTESIAN_POINT('Ctrl Pts',(19.620193665463,-4.52380831897895,0.00416407692592272));
#74737=CARTESIAN_POINT('Ctrl Pts',(19.0180063345369,-4.52228481540387,0.00412574957127487));
#74738=CARTESIAN_POINT('Ctrl Pts',(19.047219721692,-4.51244234885314,-1.10358329220441));
#74739=CARTESIAN_POINT('Ctrl Pts',(19.1161884329861,-3.5438307602279,-3.73412638843344));
#74740=CARTESIAN_POINT('Ctrl Pts',(19.2249124684193,0.865910154356953,-5.27916378381931));
#74741=CARTESIAN_POINT('Ctrl Pts',(19.3441784408365,4.9083313391403,-2.12782849802824));
#74742=CARTESIAN_POINT('Ctrl Pts',(19.4634444132536,4.4449899589576,2.97681623829445));
#74743=CARTESIAN_POINT('Ctrl Pts',(19.5827103856708,-0.0987746801464204,
5.3487955853977));
#74744=CARTESIAN_POINT('Ctrl Pts',(19.6842310260986,-3.88929985589648,3.18831563741184));
#74745=CARTESIAN_POINT('Ctrl Pts',(19.7459963423872,-4.51444710695377,0.835888152378177));
#74746=CARTESIAN_POINT('Ctrl Pts',(19.7680063345369,-4.51662655140182,-0.00131840381877607));
#74747=CARTESIAN_POINT('Origin',(-19.0048063345371,0.,0.));
#74748=CARTESIAN_POINT('',(18.120193665463,-4.51907785273017,-0.00334514387128823));
#74749=CARTESIAN_POINT('',(18.2680063345369,-4.53110217211561,-0.000654014894287402));
#74750=CARTESIAN_POINT('',(-19.0048063345371,-4.52375,5.14627461305311E-12));
#74751=CARTESIAN_POINT('Ctrl Pts',(18.120193665463,-4.51907785273017,-0.00334514387128795));
#74752=CARTESIAN_POINT('Ctrl Pts',(18.1339263520251,-4.52264256910505,-0.524993719082137));
#74753=CARTESIAN_POINT('Ctrl Pts',(18.1874143627263,-4.19793093531997,-2.55248358637957));
#74754=CARTESIAN_POINT('Ctrl Pts',(18.2806576975665,-1.20135384003343,-5.21307191786773));
#74755=CARTESIAN_POINT('Ctrl Pts',(18.3999236699837,3.73433910932905,-3.83067634842202));
#74756=CARTESIAN_POINT('Ctrl Pts',(18.5191896424009,5.24197388553433,1.06821329948656));
#74757=CARTESIAN_POINT('Ctrl Pts',(18.638455614818,1.9375680581184,4.98650176877373));
#74758=CARTESIAN_POINT('Ctrl Pts',(18.7554569558387,-3.04897393187464,4.33978615214932));
#74759=CARTESIAN_POINT('Ctrl Pts',(18.8327029727204,-4.52425331147807,1.41328337976522));
#74760=CARTESIAN_POINT('Ctrl Pts',(18.870193665463,-4.53056695484048,-0.00156093939472799));
#74761=CARTESIAN_POINT('Ctrl Pts',(18.2680063345369,-4.53110217211561,-0.000654014894286977));
#74762=CARTESIAN_POINT('Ctrl Pts',(18.2689324527186,-4.53117262419495,-0.0355933401423199));
#74763=CARTESIAN_POINT('Ctrl Pts',(18.3096138950394,-4.51496105281763,-1.57030029484246));
#74764=CARTESIAN_POINT('Ctrl Pts',(18.3900506614992,-2.78874115530351,-4.5653360687384));
#74765=CARTESIAN_POINT('Ctrl Pts',(18.5093166339163,2.33079188008128,-4.81526529524129));
#74766=CARTESIAN_POINT('Ctrl Pts',(18.6285826063335,5.31069862001794,-0.644864961947463));
#74767=CARTESIAN_POINT('Ctrl Pts',(18.7478485787507,3.41547664867964,4.11751015956628));
#74768=CARTESIAN_POINT('Ctrl Pts',(18.8671145511678,-1.61509331810011,5.10008276654765));
#74769=CARTESIAN_POINT('Ctrl Pts',(18.9571671364299,-4.29399145827576,2.30696570578231));
#74770=CARTESIAN_POINT('Ctrl Pts',(19.0074643975529,-4.52583656589393,0.403853410488209));
#74771=CARTESIAN_POINT('Ctrl Pts',(19.0180063345369,-4.52228481540387,0.00412574957127487));
#74772=CARTESIAN_POINT('Origin',(-19.0048063345371,0.,0.));
#74773=CARTESIAN_POINT('',(17.370193665463,-4.51840654405581,0.00300719303878977));
#74774=CARTESIAN_POINT('',(17.5180063345369,-4.5203228109947,-0.00378289537507237));
#74775=CARTESIAN_POINT('',(-19.0048063345371,-4.52375,5.14627461305311E-12));
#74776=CARTESIAN_POINT('Ctrl Pts',(17.370193665463,-4.51840654405581,0.00300719303878934));
#74777=CARTESIAN_POINT('Ctrl Pts',(17.3953944071908,-4.51258082867698,-0.954623115859167));
#74778=CARTESIAN_POINT('Ctrl Pts',(17.4603504730576,-3.74558763789832,-3.43148573659885));
#74779=CARTESIAN_POINT('Ctrl Pts',(17.5650618630635,0.330015295393627,-5.33951868379825));
#74780=CARTESIAN_POINT('Ctrl Pts',(17.6843278354807,4.66916704311892,-2.61117770235508));
#74781=CARTESIAN_POINT('Ctrl Pts',(17.8035938078979,4.72210487845107,2.51417886927967));
#74782=CARTESIAN_POINT('Ctrl Pts',(17.922859780315,0.440232791824194,5.33156308776582));
#74783=CARTESIAN_POINT('Ctrl Pts',(18.0283930661701,-3.70620368291918,3.49380638893738));
#74784=CARTESIAN_POINT('Ctrl Pts',(18.0941710278861,-4.51232292376063,0.985148386060359));
#74785=CARTESIAN_POINT('Ctrl Pts',(18.120193665463,-4.51907785273017,-0.00334514387128795));
#74786=CARTESIAN_POINT('Ctrl Pts',(17.5180063345369,-4.5203228109947,-0.00378289537507182));
#74787=CARTESIAN_POINT('Ctrl Pts',(17.5304005078843,-4.52402898419069,-0.474260255155535));
#74788=CARTESIAN_POINT('Ctrl Pts',(17.5825500053707,-4.23969939200739,-2.44946365805436));
#74789=CARTESIAN_POINT('Ctrl Pts',(17.6744548269962,-1.37601144972682,-5.1697159633802));
#74790=CARTESIAN_POINT('Ctrl Pts',(17.7937207994134,3.60338472540743,-3.95411041480993));
#74791=CARTESIAN_POINT('Ctrl Pts',(17.9129867718305,5.27493656789836,0.891299532400152));
#74792=CARTESIAN_POINT('Ctrl Pts',(18.0322527442477,2.10418863924757,4.91851205368746));
#74793=CARTESIAN_POINT('Ctrl Pts',(18.1505925984831,-2.95854719837581,4.43440487545489));
#74794=CARTESIAN_POINT('Ctrl Pts',(18.2291771285795,-4.52814833927571,1.46424137628141));
#74795=CARTESIAN_POINT('Ctrl Pts',(18.2680063345369,-4.53110217211561,-0.000654014894286977));
#74796=CARTESIAN_POINT('Origin',(-19.0048063345371,0.,0.));
#74797=CARTESIAN_POINT('',(16.620193665463,-4.53005497334718,0.00207663933256817));
#74798=CARTESIAN_POINT('',(16.7680063345369,-4.51748974129652,0.00236132788964866));
#74799=CARTESIAN_POINT('',(-19.0048063345371,-4.52375,5.14627461305311E-12));
#74800=CARTESIAN_POINT('Ctrl Pts',(16.620193665463,-4.53005497334718,0.00207663933256816));
#74801=CARTESIAN_POINT('Ctrl Pts',(16.6568624623565,-4.52216716072903,-1.3821656394565));
#74802=CARTESIAN_POINT('Ctrl Pts',(16.733286583389,-3.10303436385726,-4.28114918944539));
#74803=CARTESIAN_POINT('Ctrl Pts',(16.8494660285605,1.83415837421399,-5.02545847939519));
#74804=CARTESIAN_POINT('Ctrl Pts',(16.9687320009777,5.21879159998521,-1.17625851994709));
#74805=CARTESIAN_POINT('Ctrl Pts',(17.0879979733949,3.81266515595566,3.75272624612899));
#74806=CARTESIAN_POINT('Ctrl Pts',(17.2072639458121,-1.09342140597902,5.23677376814878));
#74807=CARTESIAN_POINT('Ctrl Pts',(17.3013291765014,-4.17120591260208,2.61574616717072));
#74808=CARTESIAN_POINT('Ctrl Pts',(17.3556390830517,-4.52177116147468,0.556082550935958));
#74809=CARTESIAN_POINT('Ctrl Pts',(17.370193665463,-4.51840654405581,0.00300719303878934));
#74810=CARTESIAN_POINT('Ctrl Pts',(16.7680063345369,-4.51748974129652,0.00236132788964886));
#74811=CARTESIAN_POINT('Ctrl Pts',(16.79186856305,-4.51321097395483,-0.904866519473273));
#74812=CARTESIAN_POINT('Ctrl Pts',(16.855486115702,-3.80763549775125,-3.32969321608406));
#74813=CARTESIAN_POINT('Ctrl Pts',(16.9588589924932,0.150238344599186,-5.34759750650883));
#74814=CARTESIAN_POINT('Ctrl Pts',(17.0781249649104,4.57870057212474,-2.76674388453876));
#74815=CARTESIAN_POINT('Ctrl Pts',(17.1973909373275,4.80399552983808,2.35393236969624));
#74816=CARTESIAN_POINT('Ctrl Pts',(17.3166569097447,0.619306375843183,5.31373976260104));
#74817=CARTESIAN_POINT('Ctrl Pts',(17.4235287088145,-3.6399403872671,3.59495789521742));
#74818=CARTESIAN_POINT('Ctrl Pts',(17.4906451837452,-4.51214113071371,1.03483433420766));
#74819=CARTESIAN_POINT('Ctrl Pts',(17.5180063345369,-4.5203228109947,-0.00378289537507182));
#74820=CARTESIAN_POINT('Origin',(-19.0048063345371,0.,0.));
#74821=CARTESIAN_POINT('',(15.870193665463,-4.5247597024484,-0.0040964371096966));
#74822=CARTESIAN_POINT('',(16.0180063345369,-4.52898076399324,0.00282109434503318));
#74823=CARTESIAN_POINT('',(-19.0048063345371,-4.52375,5.14627461305311E-12));
#74824=CARTESIAN_POINT('Ctrl Pts',(15.870193665463,-4.5247597024484,-0.00409643710969645));
#74825=CARTESIAN_POINT('Ctrl Pts',(15.8785751933831,-4.52770537576116,-0.321462229303889));
#74826=CARTESIAN_POINT('Ctrl Pts',(15.9267120454422,-4.35232613711668,-2.14092699303294));
#74827=CARTESIAN_POINT('Ctrl Pts',(16.0146042216404,-1.88949625357401,-5.00491496207014));
#74828=CARTESIAN_POINT('Ctrl Pts',(16.1338701940576,3.18698452797358,-4.2968010761823));
#74829=CARTESIAN_POINT('Ctrl Pts',(16.2531361664747,5.33786909584254,0.355701258745961));
#74830=CARTESIAN_POINT('Ctrl Pts',(16.3724021388919,2.58868292949964,4.68167604179753));
#74831=CARTESIAN_POINT('Ctrl Pts',(16.4916681113091,-2.53686901787644,4.70995386983385));
#74832=CARTESIAN_POINT('Ctrl Pts',(16.5742652868328,-4.47374742312347,1.73520711701237));
#74833=CARTESIAN_POINT('Ctrl Pts',(16.6171071382174,-4.5307189151892,0.118592638491145));
#74834=CARTESIAN_POINT('Ctrl Pts',(16.620193665463,-4.53005497334718,0.00207663933256816));
#74835=CARTESIAN_POINT('Ctrl Pts',(16.0180063345369,-4.52898076399324,0.0028210943450329));
#74836=CARTESIAN_POINT('Ctrl Pts',(16.0533366182156,-4.51924456004213,-1.33172626091404));
#74837=CARTESIAN_POINT('Ctrl Pts',(16.1284222260334,-3.18871039908969,-4.18484263335493));
#74838=CARTESIAN_POINT('Ctrl Pts',(16.2432631579902,1.66409356894118,-5.08430558145515));
#74839=CARTESIAN_POINT('Ctrl Pts',(16.3625291304074,5.17627646950703,-1.35112270465559));
#74840=CARTESIAN_POINT('Ctrl Pts',(16.4817951028246,3.93672784856066,3.62236725059386));
#74841=CARTESIAN_POINT('Ctrl Pts',(16.6010610752417,-0.916668278371397,
5.27058724614582));
#74842=CARTESIAN_POINT('Ctrl Pts',(16.6964648191458,-4.12589289623653,2.71875914615102));
#74843=CARTESIAN_POINT('Ctrl Pts',(16.7521132389109,-4.52033955301825,0.606607445339812));
#74844=CARTESIAN_POINT('Ctrl Pts',(16.7680063345369,-4.51748974129652,0.00236132788964886));
#74845=CARTESIAN_POINT('Origin',(-19.0048063345371,0.,0.));
#74846=CARTESIAN_POINT('',(15.120193665463,-4.51627216358632,-1.76542077389561E-5));
#74847=CARTESIAN_POINT('',(15.2680063345369,-4.52629070818003,-0.00383690431508932));
#74848=CARTESIAN_POINT('',(-19.0048063345371,-4.52375,5.14627461305311E-12));
#74849=CARTESIAN_POINT('Ctrl Pts',(15.120193665463,-4.51627223874174,-1.76540303067213E-5));
#74850=CARTESIAN_POINT('Ctrl Pts',(15.1400432485488,-4.51629844318397,-0.755195211199893));
#74851=CARTESIAN_POINT('Ctrl Pts',(15.1996481557736,-3.97854876929622,-3.02282933081675));
#74852=CARTESIAN_POINT('Ctrl Pts',(15.2990083871374,-0.388909991241378,
-5.33555235083833));
#74853=CARTESIAN_POINT('Ctrl Pts',(15.4182743595546,4.27688644041953,-3.21366025671349));
#74854=CARTESIAN_POINT('Ctrl Pts',(15.5375403319717,5.01657571134664,1.85831590483193));
#74855=CARTESIAN_POINT('Ctrl Pts',(15.6568063043889,1.15113597147179,5.22439047593186));
#74856=CARTESIAN_POINT('Ctrl Pts',(15.767690748886,-3.42511693477894,3.8950479816348));
#74857=CARTESIAN_POINT('Ctrl Pts',(15.838819869244,-4.51373343669785,1.18386950252823));
#74858=CARTESIAN_POINT('Ctrl Pts',(15.870193665463,-4.5247597024484,-0.00409643710969645));
#74859=CARTESIAN_POINT('Ctrl Pts',(15.2680063345369,-4.52629070818003,-0.0038369043150898));
#74860=CARTESIAN_POINT('Ctrl Pts',(15.2750493492422,-4.52869797060996,-0.270287775271952));
#74861=CARTESIAN_POINT('Ctrl Pts',(15.3218476880866,-4.38585365861661,-2.03818147109467));
#74862=CARTESIAN_POINT('Ctrl Pts',(15.4084013510701,-2.05676334484598,-4.93853168412494));
#74863=CARTESIAN_POINT('Ctrl Pts',(15.5276673234872,3.0406621088803,-4.40156160827348));
#74864=CARTESIAN_POINT('Ctrl Pts',(15.6469332959044,5.34681277770121,0.175965257988861));
#74865=CARTESIAN_POINT('Ctrl Pts',(15.7661992683216,2.74468256834738,4.5919590863615));
#74866=CARTESIAN_POINT('Ctrl Pts',(15.8854652407387,-2.3770183697707,4.79261456008932));
#74867=CARTESIAN_POINT('Ctrl Pts',(15.9694009294772,-4.44584540992525,1.83757239306991));
#74868=CARTESIAN_POINT('Ctrl Pts',(16.0135812940766,-4.53020020216151,0.169970220487411));
#74869=CARTESIAN_POINT('Ctrl Pts',(16.0180063345369,-4.52898076399324,0.0028210943450329));
#74870=CARTESIAN_POINT('Origin',(-19.0048063345371,0.,0.));
#74871=CARTESIAN_POINT('',(14.370193665463,-4.52469469919503,0.00410328708299658));
#74872=CARTESIAN_POINT('',(14.5180063345369,-4.51641831892787,-0.00085334569348311));
#74873=CARTESIAN_POINT('',(-19.0048063345371,-4.52375,5.14627461305311E-12));
#74874=CARTESIAN_POINT('Ctrl Pts',(14.370193665463,-4.52469469919503,0.0041032870829967));
#74875=CARTESIAN_POINT('Ctrl Pts',(14.4015113037144,-4.51368577701503,-1.18177995784863));
#74876=CARTESIAN_POINT('Ctrl Pts',(14.4725842661049,-3.4282942933837,-3.89088640352849));
#74877=CARTESIAN_POINT('Ctrl Pts',(14.5834125526344,1.14376110347399,-5.22600998927515));
#74878=CARTESIAN_POINT('Ctrl Pts',(14.7026785250516,5.01394788167348,-1.86539446490182));
#74879=CARTESIAN_POINT('Ctrl Pts',(14.8219444974688,4.28141795087999,3.20762064460667));
#74880=CARTESIAN_POINT('Ctrl Pts',(14.9412104698859,-0.381378988217642,
5.33609594527402));
#74881=CARTESIAN_POINT('Ctrl Pts',(15.0406268592173,-3.97630906655061,3.02713738035306));
#74882=CARTESIAN_POINT('Ctrl Pts',(15.1002879244097,-4.51624596016253,0.757296433492399));
#74883=CARTESIAN_POINT('Ctrl Pts',(15.120193665463,-4.51627223874174,-1.76540303067213E-5));
#74884=CARTESIAN_POINT('Ctrl Pts',(14.5180063345369,-4.51641831892787,-0.000853345693483179));
#74885=CARTESIAN_POINT('Ctrl Pts',(14.5365174044079,-4.5176016717366,-0.705050397317584));
#74886=CARTESIAN_POINT('Ctrl Pts',(14.594783798418,-4.03068622056879,-2.9200681878472));
#74887=CARTESIAN_POINT('Ctrl Pts',(14.6928055165671,-0.568146787928893,
-5.31945296803855));
#74888=CARTESIAN_POINT('Ctrl Pts',(14.8120714889842,4.16637791607122,-3.35569154009744));
#74889=CARTESIAN_POINT('Ctrl Pts',(14.9313374614014,5.07624035735161,1.68853619629629));
#74890=CARTESIAN_POINT('Ctrl Pts',(15.0506034338186,1.32620268338616,5.18271715361618));
#74891=CARTESIAN_POINT('Ctrl Pts',(15.1628263915304,-3.3479219489578,3.99386544736847));
#74892=CARTESIAN_POINT('Ctrl Pts',(15.2352940251032,-4.51510982658446,1.23373304325699));
#74893=CARTESIAN_POINT('Ctrl Pts',(15.2680063345369,-4.52629070818003,-0.0038369043150898));
#74894=CARTESIAN_POINT('Origin',(-19.0048063345371,0.,0.));
#74895=CARTESIAN_POINT('',(13.620193665463,-4.53009387229811,-0.00204267091282001));
#74896=CARTESIAN_POINT('',(13.7680063345369,-4.52314995435732,0.00416998364050888));
#74897=CARTESIAN_POINT('',(-19.0048063345371,-4.52375,5.14627461305311E-12));
#74898=CARTESIAN_POINT('Ctrl Pts',(13.620193665463,-4.53009387229811,-0.00204267091282042));
#74899=CARTESIAN_POINT('Ctrl Pts',(13.623224034741,-4.53073677915691,-0.116436113594865));
#74900=CARTESIAN_POINT('Ctrl Pts',(13.6660097281581,-4.47487801284166,-1.73091551955723));
#74901=CARTESIAN_POINT('Ctrl Pts',(13.7485507457143,-2.54351413503901,-4.70636863353064));
#74902=CARTESIAN_POINT('Ctrl Pts',(13.8678167181314,2.58207261855057,-4.68532505407631));
#74903=CARTESIAN_POINT('Ctrl Pts',(13.9870826905486,5.33736174127025,-0.363234789975878));
#74904=CARTESIAN_POINT('Ctrl Pts',(14.1063486629658,3.19304587242686,4.29229867628082));
#74905=CARTESIAN_POINT('Ctrl Pts',(14.2256146353829,-1.88243041858965,5.00757681808199));
#74906=CARTESIAN_POINT('Ctrl Pts',(14.3135629695487,-4.35087627651381,2.14524004940141));
#74907=CARTESIAN_POINT('Ctrl Pts',(14.3617559795754,-4.52766075386909,0.323607275213117));
#74908=CARTESIAN_POINT('Ctrl Pts',(14.370193665463,-4.52469469919503,0.0041032870829967));
#74909=CARTESIAN_POINT('Ctrl Pts',(13.7680063345369,-4.52314995435732,0.00416998364050923));
#74910=CARTESIAN_POINT('Ctrl Pts',(13.7979854595736,-4.5127764880711,-1.1320207248508));
#74911=CARTESIAN_POINT('Ctrl Pts',(13.8677199087493,-3.502576575626,-3.79135010209604));
#74912=CARTESIAN_POINT('Ctrl Pts',(13.9772096820641,0.96734152561576,-5.26152269068825));
#74913=CARTESIAN_POINT('Ctrl Pts',(14.0964756544813,4.94837013659463,-2.03297900704013));
#74914=CARTESIAN_POINT('Ctrl Pts',(14.2157416268984,4.38688126484615,3.06180394864691));
#74915=CARTESIAN_POINT('Ctrl Pts',(14.3350075993156,-0.201688098081399,
5.3459042792497));
#74916=CARTESIAN_POINT('Ctrl Pts',(14.4357625018617,-3.92166343592592,3.12972290055515));
#74917=CARTESIAN_POINT('Ctrl Pts',(14.4967620802688,-4.5150602424832,0.807319349011126));
#74918=CARTESIAN_POINT('Ctrl Pts',(14.5180063345369,-4.51641831892787,-0.000853345693483179));
#74919=CARTESIAN_POINT('Origin',(-19.0048063345371,0.,0.));
#74920=CARTESIAN_POINT('',(12.870193665463,-4.51844992363578,-0.00303181240373236));
#74921=CARTESIAN_POINT('',(13.0180063345369,-4.53084488398297,-0.00118107851521998));
#74922=CARTESIAN_POINT('',(-19.0048063345371,-4.52375,5.14627461305311E-12));
#74923=CARTESIAN_POINT('Ctrl Pts',(12.870193665463,-4.51844992363578,-0.00303181240373214));
#74924=CARTESIAN_POINT('Ctrl Pts',(12.8846920899067,-4.52183101233865,-0.553959891712047));
#74925=CARTESIAN_POINT('Ctrl Pts',(12.9389458384895,-4.1730583699505,-2.61142368232673));
#74926=CARTESIAN_POINT('Ctrl Pts',(13.0329549112113,-1.10081151614861,-5.23522529369453));
#74927=CARTESIAN_POINT('Ctrl Pts',(13.1522208836285,3.80736474859714,-3.75810371609987));
#74928=CARTESIAN_POINT('Ctrl Pts',(13.2714868560456,5.22044657695045,1.16889152919789));
#74929=CARTESIAN_POINT('Ctrl Pts',(13.3907528284628,1.84124949551275,5.02286473689053));
#74930=CARTESIAN_POINT('Ctrl Pts',(13.5069884316019,-3.09937585488682,4.28516814783659));
#74931=CARTESIAN_POINT('Ctrl Pts',(13.583468710602,-4.52230250325925,1.38428804770569));
#74932=CARTESIAN_POINT('Ctrl Pts',(13.620193665463,-4.53009387229811,-0.00204267091282042));
#74933=CARTESIAN_POINT('Ctrl Pts',(13.0180063345369,-4.53084488398297,-0.00118107851522056));
#74934=CARTESIAN_POINT('Ctrl Pts',(13.0196981906002,-4.53106719519265,-0.0650188296293057));
#74935=CARTESIAN_POINT('Ctrl Pts',(13.0611453708025,-4.5008850794886,-1.62870450993968));
#74936=CARTESIAN_POINT('Ctrl Pts',(13.1423478751439,-2.70036984388385,-4.61815692219858));
#74937=CARTESIAN_POINT('Ctrl Pts',(13.2616138475611,2.42302476496527,-4.76952006392394));
#74938=CARTESIAN_POINT('Ctrl Pts',(13.3808798199783,5.32212489864176,-0.542546970376561));
#74939=CARTESIAN_POINT('Ctrl Pts',(13.5001457923954,3.33560719654819,4.18247477961839));
#74940=CARTESIAN_POINT('Ctrl Pts',(13.6194117648126,-1.71293973690343,5.06805762689664));
#74941=CARTESIAN_POINT('Ctrl Pts',(13.7086986121931,-4.31527330193496,2.2480898219303));
#74942=CARTESIAN_POINT('Ctrl Pts',(13.7582301354345,-4.52653274393746,0.374682017293747));
#74943=CARTESIAN_POINT('Ctrl Pts',(13.7680063345369,-4.52314995435732,0.00416998364050923));
#74944=CARTESIAN_POINT('Origin',(-19.0048063345371,0.,0.));
#74945=CARTESIAN_POINT('',(12.120193665463,-4.51902956961554,0.00332363250920302));
#74946=CARTESIAN_POINT('',(12.2680063345369,-4.51958929800233,-0.00355049372932015));
#74947=CARTESIAN_POINT('',(-19.0048063345371,-4.52375,5.14627461305311E-12));
#74948=CARTESIAN_POINT('Ctrl Pts',(12.120193665463,-4.51902956961554,0.00332363250920252));
#74949=CARTESIAN_POINT('Ctrl Pts',(12.1461601450724,-4.51233717109749,-0.983063180516055));
#74950=CARTESIAN_POINT('Ctrl Pts',(12.2118819488208,-3.7089260789378,-3.48955300938175));
#74951=CARTESIAN_POINT('Ctrl Pts',(12.3173590767083,0.432707368140066,-5.33217912333988));
#74952=CARTESIAN_POINT('Ctrl Pts',(12.4366250491255,4.71855165499341,-2.52084115901474));
#74953=CARTESIAN_POINT('Ctrl Pts',(12.5558910215426,4.67284781705142,2.6045850242413));
#74954=CARTESIAN_POINT('Ctrl Pts',(12.6751569939598,0.337551180441248,5.33904758083378));
#74955=CARTESIAN_POINT('Ctrl Pts',(12.7799245419332,-3.74292793381757,3.43574863833749));
#74956=CARTESIAN_POINT('Ctrl Pts',(12.8449367657677,-4.51255991685876,0.95670938516384));
#74957=CARTESIAN_POINT('Ctrl Pts',(12.870193665463,-4.51844992363578,-0.00303181240373214));
#74958=CARTESIAN_POINT('Ctrl Pts',(12.2680063345369,-4.51958929800233,-0.00355049372931973));
#74959=CARTESIAN_POINT('Ctrl Pts',(12.2811662457659,-4.52324203005514,-0.503299371711655));
#74960=CARTESIAN_POINT('Ctrl Pts',(12.3340814811339,-4.21606861625357,-2.50839703100191));
#74961=CARTESIAN_POINT('Ctrl Pts',(12.4267520406409,-1.27627112038846,-5.19523846219496));
#74962=CARTESIAN_POINT('Ctrl Pts',(12.5460180130581,3.67880996828069,-3.88403499843739));
#74963=CARTESIAN_POINT('Ctrl Pts',(12.6652839854753,5.25680766681221,0.992644853889018));
#74964=CARTESIAN_POINT('Ctrl Pts',(12.7845499578925,2.00914760921968,4.95809404269169));
#74965=CARTESIAN_POINT('Ctrl Pts',(12.9021240742463,-3.01064165969237,4.38041204226545));
#74966=CARTESIAN_POINT('Ctrl Pts',(12.9799428664611,-4.52584331451383,1.43504405569548));
#74967=CARTESIAN_POINT('Ctrl Pts',(13.0180063345369,-4.53084488398297,-0.00118107851522056));
#74968=CARTESIAN_POINT('Origin',(-19.0048063345371,0.,0.));
#74969=CARTESIAN_POINT('',(11.370193665463,-4.53053606468118,0.00159735848326331));
#74970=CARTESIAN_POINT('',(11.5180063345369,-4.5179861772387,0.00274417767465035));
#74971=CARTESIAN_POINT('',(-19.0048063345371,-4.52375,5.14627461305311E-12));
#74972=CARTESIAN_POINT('Ctrl Pts',(11.370193665463,-4.53053606468118,0.00159735848326391));
#74973=CARTESIAN_POINT('Ctrl Pts',(11.4076282002381,-4.52410350302755,-1.41115327369312));
#74974=CARTESIAN_POINT('Ctrl Pts',(11.4848180591522,-3.05270309746021,-4.3357922845143));
#74975=CARTESIAN_POINT('Ctrl Pts',(11.6017632422053,1.93052816369304,-4.98923149182437));
#74976=CARTESIAN_POINT('Ctrl Pts',(11.7210292146225,5.24046098470274,-1.07561077422649));
#74977=CARTESIAN_POINT('Ctrl Pts',(11.8402951870396,3.73974201866875,3.8254018747875));
#74978=CARTESIAN_POINT('Ctrl Pts',(11.9595611594568,-1.1939948970662,5.21476232014501));
#74979=CARTESIAN_POINT('Ctrl Pts',(12.0528606522646,-4.19613118865777,2.55680616480241));
#74980=CARTESIAN_POINT('Ctrl Pts',(12.1064048209333,-4.52258339917136,0.52711948837973));
#74981=CARTESIAN_POINT('Ctrl Pts',(12.120193665463,-4.51902956961554,0.00332363250920252));
#74982=CARTESIAN_POINT('Ctrl Pts',(11.5180063345369,-4.5179861772387,0.00274417767465021));
#74983=CARTESIAN_POINT('Ctrl Pts',(11.5426343009315,-4.51282034450835,-0.933338999714355));
#74984=CARTESIAN_POINT('Ctrl Pts',(11.6070175914652,-3.77245439838875,-3.38796966408972));
#74985=CARTESIAN_POINT('Ctrl Pts',(11.711156206138,0.25311917672245,-5.34371606040058));
#74986=CARTESIAN_POINT('Ctrl Pts',(11.8304221785551,4.63109563736341,-2.67811946137613));
#74987=CARTESIAN_POINT('Ctrl Pts',(11.9496881509723,4.7578070721057,2.44594409511522));
#74988=CARTESIAN_POINT('Ctrl Pts',(12.0689541233894,0.51693459378251,5.32467363108372));
#74989=CARTESIAN_POINT('Ctrl Pts',(12.1750601845777,-3.67817244537976,3.53714560518498));
#74990=CARTESIAN_POINT('Ctrl Pts',(12.2414109216268,-4.5122073396058,1.00641283581426));
#74991=CARTESIAN_POINT('Ctrl Pts',(12.2680063345369,-4.51958929800233,-0.00355049372931973));
#74992=CARTESIAN_POINT('Origin',(-19.0048063345371,0.,0.));
#74993=CARTESIAN_POINT('',(10.620193665463,-4.52387319312239,-0.00416168075873038));
#74994=CARTESIAN_POINT('',(10.7680063345369,-4.52962834834061,0.00241115988119614));
#74995=CARTESIAN_POINT('',(-19.0048063345371,-4.52375,5.14627461305311E-12));
#74996=CARTESIAN_POINT('Ctrl Pts',(10.620193665463,-4.52387319312239,-0.00416168075873042));
#74997=CARTESIAN_POINT('Ctrl Pts',(10.6293409312647,-4.52707769761145,-0.350695986930693));
#74998=CARTESIAN_POINT('Ctrl Pts',(10.6782435212054,-4.33225334002266,-2.19975205777105));
#74999=CARTESIAN_POINT('Ctrl Pts',(10.7669014352852,-1.79283225123103,-5.04034943121707));
#75000=CARTESIAN_POINT('Ctrl Pts',(10.8861674077023,3.26908158649335,-4.23467536544114));
#75001=CARTESIAN_POINT('Ctrl Pts',(11.0054333801195,5.3300355426419,0.458356830425908));
#75002=CARTESIAN_POINT('Ctrl Pts',(11.1246993525366,2.49810982979476,4.73062544999149));
#75003=CARTESIAN_POINT('Ctrl Pts',(11.2439653249538,-2.62703713820798,4.66026241152792));
#75004=CARTESIAN_POINT('Ctrl Pts',(11.3257967625959,-4.48888884709553,1.6767120036351));
#75005=CARTESIAN_POINT('Ctrl Pts',(11.367872876099,-4.53093485742053,0.0891821691630021));
#75006=CARTESIAN_POINT('Ctrl Pts',(11.370193665463,-4.53053606468118,0.00159735848326391));
#75007=CARTESIAN_POINT('Ctrl Pts',(10.7680063345369,-4.52962834834061,0.00241115988119607));
#75008=CARTESIAN_POINT('Ctrl Pts',(10.8041023560972,-4.5208459704019,-1.36054807436645));
#75009=CARTESIAN_POINT('Ctrl Pts',(10.8799537017966,-3.14005421280247,-4.24005726281787));
#75010=CARTESIAN_POINT('Ctrl Pts',(10.995560371635,1.76162729918915,-5.05134040731361));
#75011=CARTESIAN_POINT('Ctrl Pts',(11.1148263440521,5.20131879681764,-1.2512607344911));
#75012=CARTESIAN_POINT('Ctrl Pts',(11.2340923164693,3.86629035321667,3.69745446982539));
#75013=CARTESIAN_POINT('Ctrl Pts',(11.3533582888864,-1.01792520411819,5.25197095675792));
#75014=CARTESIAN_POINT('Ctrl Pts',(11.447996294909,-4.15208915750858,2.65983099715797));
#75015=CARTESIAN_POINT('Ctrl Pts',(11.5028789767925,-4.52115921225539,0.577719182756343));
#75016=CARTESIAN_POINT('Ctrl Pts',(11.5180063345369,-4.5179861772387,0.00274417767465021));
#75017=CARTESIAN_POINT('Origin',(-19.0048063345371,0.,0.));
#75018=CARTESIAN_POINT('',(9.87019366546302,-4.51631481829542,0.000462863536248687));
#75019=CARTESIAN_POINT('',(10.0180063345369,-4.52542048575924,-0.0040079242928287));
#75020=CARTESIAN_POINT('',(-19.0048063345371,-4.52375,5.14627461305311E-12));
#75021=CARTESIAN_POINT('Ctrl Pts',(9.87019366546302,-4.51631481829542,0.000462863536248928));
#75022=CARTESIAN_POINT('Ctrl Pts',(9.89080898643035,-4.51560089924546,-0.783828764199309));
#75023=CARTESIAN_POINT('Ctrl Pts',(9.95117963153673,-3.94764305999575,-3.08154461394558));
#75024=CARTESIAN_POINT('Ctrl Pts',(10.0513056007822,-0.286161114873556,
-5.34204845411932));
#75025=CARTESIAN_POINT('Ctrl Pts',(10.1705715731993,4.33793781171498,-3.13076115529714));
#75026=CARTESIAN_POINT('Ctrl Pts',(10.2898375456165,4.97988548349452,1.95451028165742));
#75027=CARTESIAN_POINT('Ctrl Pts',(10.4091035180337,1.05038513373988,5.24557536793082));
#75028=CARTESIAN_POINT('Ctrl Pts',(10.5192222246492,-3.46801874972811,3.83820060209342));
#75029=CARTESIAN_POINT('Ctrl Pts',(10.5895856071256,-4.51315046324109,1.15539162065489));
#75030=CARTESIAN_POINT('Ctrl Pts',(10.620193665463,-4.52387319312239,-0.00416168075873042));
#75031=CARTESIAN_POINT('Ctrl Pts',(10.0180063345369,-4.52542048575924,-0.00400792429282804));
#75032=CARTESIAN_POINT('Ctrl Pts',(10.0258150871238,-4.52814717979581,-0.299574684771682));
#75033=CARTESIAN_POINT('Ctrl Pts',(10.0733791638498,-4.3669142806853,-2.09694694671342));
#75034=CARTESIAN_POINT('Ctrl Pts',(10.1606985647148,-1.96134584123722,-4.97719731805657));
#75035=CARTESIAN_POINT('Ctrl Pts',(10.279964537132,3.12480226517166,-4.34223231246161));
#75036=CARTESIAN_POINT('Ctrl Pts',(10.3992305095491,5.34243639065652,0.278826224728918));
#75037=CARTESIAN_POINT('Ctrl Pts',(10.5184964819663,2.65580708494681,4.64392715052188));
#75038=CARTESIAN_POINT('Ctrl Pts',(10.6377624543835,-2.46880680580944,4.74598394512631));
#75039=CARTESIAN_POINT('Ctrl Pts',(10.7209324052403,-4.46203274740751,1.77899348776185));
#75040=CARTESIAN_POINT('Ctrl Pts',(10.7643470319582,-4.53051867854459,0.140583734725522));
#75041=CARTESIAN_POINT('Ctrl Pts',(10.7680063345369,-4.52962834834061,0.00241115988119607));
#75042=CARTESIAN_POINT('Origin',(-19.0048063345371,0.,0.));
#75043=CARTESIAN_POINT('',(9.12019366546302,-4.52557728081363,0.00398177268663652));
#75044=CARTESIAN_POINT('',(9.26800633453692,-4.5163005375385,-0.000377275191646986));
#75045=CARTESIAN_POINT('',(-19.0048063345371,-4.52375,5.14627461305311E-12));
#75046=CARTESIAN_POINT('Ctrl Pts',(9.12019366546302,-4.52557728081363,0.00398177268663646));
#75047=CARTESIAN_POINT('Ctrl Pts',(9.15227704159602,-4.5144046866037,-1.21028811178658));
#75048=CARTESIAN_POINT('Ctrl Pts',(9.22411574186808,-3.38454463484326,-3.94752458958706));
#75049=CARTESIAN_POINT('Ctrl Pts',(9.33570976627918,1.24411813547422,-5.20303180220995));
#75050=CARTESIAN_POINT('Ctrl Pts',(9.45497573869635,5.04891686558556,-1.76856109711541));
#75051=CARTESIAN_POINT('Ctrl Pts',(9.57424171111352,4.21889796935353,3.28941785032073));
#75052=CARTESIAN_POINT('Ctrl Pts',(9.69350768353068,-0.483995682528848,
5.32776858066465));
#75053=CARTESIAN_POINT('Ctrl Pts',(9.79215833498051,-4.00648469947538,2.96837102108853));
#75054=CARTESIAN_POINT('Ctrl Pts',(9.85105366229129,-4.51697764633978,0.728627332389643));
#75055=CARTESIAN_POINT('Ctrl Pts',(9.87019366546302,-4.51631481829542,0.000462863536248928));
#75056=CARTESIAN_POINT('Ctrl Pts',(9.26800633453692,-4.5163005375385,-0.000377275191646917));
#75057=CARTESIAN_POINT('Ctrl Pts',(9.2872831422895,-4.51684456770769,-0.733752169377256));
#75058=CARTESIAN_POINT('Ctrl Pts',(9.34631527418114,-4.0011510798866,-2.97887378297804));
#75059=CARTESIAN_POINT('Ctrl Pts',(9.44510273021184,-0.46567453527804,-5.32940126834165));
#75060=CARTESIAN_POINT('Ctrl Pts',(9.56436870262899,4.23018298784551,-3.27489275261803));
#75061=CARTESIAN_POINT('Ctrl Pts',(9.68363467504617,5.04280630516079,1.78591019383345));
#75062=CARTESIAN_POINT('Ctrl Pts',(9.80290064746333,1.2262213840307,5.20727872973531));
#75063=CARTESIAN_POINT('Ctrl Pts',(9.91435786729357,-3.39242830756635,3.93742298437625));
#75064=CARTESIAN_POINT('Ctrl Pts',(9.98605976298477,-4.51426524359083,1.20519220811969));
#75065=CARTESIAN_POINT('Ctrl Pts',(10.0180063345369,-4.52542048575924,-0.00400792429282804));
#75066=CARTESIAN_POINT('Origin',(-19.0048063345371,0.,0.));
#75067=CARTESIAN_POINT('',(8.37019366546303,-4.52951872580807,-0.00248766312977575));
#75068=CARTESIAN_POINT('',(8.51800633453692,-4.52403144532135,0.00415447988692308));
#75069=CARTESIAN_POINT('',(-19.0048063345371,-4.52375,5.14627461305311E-12));
#75070=CARTESIAN_POINT('Ctrl Pts',(8.37019366546303,-4.52951872580807,-0.00248766312977579));
#75071=CARTESIAN_POINT('Ctrl Pts',(8.37398977262264,-4.53046593894472,-0.14583501537258));
#75072=CARTESIAN_POINT('Ctrl Pts',(8.41754120392131,-4.45918503465124,-1.78945556809376));
#75073=CARTESIAN_POINT('Ctrl Pts',(8.50084795935902,-2.4524742178731,-4.75444424517648));
#75074=CARTESIAN_POINT('Ctrl Pts',(8.6201139317762,2.67175841346331,-4.63476826280582));
#75075=CARTESIAN_POINT('Ctrl Pts',(8.73937990419336,5.34336341837622,-0.260455848433275));
#75076=CARTESIAN_POINT('Ctrl Pts',(8.85864587661052,3.10985399681577,4.35295049228831));
#75077=CARTESIAN_POINT('Ctrl Pts',(8.97791184902769,-1.97844715602509,4.97042419926512));
#75078=CARTESIAN_POINT('Ctrl Pts',(9.06509444531185,-4.37034497134543,2.08644536657521));
#75079=CARTESIAN_POINT('Ctrl Pts',(9.11252171745696,-4.52824893112611,0.294344463332979));
#75080=CARTESIAN_POINT('Ctrl Pts',(9.12019366546302,-4.52557728081363,0.00398177268663646));
#75081=CARTESIAN_POINT('Ctrl Pts',(8.51800633453692,-4.52403144532135,0.00415447988692291));
#75082=CARTESIAN_POINT('Ctrl Pts',(8.54875119745517,-4.51324421933796,-1.1604773474593));
#75083=CARTESIAN_POINT('Ctrl Pts',(8.61925138451249,-3.46042089846282,-3.84837281968134));
#75084=CARTESIAN_POINT('Ctrl Pts',(8.72950689570885,1.06841463020081,-5.2419329287755));
#75085=CARTESIAN_POINT('Ctrl Pts',(8.848772868126,4.98657624511604,-1.93737657760491));
#75086=CARTESIAN_POINT('Ctrl Pts',(8.96803884054318,4.32714783601959,3.14565768274914));
#75087=CARTESIAN_POINT('Ctrl Pts',(9.08730481296034,-0.304526818381393,
5.34103305257461));
#75088=CARTESIAN_POINT('Ctrl Pts',(9.18729397762492,-3.95322283016004,3.07105915382242));
#75089=CARTESIAN_POINT('Ctrl Pts',(9.24752781815045,-4.51572259274196,0.778715922228201));
#75090=CARTESIAN_POINT('Ctrl Pts',(9.26800633453692,-4.5163005375385,-0.000377275191646917));
#75091=CARTESIAN_POINT('Origin',(-19.0048063345371,0.,0.));
#75092=CARTESIAN_POINT('',(7.62019366546304,-4.51789179120342,-0.00267828408389951));
#75093=CARTESIAN_POINT('',(7.76800633453693,-4.53045826813502,-0.00168539955221481));
#75094=CARTESIAN_POINT('',(-19.0048063345371,-4.52375,5.14627461305311E-12));
#75095=CARTESIAN_POINT('Ctrl Pts',(7.62019366546304,-4.51789179120342,-0.00267828408389924));
#75096=CARTESIAN_POINT('Ctrl Pts',(7.63545782778832,-4.52101270627242,-0.582883426044371));
#75097=CARTESIAN_POINT('Ctrl Pts',(7.69047731425265,-4.14746281599376,-2.67035974633324));
#75098=CARTESIAN_POINT('Ctrl Pts',(7.78525212485605,-0.999861493359396,
-5.25543974029968));
#75099=CARTESIAN_POINT('Ctrl Pts',(7.90451809727322,3.87898028412496,-3.68413922445854));
#75100=CARTESIAN_POINT('Ctrl Pts',(8.02378406969037,5.19698581262198,1.26913684574598));
#75101=CARTESIAN_POINT('Ctrl Pts',(8.14305004210754,1.74424900381116,5.05736742609511));
#75102=CARTESIAN_POINT('Ctrl Pts',(8.25851990736508,-3.14881692963313,4.23021577656234));
#75103=CARTESIAN_POINT('Ctrl Pts',(8.33423444848359,-4.52054610167646,1.35539248250157));
#75104=CARTESIAN_POINT('Ctrl Pts',(8.37019366546303,-4.52951872580807,-0.00248766312977579));
#75105=CARTESIAN_POINT('Ctrl Pts',(7.76800633453693,-4.53045826813502,-0.00168539955221455));
#75106=CARTESIAN_POINT('Ctrl Pts',(7.77046392848179,-4.53090073763734,-0.0944373503981022));
#75107=CARTESIAN_POINT('Ctrl Pts',(7.81267684656572,-4.48622713824118,-1.68715899213078));
#75108=CARTESIAN_POINT('Ctrl Pts',(7.89464508878868,-2.6109984177212,-4.66926738519707));
#75109=CARTESIAN_POINT('Ctrl Pts',(8.01391106120587,2.51436025322183,-4.72200838296865));
#75110=CARTESIAN_POINT('Ctrl Pts',(8.13317703362301,5.33158006372075,-0.440028039951035));
#75111=CARTESIAN_POINT('Ctrl Pts',(8.25244300604019,3.25450236181101,4.2458903693777));
#75112=CARTESIAN_POINT('Ctrl Pts',(8.37170897845735,-1.81015174768696,5.0341554705982));
#75113=CARTESIAN_POINT('Ctrl Pts',(8.46023008795626,-4.33588773946907,2.18924030229226));
#75114=CARTESIAN_POINT('Ctrl Pts',(8.50899587331612,-4.5271928801816,0.345475563175432));
#75115=CARTESIAN_POINT('Ctrl Pts',(8.51800633453692,-4.52403144532135,0.00415447988692291));
#75116=CARTESIAN_POINT('Origin',(-19.0048063345371,0.,0.));
#75117=CARTESIAN_POINT('',(6.87019366546302,-4.51971627441788,0.00359563931439616));
#75118=CARTESIAN_POINT('',(7.01800633453693,-4.51891345091625,-0.00327023183485431));
#75119=CARTESIAN_POINT('',(-19.0048063345371,-4.52375,5.14627461305311E-12));
#75120=CARTESIAN_POINT('Ctrl Pts',(6.87019366546302,-4.51971627441788,0.0035956393143962));
#75121=CARTESIAN_POINT('Ctrl Pts',(6.89692588295397,-4.51218785835947,-1.01149097213452));
#75122=CARTESIAN_POINT('Ctrl Pts',(6.96341342458398,-3.67140572599566,-3.54748510584191));
#75123=CARTESIAN_POINT('Ctrl Pts',(7.06965629035308,0.535239182461503,-5.32286472563243));
#75124=CARTESIAN_POINT('Ctrl Pts',(7.18892226277021,4.76618869399877,-2.42957099155845));
#75125=CARTESIAN_POINT('Ctrl Pts',(7.3081882351874,4.62186010975348,2.69402653953035));
#75126=CARTESIAN_POINT('Ctrl Pts',(7.42745420760454,0.234744552882073,5.34455469283609));
#75127=CARTESIAN_POINT('Ctrl Pts',(7.53145601769645,-3.7788013523074,3.37756627327991));
#75128=CARTESIAN_POINT('Ctrl Pts',(7.59570250364927,-4.51288432113509,0.928253771938683));
#75129=CARTESIAN_POINT('Ctrl Pts',(7.62019366546304,-4.51789179120342,-0.00267828408389924));
#75130=CARTESIAN_POINT('Ctrl Pts',(7.01800633453693,-4.51891345091625,-0.00327023183485403));
#75131=CARTESIAN_POINT('Ctrl Pts',(7.03193198364747,-4.52243905823974,-0.53229706378677));
#75132=CARTESIAN_POINT('Ctrl Pts',(7.08561295689706,-4.19173085158956,-2.56733631833659));
#75133=CARTESIAN_POINT('Ctrl Pts',(7.1790492542857,-1.17605810855195,-5.21883684139645));
#75134=CARTESIAN_POINT('Ctrl Pts',(7.29831522670288,3.75287271923664,-3.81252108256694));
#75135=CARTESIAN_POINT('Ctrl Pts',(7.41758119912002,5.23673184321061,1.09362253730968));
#75136=CARTESIAN_POINT('Ctrl Pts',(7.53684717153721,1.91336246699203,4.99583974139622));
#75137=CARTESIAN_POINT('Ctrl Pts',(7.65365555000949,-3.06176589728834,4.32605514967914));
#75138=CARTESIAN_POINT('Ctrl Pts',(7.73070860434274,-4.52374311970654,1.40596668425102));
#75139=CARTESIAN_POINT('Ctrl Pts',(7.76800633453693,-4.53045826813502,-0.00168539955221455));
#75140=CARTESIAN_POINT('Origin',(-19.0048063345371,0.,0.));
#75141=CARTESIAN_POINT('',(6.12019366546304,-4.53090073291162,0.00108832199009027));
#75142=CARTESIAN_POINT('',(6.26800633453693,-4.51855722871701,0.00309087752998455));
#75143=CARTESIAN_POINT('',(-19.0048063345371,-4.52375,5.14627461305311E-12));
#75144=CARTESIAN_POINT('Ctrl Pts',(6.12019366546304,-4.53090073291162,0.00108832199009022));
#75145=CARTESIAN_POINT('Ctrl Pts',(6.15839393811966,-4.52623986823191,-1.4402512020058));
#75146=CARTESIAN_POINT('Ctrl Pts',(6.23634953491534,-3.00140589985132,-4.39008539965263));
#75147=CARTESIAN_POINT('Ctrl Pts',(6.35406045585007,2.02618295863798,-4.95115668182184));
#75148=CARTESIAN_POINT('Ctrl Pts',(6.47332642826723,5.26018950109706,-0.974564663002068));
#75149=CARTESIAN_POINT('Ctrl Pts',(6.59259240068441,3.66543382254001,3.89666071943709));
#75150=CARTESIAN_POINT('Ctrl Pts',(6.71185837310155,-1.29412617765311,5.19081952163018));
#75151=CARTESIAN_POINT('Ctrl Pts',(6.80439212802777,-4.22034197546579,2.49786753720102));
#75152=CARTESIAN_POINT('Ctrl Pts',(6.85717055881492,-4.52338388505486,0.498114330194732));
#75153=CARTESIAN_POINT('Ctrl Pts',(6.87019366546302,-4.51971627441788,0.0035956393143962));
#75154=CARTESIAN_POINT('Ctrl Pts',(6.26800633453693,-4.51855722871701,0.00309087752998441));
#75155=CARTESIAN_POINT('Ctrl Pts',(6.29340003881314,-4.51251100940576,-0.961791319275635));
#75156=CARTESIAN_POINT('Ctrl Pts',(6.35854906722839,-3.73642960746153,-3.44613058706164));
#75157=CARTESIAN_POINT('Ctrl Pts',(6.46345341978273,0.355906263086912,-5.33785550419859));
#75158=CARTESIAN_POINT('Ctrl Pts',(6.58271939219988,4.68177552013038,-2.58850316416958));
#75159=CARTESIAN_POINT('Ctrl Pts',(6.70198536461705,4.70985650278392,2.5370499354549));
#75160=CARTESIAN_POINT('Ctrl Pts',(6.8212513370342,0.41437135872153,5.33363544206753));
#75161=CARTESIAN_POINT('Ctrl Pts',(6.92659166034084,-3.71553874394547,3.47918850561399));
#75162=CARTESIAN_POINT('Ctrl Pts',(6.99217665950841,-4.51237405797874,0.977983212239285));
#75163=CARTESIAN_POINT('Ctrl Pts',(7.01800633453693,-4.51891345091625,-0.00327023183485403));
#75164=CARTESIAN_POINT('Origin',(-19.0048063345371,0.,0.));
#75165=CARTESIAN_POINT('',(5.37019366546304,-4.52299381468164,-0.00416642727447685));
#75166=CARTESIAN_POINT('',(5.51800633453693,-4.53018638553777,0.00195909808577518));
#75167=CARTESIAN_POINT('',(-19.0048063345371,-4.52375,5.14627461305311E-12));
#75168=CARTESIAN_POINT('Ctrl Pts',(5.37019366546304,-4.52299381468164,-0.00416642727447635));
#75169=CARTESIAN_POINT('Ctrl Pts',(5.38010666914628,-4.52641083528021,-0.379896318639062));
#75170=CARTESIAN_POINT('Ctrl Pts',(5.42977499696857,-4.31152030878754,-2.25860656938695));
#75171=CARTESIAN_POINT('Ctrl Pts',(5.51919864892993,-1.69550425170618,-5.07391714578299));
#75172=CARTESIAN_POINT('Ctrl Pts',(5.63846462134707,3.34996790097437,-4.17098129128691));
#75173=CARTESIAN_POINT('Ctrl Pts',(5.75773059376426,5.32022794609337,0.560842644091171));
#75174=CARTESIAN_POINT('Ctrl Pts',(5.8769965661814,2.40661152479762,4.77782281363966));
#75175=CARTESIAN_POINT('Ctrl Pts',(5.99626253859857,-2.71623230345395,4.6088449684815));
#75176=CARTESIAN_POINT('Ctrl Pts',(6.07732823835912,-4.50344228157147,1.61826644506594));
#75177=CARTESIAN_POINT('Ctrl Pts',(6.1186386139806,-4.53109046675448,0.0597621744943599));
#75178=CARTESIAN_POINT('Ctrl Pts',(6.12019366546304,-4.53090073291162,0.00108832199009022));
#75179=CARTESIAN_POINT('Ctrl Pts',(5.51800633453693,-4.53018638553777,0.00195909808577534));
#75180=CARTESIAN_POINT('Ctrl Pts',(5.55486809397881,-4.52263664999813,-1.38946064949308));
#75181=CARTESIAN_POINT('Ctrl Pts',(5.63148517755975,-3.09044188949161,-4.29495111977223));
#75182=CARTESIAN_POINT('Ctrl Pts',(5.74785758527973,1.85850858938807,-5.01650440794967));
#75183=CARTESIAN_POINT('Ctrl Pts',(5.86712355769689,5.22443475258933,-1.1509353447283));
#75184=CARTESIAN_POINT('Ctrl Pts',(5.98638953011406,3.79442093031935,3.77117229192225));
#75185=CARTESIAN_POINT('Ctrl Pts',(6.10565550253122,-1.11880512891234,5.2314095361888));
#75186=CARTESIAN_POINT('Ctrl Pts',(6.19952777067219,-4.17755487009671,2.60089376910365));
#75187=CARTESIAN_POINT('Ctrl Pts',(6.25364471467408,-4.52197671814679,0.548787998841091));
#75188=CARTESIAN_POINT('Ctrl Pts',(6.26800633453693,-4.51855722871701,0.00309087752998441));
#75189=CARTESIAN_POINT('Origin',(-19.0048063345371,0.,0.));
#75190=CARTESIAN_POINT('',(4.62019366546303,-4.5164488708372,0.000937415633822161));
#75191=CARTESIAN_POINT('',(4.76800633453694,-4.52453633389133,-0.00411860558352517));
#75192=CARTESIAN_POINT('',(-19.0048063345371,-4.52375,5.14627461305311E-12));
#75193=CARTESIAN_POINT('Ctrl Pts',(4.62019366546303,-4.5164488708372,0.000937415633822658));
#75194=CARTESIAN_POINT('Ctrl Pts',(4.64157472431194,-4.51494682565391,-0.81242583017847));
#75195=CARTESIAN_POINT('Ctrl Pts',(4.70271110729991,-3.91594066105292,-3.14019634832245));
#75196=CARTESIAN_POINT('Ctrl Pts',(4.80360281442692,-0.183306255264012,
-5.34656606492479));
#75197=CARTESIAN_POINT('Ctrl Pts',(4.9228687868441,4.39738257509714,-3.04670253849241));
#75198=CARTESIAN_POINT('Ctrl Pts',(5.04213475926125,4.94135089461829,2.04998078188042));
#75199=CARTESIAN_POINT('Ctrl Pts',(5.16140073167843,0.949245273126337,5.26481749743252));
#75200=CARTESIAN_POINT('Ctrl Pts',(5.27075370041235,-3.5100128039859,3.78114097945864));
#75201=CARTESIAN_POINT('Ctrl Pts',(5.34035134500722,-4.51270714204787,1.12693895523339));
#75202=CARTESIAN_POINT('Ctrl Pts',(5.37019366546304,-4.52299381468164,-0.00416642727447635));
#75203=CARTESIAN_POINT('Ctrl Pts',(4.76800633453694,-4.52453633389133,-0.00411860558352531));
#75204=CARTESIAN_POINT('Ctrl Pts',(4.77658082500543,-4.52755115931345,-0.328832045921557));
#75205=CARTESIAN_POINT('Ctrl Pts',(4.82491063961298,-4.34732968960615,-2.1557477070525));
#75206=CARTESIAN_POINT('Ctrl Pts',(4.91299577835959,-1.86520192939329,-5.01401958655883));
#75207=CARTESIAN_POINT('Ctrl Pts',(5.03226175077674,3.20778511302202,-4.28129481821586));
#75208=CARTESIAN_POINT('Ctrl Pts',(5.15152772319392,5.33608136745939,0.381583924793045));
#75209=CARTESIAN_POINT('Ctrl Pts',(5.27079369561107,2.56594799116161,4.69417527990397));
#75210=CARTESIAN_POINT('Ctrl Pts',(5.39005966802824,-2.5596808892866,4.69759559741243));
#75211=CARTESIAN_POINT('Ctrl Pts',(5.47246388100352,-4.47761888070279,1.72046201744189));
#75212=CARTESIAN_POINT('Ctrl Pts',(5.51511276983976,-4.53077902269241,0.111182399455819));
#75213=CARTESIAN_POINT('Ctrl Pts',(5.51800633453693,-4.53018638553777,0.00195909808577534));
#75214=CARTESIAN_POINT('Origin',(-19.0048063345371,0.,0.));
#75215=CARTESIAN_POINT('',(3.87019366546304,-4.52644367634736,0.00380007935178159));
#75216=CARTESIAN_POINT('',(4.01800633453694,-4.5162743706215,0.000103656827587228));
#75217=CARTESIAN_POINT('',(-19.0048063345371,-4.52375,5.14627461305311E-12));
#75218=CARTESIAN_POINT('Ctrl Pts',(3.87019366546304,-4.52644367634736,0.00380007935178173));
#75219=CARTESIAN_POINT('Ctrl Pts',(3.90304277947762,-4.51527724527072,-1.2388368090617));
#75220=CARTESIAN_POINT('Ctrl Pts',(3.97564721763126,-3.33987304397421,-4.00392317487317));
#75221=CARTESIAN_POINT('Ctrl Pts',(4.08800697992394,1.34401439322441,-5.17812660917343));
#75222=CARTESIAN_POINT('Ctrl Pts',(4.2072729523411,5.08201592186332,-1.67107272126372));
#75223=CARTESIAN_POINT('Ctrl Pts',(4.32653892475827,4.15481546776415,3.36999678021387));
#75224=CARTESIAN_POINT('Ctrl Pts',(4.44580489717544,-0.586433123165232,
5.31746801230425));
#75225=CARTESIAN_POINT('Ctrl Pts',(4.54368981074369,-4.03588134478939,2.90955762213697));
#75226=CARTESIAN_POINT('Ctrl Pts',(4.60181940017289,-4.51773968514488,0.699918329601546));
#75227=CARTESIAN_POINT('Ctrl Pts',(4.62019366546303,-4.5164488708372,0.000937415633822658));
#75228=CARTESIAN_POINT('Ctrl Pts',(4.01800633453694,-4.5162743706215,0.000103656827587367));
#75229=CARTESIAN_POINT('Ctrl Pts',(4.0380488801711,-4.51611900984864,-0.762414301265039));
#75230=CARTESIAN_POINT('Ctrl Pts',(4.09784674994431,-3.97083530460699,-3.03763086589696));
#75231=CARTESIAN_POINT('Ctrl Pts',(4.1973999438566,-0.363029814411452,-5.33737576020804));
#75232=CARTESIAN_POINT('Ctrl Pts',(4.31666591627375,4.29242136001334,-3.19288106886381));
#75233=CARTESIAN_POINT('Ctrl Pts',(4.43593188869093,5.0075045884559,1.88262275785692));
#75234=CARTESIAN_POINT('Ctrl Pts',(4.55519786110808,1.12578593870418,5.22991172698201));
#75235=CARTESIAN_POINT('Ctrl Pts',(4.66588934305676,-3.43601401505965,3.88074351461167));
#75236=CARTESIAN_POINT('Ctrl Pts',(4.73682550086638,-4.51357302704782,1.17669042452511));
#75237=CARTESIAN_POINT('Ctrl Pts',(4.76800633453694,-4.52453633389133,-0.00411860558352531));
#75238=CARTESIAN_POINT('Origin',(-19.0048063345371,0.,0.));
#75239=CARTESIAN_POINT('',(3.12019366546304,-4.5288567256231,-0.00288945374903278));
#75240=CARTESIAN_POINT('',(3.26800633453694,-4.52491800259618,0.00407838215102319));
#75241=CARTESIAN_POINT('',(-19.0048063345371,-4.52375,5.14627461305311E-12));
#75242=CARTESIAN_POINT('Ctrl Pts',(3.12019366546304,-4.5288567256231,-0.00288945374903232));
#75243=CARTESIAN_POINT('Ctrl Pts',(3.12475551050424,-4.53013724628028,-0.175218534882211));
#75244=CARTESIAN_POINT('Ctrl Pts',(3.16907267968449,-4.44288947225829,-1.84804278754527));
#75245=CARTESIAN_POINT('Ctrl Pts',(3.25314517300379,-2.3605259971177,-4.80075899069673));
#75246=CARTESIAN_POINT('Ctrl Pts',(3.37241114542096,2.76045469022341,-4.58249492886218));
#75247=CARTESIAN_POINT('Ctrl Pts',(3.49167711783813,5.34738611599374,-0.157580443906409));
#75248=CARTESIAN_POINT('Ctrl Pts',(3.61094309025528,3.02551034903617,4.41199014025406));
#75249=CARTESIAN_POINT('Ctrl Pts',(3.73020906267246,-2.07373115154603,4.93143072352554));
#75250=CARTESIAN_POINT('Ctrl Pts',(3.81662592107503,-4.38916996825105,2.02768651061558));
#75251=CARTESIAN_POINT('Ctrl Pts',(3.86328745533856,-4.52879131103003,0.265052527621712));
#75252=CARTESIAN_POINT('Ctrl Pts',(3.87019366546304,-4.52644367634736,0.00380007935178173));
#75253=CARTESIAN_POINT('Ctrl Pts',(3.26800633453694,-4.52491800259618,0.00407838215102287));
#75254=CARTESIAN_POINT('Ctrl Pts',(3.29951693533677,-4.51385291460914,-1.1889605374125));
#75255=CARTESIAN_POINT('Ctrl Pts',(3.37078286027565,-3.41735611451173,-3.90518081470287));
#75256=CARTESIAN_POINT('Ctrl Pts',(3.48180410935361,1.16909203446164,-5.22040175338702));
#75257=CARTESIAN_POINT('Ctrl Pts',(3.60107008177076,5.0229355146086,-1.84105661724222));
#75258=CARTESIAN_POINT('Ctrl Pts',(3.72033605418794,4.2658117954781,3.2283463843534));
#75259=CARTESIAN_POINT('Ctrl Pts',(3.83960202660509,-0.407252753478724,
5.33418370949033));
#75260=CARTESIAN_POINT('Ctrl Pts',(3.9388254533881,-3.98398716984629,3.01233344768666));
#75261=CARTESIAN_POINT('Ctrl Pts',(3.99829355603205,-4.51642717518832,0.750075635849043));
#75262=CARTESIAN_POINT('Ctrl Pts',(4.01800633453694,-4.5162743706215,0.000103656827587367));
#75263=CARTESIAN_POINT('Origin',(-19.0048063345371,0.,0.));
#75264=CARTESIAN_POINT('',(2.37019366546305,-4.5174092464024,-0.00228951928982141));
#75265=CARTESIAN_POINT('',(2.51800633453694,-4.52995801530325,-0.00215854265389115));
#75266=CARTESIAN_POINT('',(-19.0048063345371,-4.52375,5.14627461305311E-12));
#75267=CARTESIAN_POINT('Ctrl Pts',(2.37019366546305,-4.5174092464024,-0.00228951928982118));
#75268=CARTESIAN_POINT('Ctrl Pts',(2.38622356566991,-4.52019326613613,-0.611764002830002));
#75269=CARTESIAN_POINT('Ctrl Pts',(2.44200879001584,-4.12113506616917,-2.72928560151133));
#75270=CARTESIAN_POINT('Ctrl Pts',(2.5375493385008,-0.898541159731936,-5.27370777101761));
#75271=CARTESIAN_POINT('Ctrl Pts',(2.65681531091797,3.94915919222963,-3.60881026714515));
#75272=CARTESIAN_POINT('Ctrl Pts',(2.77608128333514,5.17160028152781,1.36891212206108));
#75273=CARTESIAN_POINT('Ctrl Pts',(2.8953472557523,1.64660250832305,5.0899970578978));
#75274=CARTESIAN_POINT('Ctrl Pts',(3.01005138312827,-3.19730291715651,4.1749455591871));
#75275=CARTESIAN_POINT('Ctrl Pts',(3.08500018636519,-4.51897783307502,1.3265857607853));
#75276=CARTESIAN_POINT('Ctrl Pts',(3.12019366546304,-4.5288567256231,-0.00288945374903232));
#75277=CARTESIAN_POINT('Ctrl Pts',(2.51800633453694,-4.52995801530325,-0.00215854265389051));
#75278=CARTESIAN_POINT('Ctrl Pts',(2.52122966636339,-4.53067412723567,-0.123845793639021));
#75279=CARTESIAN_POINT('Ctrl Pts',(2.56420832232889,-4.47097988144249,-1.745662850511));
#75280=CARTESIAN_POINT('Ctrl Pts',(2.64694230243346,-2.52065997660762,-4.71864852835388));
#75281=CARTESIAN_POINT('Ctrl Pts',(2.76620827485062,2.60476451764482,-4.67274784890289));
#75282=CARTESIAN_POINT('Ctrl Pts',(2.88547424726778,5.33906061341968,-0.337346139800582));
#75283=CARTESIAN_POINT('Ctrl Pts',(3.00474021968495,3.17219218262773,4.3077334421112));
#75284=CARTESIAN_POINT('Ctrl Pts',(3.1240061921021,-1.90669334680315,4.99838885372723));
#75285=CARTESIAN_POINT('Ctrl Pts',(3.21176156371945,-4.35584349366905,2.13042087106249));
#75286=CARTESIAN_POINT('Ctrl Pts',(3.25976161119772,-4.52781317396269,0.316236055284816));
#75287=CARTESIAN_POINT('Ctrl Pts',(3.26800633453694,-4.52491800259618,0.00407838215102287));
#75288=CARTESIAN_POINT('Origin',(-19.0048063345371,0.,0.));
#75289=CARTESIAN_POINT('',(1.62019366546304,-4.52045926477682,0.00381908414570068));
#75290=CARTESIAN_POINT('',(1.76800633453694,-4.51830251797945,-0.00294632473948842));
#75291=CARTESIAN_POINT('',(-19.0048063345371,-4.52375,5.14627461305311E-12));
#75292=CARTESIAN_POINT('Ctrl Pts',(1.62019366546304,-4.52045926477682,0.00381908414570031));
#75293=CARTESIAN_POINT('Ctrl Pts',(1.64769162083558,-4.51214039746521,-1.03991157870731));
#75294=CARTESIAN_POINT('Ctrl Pts',(1.71494490034717,-3.63301811037992,-3.6052702635876));
#75295=CARTESIAN_POINT('Ctrl Pts',(1.82195350399781,0.637572764456073,-5.31157894037619));
#75296=CARTESIAN_POINT('Ctrl Pts',(1.94121947641498,4.81206051717935,-2.33740100300047));
#75297=CARTESIAN_POINT('Ctrl Pts',(2.06048544883214,4.56916064047356,2.78247028939603));
#75298=CARTESIAN_POINT('Ctrl Pts',(2.17975142124932,0.13185098482894,5.34808238414702));
#75299=CARTESIAN_POINT('Ctrl Pts',(2.2829874934596,-3.81383264233026,3.31927032643957));
#75300=CARTESIAN_POINT('Ctrl Pts',(2.34646824153085,-4.51328869371237,0.899777262863328));
#75301=CARTESIAN_POINT('Ctrl Pts',(2.37019366546305,-4.5174092464024,-0.00228951928982118));
#75302=CARTESIAN_POINT('Ctrl Pts',(1.76800633453694,-4.51830251797944,-0.00294632473948821));
#75303=CARTESIAN_POINT('Ctrl Pts',(1.78269772152906,-4.52162528364921,-0.561252537622042));
#75304=CARTESIAN_POINT('Ctrl Pts',(1.83714443266024,-4.1666769618709,-2.62627596164084));
#75305=CARTESIAN_POINT('Ctrl Pts',(1.93134646793046,-1.07540952932231,-5.24050236103854));
#75306=CARTESIAN_POINT('Ctrl Pts',(2.05061244034763,3.82554554823664,-3.73959515324518));
#75307=CARTESIAN_POINT('Ctrl Pts',(2.16987841276479,5.21471653241851,1.19419518435166));
#75308=CARTESIAN_POINT('Ctrl Pts',(2.28914438518196,1.81686868775421,5.03173517022369));
#75309=CARTESIAN_POINT('Ctrl Pts',(2.40518702577268,-3.11192516407456,4.27135130982762));
#75310=CARTESIAN_POINT('Ctrl Pts',(2.48147434222434,-4.52184188050285,1.37699754703399));
#75311=CARTESIAN_POINT('Ctrl Pts',(2.51800633453694,-4.52995801530325,-0.00215854265389051));
#75312=CARTESIAN_POINT('Origin',(-19.0048063345371,0.,0.));
#75313=CARTESIAN_POINT('',(0.870193665463051,-4.53113324750611,0.000558172709172654));
#75314=CARTESIAN_POINT('',(1.01800633453695,-4.51919695317837,0.00339653540470913));
#75315=CARTESIAN_POINT('',(-19.0048063345371,-4.52375,5.14627461305311E-12));
#75316=CARTESIAN_POINT('Ctrl Pts',(0.870193665463051,-4.53113324750611,
0.000558172709172731));
#75317=CARTESIAN_POINT('Ctrl Pts',(0.909159676001256,-4.52858208666899,
-1.46947121982517));
#75318=CARTESIAN_POINT('Ctrl Pts',(0.987881010678515,-2.94913757193914,
-4.44401136316868));
#75319=CARTESIAN_POINT('Ctrl Pts',(1.10635766949483,2.12108733213468,-4.91124815085553));
#75320=CARTESIAN_POINT('Ctrl Pts',(1.22562364191199,5.27796984247255,-0.873157609927544));
#75321=CARTESIAN_POINT('Ctrl Pts',(1.34488961432916,3.58976808851186,3.96647638849978));
#75322=CARTESIAN_POINT('Ctrl Pts',(1.46415558674632,-1.39377816290472,5.16495424011036));
#75323=CARTESIAN_POINT('Ctrl Pts',(1.55592360379095,-4.24384740014909,2.43893578023149));
#75324=CARTESIAN_POINT('Ctrl Pts',(1.60793629669652,-4.52416744682079,0.469067916438565));
#75325=CARTESIAN_POINT('Ctrl Pts',(1.62019366546304,-4.52045926477682,0.00381908414570031));
#75326=CARTESIAN_POINT('Ctrl Pts',(1.01800633453695,-4.51919695317837,0.00339653540470948));
#75327=CARTESIAN_POINT('Ctrl Pts',(1.04416577669474,-4.51229041994084,-0.990227835244301));
#75328=CARTESIAN_POINT('Ctrl Pts',(1.11008054299158,-3.69955244106376,-3.50416488459642));
#75329=CARTESIAN_POINT('Ctrl Pts',(1.21575063342748,0.458561535247667,-5.33001800843103));
#75330=CARTESIAN_POINT('Ctrl Pts',(1.33501660584464,4.73072145051602,-2.49792818340231));
#75331=CARTESIAN_POINT('Ctrl Pts',(1.4542825782618,4.66016158094803,2.62721614856175));
#75332=CARTESIAN_POINT('Ctrl Pts',(1.57354855067898,0.311654656198974,5.34062187643698));
#75333=CARTESIAN_POINT('Ctrl Pts',(1.67812313610401,-3.75204777525101,3.42109829131755));
#75334=CARTESIAN_POINT('Ctrl Pts',(1.74294239739001,-4.51263378228107,0.94954045107943));
#75335=CARTESIAN_POINT('Ctrl Pts',(1.76800633453694,-4.51830251797944,-0.00294632473948821));
#75336=CARTESIAN_POINT('Origin',(-19.0048063345371,0.,0.));
#75337=CARTESIAN_POINT('',(0.120193665463054,-4.5221327339856,-0.00411166771258635));
#75338=CARTESIAN_POINT('',(0.268006334536952,-4.53063960879454,0.00147156798560651));
#75339=CARTESIAN_POINT('',(-19.0048063345371,-4.52375,5.14627461305311E-12));
#75340=CARTESIAN_POINT('Ctrl Pts',(0.120193665463054,-4.5221327339856,-0.00411166771258617));
#75341=CARTESIAN_POINT('Ctrl Pts',(0.130872407027874,-4.52570863968184,
-0.409061250785844));
#75342=CARTESIAN_POINT('Ctrl Pts',(0.181306472731748,-4.29011830250525,
-2.31748674548857));
#75343=CARTESIAN_POINT('Ctrl Pts',(0.271495862574679,-1.59754830160526,
-5.10560567355749));
#75344=CARTESIAN_POINT('Ctrl Pts',(0.390761834991842,3.42961351418844,-4.10574244359289));
#75345=CARTESIAN_POINT('Ctrl Pts',(0.510027807409007,5.30844993855932,0.663120742876867));
#75346=CARTESIAN_POINT('Ctrl Pts',(0.629293779826171,2.3142219020159,4.82325065262569));
#75347=CARTESIAN_POINT('Ctrl Pts',(0.748559752243337,-2.80442147910245,
4.55572058376859));
#75348=CARTESIAN_POINT('Ctrl Pts',(0.828859714122298,-4.51741504144067,
1.5598712850993));
#75349=CARTESIAN_POINT('Ctrl Pts',(0.869404351862201,-4.53118492500449,
0.0303357705989649));
#75350=CARTESIAN_POINT('Ctrl Pts',(0.870193665463051,-4.53113324750611,
0.000558172709172731));
#75351=CARTESIAN_POINT('Ctrl Pts',(0.268006334536952,-4.53063960879454,
0.00147156798560636));
#75352=CARTESIAN_POINT('Ctrl Pts',(0.30563383186041,-4.52462283428668,-1.41847499082472));
#75353=CARTESIAN_POINT('Ctrl Pts',(0.383016653322921,-3.03986771850672,
-4.34950762223985));
#75354=CARTESIAN_POINT('Ctrl Pts',(0.500154798924492,1.95470155837633,-4.9798104852985));
#75355=CARTESIAN_POINT('Ctrl Pts',(0.619420771341654,5.24561577554724,-1.05018369209291));
#75356=CARTESIAN_POINT('Ctrl Pts',(0.738686743758821,3.72114619758183,3.84349341459433));
#75357=CARTESIAN_POINT('Ctrl Pts',(0.857952716175984,-1.21927069064937,
5.20891059961017));
#75358=CARTESIAN_POINT('Ctrl Pts',(0.951059246435361,-4.20229923544821,
2.54195357514844));
#75359=CARTESIAN_POINT('Ctrl Pts',(1.00441045255568,-4.52278649496717,0.51981426310584));
#75360=CARTESIAN_POINT('Ctrl Pts',(1.01800633453695,-4.51919695317837,0.00339653540470948));
#75361=CARTESIAN_POINT('Origin',(-19.0048063345371,0.,0.));
#75362=CARTESIAN_POINT('',(-0.629806334536947,-4.51667307150718,0.00139986576683541));
#75363=CARTESIAN_POINT('',(-0.481993665463047,-4.52365053271834,-0.00416855255043758));
#75364=CARTESIAN_POINT('',(-19.0048063345371,-4.52375,5.14627461305311E-12));
#75365=CARTESIAN_POINT('Ctrl Pts',(-0.629806334536947,-4.51667307150718,
0.00139986576683564));
#75366=CARTESIAN_POINT('Ctrl Pts',(-0.607659537806456,-4.51434322716492,
-0.840988711232888));
#75367=CARTESIAN_POINT('Ctrl Pts',(-0.545757416936911,-3.88343245072244,
-3.19877541626441));
#75368=CARTESIAN_POINT('Ctrl Pts',(-0.444099971928309,-0.0803835059582494,
-5.3491035101028));
#75369=CARTESIAN_POINT('Ctrl Pts',(-0.324833999511145,4.45519871447649,
-2.9615155384281));
#75370=CARTESIAN_POINT('Ctrl Pts',(-0.205568027093979,4.90098621647057,
2.14469204684251));
#75371=CARTESIAN_POINT('Ctrl Pts',(-0.0863020546768169,0.847753848005954,
5.28210973788082));
#75372=CARTESIAN_POINT('Ctrl Pts',(0.0222851761755296,-3.55110674608297,
3.72388277406811));
#75373=CARTESIAN_POINT('Ctrl Pts',(0.0911170828888195,-4.51239608883662,
1.09850420880814));
#75374=CARTESIAN_POINT('Ctrl Pts',(0.120193665463054,-4.5221327339856,-0.00411166771258617));
#75375=CARTESIAN_POINT('Ctrl Pts',(-0.481993665463047,-4.52365053271834,
-0.00416855255043813));
#75376=CARTESIAN_POINT('Ctrl Pts',(-0.472653437112973,-4.52691325946138,
-0.358057576997311));
#75377=CARTESIAN_POINT('Ctrl Pts',(-0.423557884623844,-4.32709133434675,
-2.21458053169529));
#75378=CARTESIAN_POINT('Ctrl Pts',(-0.33470700799566,-1.76836721737897,
-5.04898485205759));
#75379=CARTESIAN_POINT('Ctrl Pts',(-0.215441035578497,3.2895799187264,-4.21877169447693));
#75380=CARTESIAN_POINT('Ctrl Pts',(-0.0961750631613321,5.32775006176976,
0.484200300619735));
#75381=CARTESIAN_POINT('Ctrl Pts',(0.0230909092558323,2.4751385673978,4.74268486450319));
#75382=CARTESIAN_POINT('Ctrl Pts',(0.142356881672996,-2.64960696388247,
4.64746743815955));
#75383=CARTESIAN_POINT('Ctrl Pts',(0.223995356766704,-4.49261143470523,
1.66197929681203));
#75384=CARTESIAN_POINT('Ctrl Pts',(0.265878507721356,-4.53097985608846,
0.0817692380266874));
#75385=CARTESIAN_POINT('Ctrl Pts',(0.268006334536952,-4.53063960879454,
0.00147156798560636));
#75386=CARTESIAN_POINT('Origin',(-19.0048063345371,0.,0.));
#75387=CARTESIAN_POINT('',(-1.37980633453694,-4.52728092082441,0.00355961958845701));
#75388=CARTESIAN_POINT('',(-1.23199366546305,-4.51634007617231,0.000583253576266762));
#75389=CARTESIAN_POINT('',(-19.0048063345371,-4.52375,5.14627461305311E-12));
#75390=CARTESIAN_POINT('Ctrl Pts',(-1.37980633453694,-4.52728092082441,
0.00355961958845723));
#75391=CARTESIAN_POINT('Ctrl Pts',(-1.34619148264078,-4.51631056435734,
-1.26743466713941));
#75392=CARTESIAN_POINT('Ctrl Pts',(-1.27282130660557,-3.29427248004508,
-4.06006742591324));
#75393=CARTESIAN_POINT('Ctrl Pts',(-1.1596958064313,1.4434128789333,-5.15130363410601));
#75394=CARTESIAN_POINT('Ctrl Pts',(-1.04042983401413,5.1132327918697,-1.57296544334973));
#75395=CARTESIAN_POINT('Ctrl Pts',(-0.921163861596969,4.08919417984387,
3.4493275909016));
#75396=CARTESIAN_POINT('Ctrl Pts',(-0.801897889179802,-0.688653371177603,
5.30519805513329));
#75397=CARTESIAN_POINT('Ctrl Pts',(-0.704778713493129,-4.06450823554763,
2.8507052065737));
#75398=CARTESIAN_POINT('Ctrl Pts',(-0.64741486194551,-4.51852548964501,
0.671168163515238));
#75399=CARTESIAN_POINT('Ctrl Pts',(-0.629806334536947,-4.51667307150718,
0.00139986576683564));
#75400=CARTESIAN_POINT('Ctrl Pts',(-1.23199366546305,-4.51634007617231,
0.00058325357626697));
#75401=CARTESIAN_POINT('Ctrl Pts',(-1.2111853819473,-4.51543176696114,-0.791038463333831));
#75402=CARTESIAN_POINT('Ctrl Pts',(-1.1506217742925,-3.93972969518399,-3.09633097448578));
#75403=CARTESIAN_POINT('Ctrl Pts',(-1.05030284249865,-0.260250641047462,
-5.34337349018783));
#75404=CARTESIAN_POINT('Ctrl Pts',(-0.931036870081484,4.35306998183813,
-3.10968686285734));
#75405=CARTESIAN_POINT('Ctrl Pts',(-0.811770897664319,4.97034828165621,
1.97863806969469));
#75406=CARTESIAN_POINT('Ctrl Pts',(-0.692504925247154,1.02493354489289,
5.25060776295097));
#75407=CARTESIAN_POINT('Ctrl Pts',(-0.582579181180064,-3.47868636868056,
3.82384134221039));
#75408=CARTESIAN_POINT('Ctrl Pts',(-0.512408761252028,-4.51302593739761,
1.14821960904481));
#75409=CARTESIAN_POINT('Ctrl Pts',(-0.481993665463047,-4.52365053271834,
-0.00416855255043813));
#75410=CARTESIAN_POINT('Origin',(-19.0048063345371,0.,0.));
#75411=CARTESIAN_POINT('',(-2.12980633453694,-4.5281227353363,-0.00324265984058113));
#75412=CARTESIAN_POINT('',(-1.98199366546304,-4.5257976962895,0.00394161820304176));
#75413=CARTESIAN_POINT('',(-19.0048063345371,-4.52375,5.14627461305311E-12));
#75414=CARTESIAN_POINT('Ctrl Pts',(-2.12980633453694,-4.5281227353363,-0.00324265984058134));
#75415=CARTESIAN_POINT('Ctrl Pts',(-2.12447875161416,-4.52975245353138,
-0.204583738014264));
#75416=CARTESIAN_POINT('Ctrl Pts',(-2.07939584455233,-4.42598350509595,
-1.90667553345163));
#75417=CARTESIAN_POINT('Ctrl Pts',(-1.99455761335145,-2.26770352691226,
-4.84529571686329));
#75418=CARTESIAN_POINT('Ctrl Pts',(-1.87529164093429,2.84812859908841,-4.52852441230905));
#75419=CARTESIAN_POINT('Ctrl Pts',(-1.75602566851712,5.3494283442679,-0.0546466775498073));
#75420=CARTESIAN_POINT('Ctrl Pts',(-1.63675969609995,2.94004616678162,4.46939575412793));
#75421=CARTESIAN_POINT('Ctrl Pts',(-1.51749372368279,-2.1682471155684,4.89061083257026));
#75422=CARTESIAN_POINT('Ctrl Pts',(-1.43184260316178,-4.40735967461942,
1.96896633272643));
#75423=CARTESIAN_POINT('Ctrl Pts',(-1.38594680677984,-4.52928489125952,
0.235733932378456));
#75424=CARTESIAN_POINT('Ctrl Pts',(-1.37980633453694,-4.52728092082441,
0.00355961958845723));
#75425=CARTESIAN_POINT('Ctrl Pts',(-1.98199366546304,-4.5257976962895,0.00394161820304197));
#75426=CARTESIAN_POINT('Ctrl Pts',(-1.94971732678163,-4.51460986650304,
-1.21747812123507));
#75427=CARTESIAN_POINT('Ctrl Pts',(-1.87768566396116,-3.37337480828373,
-3.96175999185013));
#75428=CARTESIAN_POINT('Ctrl Pts',(-1.76589867700163,1.26933645129948,-5.19693713885497));
#75429=CARTESIAN_POINT('Ctrl Pts',(-1.64663270458447,5.05743447897554,-1.74405479921852));
#75430=CARTESIAN_POINT('Ctrl Pts',(-1.52736673216731,4.20289585976879,3.30983942869535));
#75431=CARTESIAN_POINT('Ctrl Pts',(-1.40810075975014,-0.509827857576372,
5.32535878673416));
#75432=CARTESIAN_POINT('Ctrl Pts',(-1.30964307084872,-4.01396563289227,
2.95355445726466));
#75433=CARTESIAN_POINT('Ctrl Pts',(-1.25094070608636,-4.51716713965928,
0.721396617025564));
#75434=CARTESIAN_POINT('Ctrl Pts',(-1.23199366546305,-4.51634007617231,
0.00058325357626697));
#75435=CARTESIAN_POINT('Origin',(-19.0048063345371,0.,0.));
#75436=CARTESIAN_POINT('',(-2.87980633453694,-4.51700722203196,-0.00187082749320296));
#75437=CARTESIAN_POINT('',(-2.73199366546304,-4.52935956130001,-0.002593214221287));
#75438=CARTESIAN_POINT('',(-19.0048063345371,-4.52375,5.14627461305311E-12));
#75439=CARTESIAN_POINT('Ctrl Pts',(-2.87980633453694,-4.51700722203196,
-0.00187082749320257));
#75440=CARTESIAN_POINT('Ctrl Pts',(-2.86301069644849,-4.51937852208916,
-0.640601591406374));
#75441=CARTESIAN_POINT('Ctrl Pts',(-2.80645973422099,-4.09406588665098,
-2.7881947122476));
#75442=CARTESIAN_POINT('Ctrl Pts',(-2.71015344785444,-0.796888040481462,
-5.29002262006144));
#75443=CARTESIAN_POINT('Ctrl Pts',(-2.59088747543727,4.01787548130092,-3.53214474315326));
#75444=CARTESIAN_POINT('Ctrl Pts',(-2.4716215030201,5.1442993855074,1.46818040515877));
#75445=CARTESIAN_POINT('Ctrl Pts',(-2.35235553060294,1.54834617361307,5.12074154751847));
#75446=CARTESIAN_POINT('Ctrl Pts',(-2.23841714110855,-3.24483985403934,
4.11937367175704));
#75447=CARTESIAN_POINT('Ctrl Pts',(-2.16423407575322,-4.51759122093492,
1.2978574142544));
#75448=CARTESIAN_POINT('Ctrl Pts',(-2.12980633453694,-4.5281227353363,-0.00324265984058134));
#75449=CARTESIAN_POINT('Ctrl Pts',(-2.73199366546304,-4.52935956130001,
-0.00259321422128662));
#75450=CARTESIAN_POINT('Ctrl Pts',(-2.72800459575501,-4.53038856066062,
-0.153241100583692));
#75451=CARTESIAN_POINT('Ctrl Pts',(-2.68426020190793,-4.4551357826128,-1.8042149261768));
#75452=CARTESIAN_POINT('Ctrl Pts',(-2.60076048392179,-2.42938797848125,
-4.76628206276323));
#75453=CARTESIAN_POINT('Ctrl Pts',(-2.48149451150462,2.69420407591751,-4.62175670596335));
#75454=CARTESIAN_POINT('Ctrl Pts',(-2.36222853908746,5.34456377722621,-0.234539299413323));
#75455=CARTESIAN_POINT('Ctrl Pts',(-2.2429625666703,3.0887071435723,4.36798109348626));
#75456=CARTESIAN_POINT('Ctrl Pts',(-2.12369659425313,-2.00252877889888,
4.96077102288439));
#75457=CARTESIAN_POINT('Ctrl Pts',(-2.03670696051738,-4.37514918048342,
2.07163492985408));
#75458=CARTESIAN_POINT('Ctrl Pts',(-1.98947265092069,-4.52839010979406,
0.286965679856997));
#75459=CARTESIAN_POINT('Ctrl Pts',(-1.98199366546304,-4.5257976962895,0.00394161820304197));
#75460=CARTESIAN_POINT('Origin',(-19.0048063345371,0.,0.));
#75461=CARTESIAN_POINT('',(-3.62980633453693,-4.52125034636371,0.00399034990006141));
#75462=CARTESIAN_POINT('',(-3.48199366546304,-4.51776292098496,-0.00258343477365697));
#75463=CARTESIAN_POINT('',(-19.0048063345371,-4.52375,5.14627461305311E-12));
#75464=CARTESIAN_POINT('Ctrl Pts',(-3.62980633453693,-4.52125034636371,
0.00399034990006115));
#75465=CARTESIAN_POINT('Ctrl Pts',(-3.60154264128282,-4.51220230515001,
-1.06833051476153));
#75466=CARTESIAN_POINT('Ctrl Pts',(-3.53352362388965,-3.59375490220193,
-3.66289634246604));
#75467=CARTESIAN_POINT('Ctrl Pts',(-3.42574928235742,0.73967021363975,-5.29832594739868));
#75468=CARTESIAN_POINT('Ctrl Pts',(-3.30648330994026,4.85615013534878,-2.24436532961465));
#75469=CARTESIAN_POINT('Ctrl Pts',(-3.18721733752309,4.51476892709962,2.86988351762224));
#75470=CARTESIAN_POINT('Ctrl Pts',(-3.06795136510593,0.0289085841635225,
5.34962934824326));
#75471=CARTESIAN_POINT('Ctrl Pts',(-2.96548103077721,-3.84803061328253,
3.2608714513295));
#75472=CARTESIAN_POINT('Ctrl Pts',(-2.90276602058755,-4.51376564796621,
0.871275981998934));
#75473=CARTESIAN_POINT('Ctrl Pts',(-2.87980633453694,-4.51700722203196,
-0.00187082749320257));
#75474=CARTESIAN_POINT('Ctrl Pts',(-3.48199366546304,-4.51776292098496,
-0.00258343477365669));
#75475=CARTESIAN_POINT('Ctrl Pts',(-3.46653654058934,-4.52080615393757,
-0.59016526618593));
#75476=CARTESIAN_POINT('Ctrl Pts',(-3.41132409157659,-4.14089776643248,
-2.6852100500767));
#75477=CARTESIAN_POINT('Ctrl Pts',(-3.31635631842477,-0.97436265912244,
-5.26022699703307));
#75478=CARTESIAN_POINT('Ctrl Pts',(-3.19709034600761,3.89680154001646,-3.66528421947511));
#75479=CARTESIAN_POINT('Ctrl Pts',(-3.07782437359044,5.19076988807344,1.29432554671451));
#75480=CARTESIAN_POINT('Ctrl Pts',(-2.95855840117328,1.71970200914856,5.0657670348663));
#75481=CARTESIAN_POINT('Ctrl Pts',(-2.84328149846415,-3.16112500776204,
4.21631729843839));
#75482=CARTESIAN_POINT('Ctrl Pts',(-2.76775991989407,-4.52013348714372,
1.34812538121587));
#75483=CARTESIAN_POINT('Ctrl Pts',(-2.73199366546304,-4.52935956130001,
-0.00259321422128662));
#75484=CARTESIAN_POINT('Origin',(-19.0048063345371,0.,0.));
#75485=CARTESIAN_POINT('',(-4.37980633453694,-4.53121768806138,1.67337722143111E-5));
#75486=CARTESIAN_POINT('',(-4.23199366546304,-4.51989857042376,0.00365667477888132));
#75487=CARTESIAN_POINT('',(-19.0048063345371,-4.52375,5.14627461305311E-12));
#75488=CARTESIAN_POINT('Ctrl Pts',(-4.37980633453694,-4.53121768806138,
1.6733772214251E-5));
#75489=CARTESIAN_POINT('Ctrl Pts',(-4.34007458611715,-4.53113573122214,
-1.49882557159262));
#75490=CARTESIAN_POINT('Ctrl Pts',(-4.2605875135583,-2.8958932222745,-4.49755267314905));
#75491=CARTESIAN_POINT('Ctrl Pts',(-4.14134511686041,2.21520613519663,-4.86952067953422));
#75492=CARTESIAN_POINT('Ctrl Pts',(-4.02207914444325,5.29379542366406,-0.771427172335632));
#75493=CARTESIAN_POINT('Ctrl Pts',(-3.90281317202608,3.51277284030709,4.03482302489525));
#75494=CARTESIAN_POINT('Ctrl Pts',(-3.78354719960892,-1.49291394549895,
5.13717605510642));
#75495=CARTESIAN_POINT('Ctrl Pts',(-3.69254492044586,-4.2666565334125,2.38001604204234));
#75496=CARTESIAN_POINT('Ctrl Pts',(-3.64129796542187,-4.52492915609762,
0.439981338626065));
#75497=CARTESIAN_POINT('Ctrl Pts',(-3.62980633453693,-4.52125034636371,
0.00399034990006115));
#75498=CARTESIAN_POINT('Ctrl Pts',(-4.23199366546304,-4.51989857042376,
0.00365667477888139));
#75499=CARTESIAN_POINT('Ctrl Pts',(-4.20506848542367,-4.51216606523885,
-1.01865332044624));
#75500=CARTESIAN_POINT('Ctrl Pts',(-4.13838798124524,-3.66181433414549,
-3.5620610773861));
#75501=CARTESIAN_POINT('Ctrl Pts',(-4.03195215292777,0.561046973578825,
-5.32020647580954));
#75502=CARTESIAN_POINT('Ctrl Pts',(-3.91268618051059,4.77791530080097,-2.40642806461773));
#75503=CARTESIAN_POINT('Ctrl Pts',(-3.79342020809343,4.60874071171544,2.71640934028442));
#75504=CARTESIAN_POINT('Ctrl Pts',(-3.67415423567627,0.208822528592261,
5.3456303466813));
#75505=CARTESIAN_POINT('Ctrl Pts',(-3.5703453881328,-3.78770815692856,3.36288627847629));
#75506=CARTESIAN_POINT('Ctrl Pts',(-3.50629186472839,-4.51297903774032,
0.921079959357981));
#75507=CARTESIAN_POINT('Ctrl Pts',(-3.48199366546304,-4.51776292098496,
-0.00258343477365669));
#75508=CARTESIAN_POINT('Origin',(-19.0048063345371,0.,0.));
#75509=CARTESIAN_POINT('',(-5.12980633453694,-4.5213004327236,-0.00399911873852178));
#75510=CARTESIAN_POINT('',(-4.98199366546304,-4.5309724658868,0.000956350713833126));
#75511=CARTESIAN_POINT('',(-19.0048063345371,-4.52375,5.14627461305311E-12));
#75512=CARTESIAN_POINT('Ctrl Pts',(-5.12980633453694,-4.5213004327236,-0.00399911873852177));
#75513=CARTESIAN_POINT('Ctrl Pts',(-5.11836185509054,-4.52497523886784,
-0.438189005660487));
#75514=CARTESIAN_POINT('Ctrl Pts',(-5.06716205150508,-4.26803848439264,
-2.37638847486489));
#75515=CARTESIAN_POINT('Ctrl Pts',(-4.97620692378056,-1.49900068010318,
-5.13540327830972));
#75516=CARTESIAN_POINT('Ctrl Pts',(-4.8569409513634,3.50798892841612,-4.03898298435808));
#75517=CARTESIAN_POINT('Ctrl Pts',(-4.73767497894623,5.29470588216781,0.765153246847895));
#75518=CARTESIAN_POINT('Ctrl Pts',(-4.61840900652908,2.22097517906763,4.86689214219808));
#75519=CARTESIAN_POINT('Ctrl Pts',(-4.4991430341119,-2.89157200322203,4.50090893264979));
#75520=CARTESIAN_POINT('Ctrl Pts',(-4.41960881011453,-4.53081425398383,
1.50152710822327));
#75521=CARTESIAN_POINT('Ctrl Pts',(-4.37982991025621,-4.53121773669229,
0.000906105290546244));
#75522=CARTESIAN_POINT('Ctrl Pts',(-4.37980633453694,-4.53121768806138,
1.6733772214251E-5));
#75523=CARTESIAN_POINT('Ctrl Pts',(-4.98199366546304,-4.5309724658868,0.000956350713833048));
#75524=CARTESIAN_POINT('Ctrl Pts',(-4.943600430258,-4.5268105339362,-1.44760255615506));
#75525=CARTESIAN_POINT('Ctrl Pts',(-4.8654518709139,-2.98832627775091,-4.40370984899896));
#75526=CARTESIAN_POINT('Ctrl Pts',(-4.74754798743075,2.05017057992043,-4.94127222939968));
#75527=CARTESIAN_POINT('Ctrl Pts',(-4.62828201501358,5.26485402104248,-0.949043091182221));
#75528=CARTESIAN_POINT('Ctrl Pts',(-4.50901604259642,3.64649329319062,3.91439105283614));
#75529=CARTESIAN_POINT('Ctrl Pts',(-4.38975007017925,-1.31928468068921,
5.18448247977621));
#75530=CARTESIAN_POINT('Ctrl Pts',(-4.29740927780146,-4.22633141630272,
2.48301617388978));
#75531=CARTESIAN_POINT('Ctrl Pts',(-4.24482380956272,-4.52358319409679,
0.490798619014908));
#75532=CARTESIAN_POINT('Ctrl Pts',(-4.23199366546304,-4.51989857042376,
0.00365667477888139));
#75533=CARTESIAN_POINT('Origin',(-19.0048063345371,0.,0.));
#75534=CARTESIAN_POINT('',(-5.87980633453694,-4.51698519435381,0.00184419225129259));
#75535=CARTESIAN_POINT('',(-5.73199366546304,-4.52277473914781,-0.00415818099157916));
#75536=CARTESIAN_POINT('',(-19.0048063345371,-4.52375,5.14627461305311E-12));
#75537=CARTESIAN_POINT('Ctrl Pts',(-5.87980633453694,-4.51698519435381,
0.00184419225129261));
#75538=CARTESIAN_POINT('Ctrl Pts',(-5.85689379992486,-4.51379722466762,
-0.869520083832802));
#75539=CARTESIAN_POINT('Ctrl Pts',(-5.79422594117374,-3.85010936700085,
-3.25727232317951));
#75540=CARTESIAN_POINT('Ctrl Pts',(-5.69180275828355,0.0225690143544715,
-5.34965984987971));
#75541=CARTESIAN_POINT('Ctrl Pts',(-5.57253678586638,4.51136481694416,-2.87523170514354));
#75542=CARTESIAN_POINT('Ctrl Pts',(-5.45327081344922,4.85880639859978,2.23860899907733));
#75543=CARTESIAN_POINT('Ctrl Pts',(-5.33400484103205,0.745948446959714,
5.29744568488459));
#75544=CARTESIAN_POINT('Ctrl Pts',(-5.22618334806129,-3.59130840982308,
3.66643927470266));
#75545=CARTESIAN_POINT('Ctrl Pts',(-5.15811717922959,-4.51220986058247,
1.07008052929913));
#75546=CARTESIAN_POINT('Ctrl Pts',(-5.12980633453694,-4.5213004327236,-0.00399911873852177));
#75547=CARTESIAN_POINT('Ctrl Pts',(-5.73199366546304,-4.52277473914781,
-0.00415818099157958));
#75548=CARTESIAN_POINT('Ctrl Pts',(-5.72188769923138,-4.52623711933511,
-0.387249167118643));
#75549=CARTESIAN_POINT('Ctrl Pts',(-5.67202640886067,-4.30619055181852,
-2.27344188077484));
#75550=CARTESIAN_POINT('Ctrl Pts',(-5.5824097943509,-1.67087756910494,-5.08208016474257));
#75551=CARTESIAN_POINT('Ctrl Pts',(-5.46314382193374,3.37015638858599,-4.15468609744235));
#75552=CARTESIAN_POINT('Ctrl Pts',(-5.34387784951657,5.31744555918776,0.586637346988937));
#75553=CARTESIAN_POINT('Ctrl Pts',(-5.22461187709941,2.38341244602753,4.7894379382062));
#75554=CARTESIAN_POINT('Ctrl Pts',(-5.10534590468224,-2.73855172438397,
4.59561803293978));
#75555=CARTESIAN_POINT('Ctrl Pts',(-5.02447316747012,-4.50701785980123,
1.60354636847148));
#75556=CARTESIAN_POINT('Ctrl Pts',(-4.98335575439705,-4.53112012006139,
0.0523473326608906));
#75557=CARTESIAN_POINT('Ctrl Pts',(-4.98199366546304,-4.5309724658868,0.000956350713833048));
#75558=CARTESIAN_POINT('Origin',(-19.0048063345371,0.,0.));
#75559=CARTESIAN_POINT('',(-6.62980633453694,-4.52807551305362,0.00326271820855672));
#75560=CARTESIAN_POINT('',(-6.48199366546304,-4.51649700603775,0.0010553308724473));
#75561=CARTESIAN_POINT('',(-19.0048063345371,-4.52375,5.14627461305311E-12));
#75562=CARTESIAN_POINT('Ctrl Pts',(-6.62980633453694,-4.52807551305362,
0.00326271820855709));
#75563=CARTESIAN_POINT('Ctrl Pts',(-6.59542574475919,-4.51751162682835,
-1.29609075831453));
#75564=CARTESIAN_POINT('Ctrl Pts',(-6.52128983084239,-3.24773613231329,
-4.11594224841461));
#75565=CARTESIAN_POINT('Ctrl Pts',(-6.40739859278654,1.54227677916538,-5.12257281122204));
#75566=CARTESIAN_POINT('Ctrl Pts',(-6.28813262036938,5.14255591405802,-1.47427559859448));
#75567=CARTESIAN_POINT('Ctrl Pts',(-6.16886664795221,4.0220584092331,3.52738090125541));
#75568=CARTESIAN_POINT('Ctrl Pts',(-6.04960067553505,-0.790618568056538,
5.2909632534793));
#75569=CARTESIAN_POINT('Ctrl Pts',(-5.95324723772995,-4.09237462138663,
2.79182142727619));
#75570=CARTESIAN_POINT('Ctrl Pts',(-5.89664912406392,-4.5193286410022,0.64237590783374));
#75571=CARTESIAN_POINT('Ctrl Pts',(-5.87980633453694,-4.51698519435381,
0.00184419225129261));
#75572=CARTESIAN_POINT('Ctrl Pts',(-6.48199366546304,-4.51649700603775,
0.00105533087244723));
#75573=CARTESIAN_POINT('Ctrl Pts',(-6.46041964406571,-4.514789747878,-0.819626683720531));
#75574=CARTESIAN_POINT('Ctrl Pts',(-6.39909029852933,-3.90782509244913,
-3.15496527216252));
#75575=CARTESIAN_POINT('Ctrl Pts',(-6.29800562885389,-0.157375080700092,
-5.34739223694899));
#75576=CARTESIAN_POINT('Ctrl Pts',(-6.17873965643672,4.41210639136683,-3.02534094658233));
#75577=CARTESIAN_POINT('Ctrl Pts',(-6.05947368401956,4.93135114605077,2.07392056891087));
#75578=CARTESIAN_POINT('Ctrl Pts',(-5.94020771160239,0.923701554504711,
5.2693591726142));
#75579=CARTESIAN_POINT('Ctrl Pts',(-5.83104770541689,-3.5204528709042,3.76673040395475));
#75580=CARTESIAN_POINT('Ctrl Pts',(-5.76164302337044,-4.51261664569771,
1.11977212892738));
#75581=CARTESIAN_POINT('Ctrl Pts',(-5.73199366546304,-4.52277473914781,
-0.00415818099157958));
#75582=CARTESIAN_POINT('Origin',(-19.0048063345371,0.,0.));
#75583=CARTESIAN_POINT('',(-7.37980633453694,-4.52733122205943,-0.00354293946284749));
#75584=CARTESIAN_POINT('',(-7.23199366546304,-4.5266579896236,0.00374494774771153));
#75585=CARTESIAN_POINT('',(-19.0048063345371,-4.52375,5.14627461305311E-12));
#75586=CARTESIAN_POINT('Ctrl Pts',(-7.37980633453694,-4.52733122205943,
-0.00354293946284695));
#75587=CARTESIAN_POINT('Ctrl Pts',(-7.37371301373258,-4.52931362694418,
-0.233927783108747));
#75588=CARTESIAN_POINT('Ctrl Pts',(-7.32786436878916,-4.40845915531641,
-1.96535187413747));
#75589=CARTESIAN_POINT('Ctrl Pts',(-7.24226039970668,-2.17404118518495,
-4.88803792895919));
#75590=CARTESIAN_POINT('Ctrl Pts',(-7.12299442728953,2.93474766896221,-4.4728767017821));
#75591=CARTESIAN_POINT('Ctrl Pts',(-7.00372845487236,5.34948934683475,0.0483073278670784));
#75592=CARTESIAN_POINT('Ctrl Pts',(-6.8844624824552,2.85349310274905,4.52514607304423));
#75593=CARTESIAN_POINT('Ctrl Pts',(-6.76519651003803,-2.26196004295795,
4.84797964454119));
#75594=CARTESIAN_POINT('Ctrl Pts',(-6.68031112739861,-4.42492236636027,
1.91028737732804));
#75595=CARTESIAN_POINT('Ctrl Pts',(-6.63518106889825,-4.52972697053736,
0.206391280659083));
#75596=CARTESIAN_POINT('Ctrl Pts',(-6.62980633453694,-4.52807551305362,
0.00326271820855709));
#75597=CARTESIAN_POINT('Ctrl Pts',(-7.23199366546304,-4.5266579896236,0.00374494774771174));
#75598=CARTESIAN_POINT('Ctrl Pts',(-7.19895158890004,-4.51552227061198,
-1.2460383771676));
#75599=CARTESIAN_POINT('Ctrl Pts',(-7.12615418819799,-3.32846977442805,
-4.01809588963737));
#75600=CARTESIAN_POINT('Ctrl Pts',(-7.01360146335687,1.36911075397815,-5.17154777558412));
#75601=CARTESIAN_POINT('Ctrl Pts',(-6.89433549093971,5.09006036110679,-1.64640704933419));
#75602=CARTESIAN_POINT('Ctrl Pts',(-6.77506951852255,4.13842333057186,3.3901066338371));
#75603=CARTESIAN_POINT('Ctrl Pts',(-6.65580354610538,-0.612214140739847,
5.31456155272341));
#75604=CARTESIAN_POINT('Ctrl Pts',(-6.55811159508555,-4.04316743284744,
2.89473048394592));
#75605=CARTESIAN_POINT('Ctrl Pts',(-6.50017496820477,-4.51793578172491,
0.692677346406831));
#75606=CARTESIAN_POINT('Ctrl Pts',(-6.48199366546304,-4.51649700603775,
0.00105533087244723));
#75607=CARTESIAN_POINT('Origin',(-19.0048063345371,0.,0.));
#75608=CARTESIAN_POINT('',(-8.12980633453695,-4.51668977813578,-0.00142781023108144));
#75609=CARTESIAN_POINT('',(-7.98199366546304,-4.52867803382547,-0.00298322746560442));
#75610=CARTESIAN_POINT('',(-19.0048063345371,-4.52375,5.14627461305311E-12));
#75611=CARTESIAN_POINT('Ctrl Pts',(-8.12980633453695,-4.51668977813578,
-0.00142781023108107));
#75612=CARTESIAN_POINT('Ctrl Pts',(-8.11224495856691,-4.51857450838071,
-0.669396461747199));
#75613=CARTESIAN_POINT('Ctrl Pts',(-8.05492825845782,-4.06624602752072,
-2.84708018096034));
#75614=CARTESIAN_POINT('Ctrl Pts',(-7.95785623420967,-0.694939784074152,
-5.30437824502882));
#75615=CARTESIAN_POINT('Ctrl Pts',(-7.83859026179251,4.08510370142725,-3.45417104648997));
#75616=CARTESIAN_POINT('Ctrl Pts',(-7.71932428937535,5.11509323577896,1.56690492982581));
#75617=CARTESIAN_POINT('Ctrl Pts',(-7.60005831695818,1.44951639010705,5.1495895083623));
#75618=CARTESIAN_POINT('Ctrl Pts',(-7.48688566534538,-3.29143404128054,
4.06351594110314));
#75619=CARTESIAN_POINT('Ctrl Pts',(-7.41346833787163,-4.51637960438101,
1.26919743053686));
#75620=CARTESIAN_POINT('Ctrl Pts',(-7.37980633453694,-4.52733122205943,
-0.00354293946284695));
#75621=CARTESIAN_POINT('Ctrl Pts',(-7.98199366546304,-4.52867803382547,
-0.00298322746560407));
#75622=CARTESIAN_POINT('Ctrl Pts',(-7.97723885787343,-4.53004555346133,
-0.182620278006116));
#75623=CARTESIAN_POINT('Ctrl Pts',(-7.93272872614476,-4.43868714409182,
-1.86281378505977));
#75624=CARTESIAN_POINT('Ctrl Pts',(-7.84846327027703,-2.33721622703428,
-4.8121503467676));
#75625=CARTESIAN_POINT('Ctrl Pts',(-7.72919729785987,2.78264580301424,-4.56905383933861));
#75626=CARTESIAN_POINT('Ctrl Pts',(-7.60993132544269,5.34808751697683,-0.131645594550073));
#75627=CARTESIAN_POINT('Ctrl Pts',(-7.49066535302554,3.00407816434195,4.42661101005405));
#75628=CARTESIAN_POINT('Ctrl Pts',(-7.37139938060837,-2.09762255015898,
4.92131591028987));
#75629=CARTESIAN_POINT('Ctrl Pts',(-7.28517548475421,-4.39381329989842,
2.01288556324745));
#75630=CARTESIAN_POINT('Ctrl Pts',(-7.2387069130391,-4.52892046360946,0.257666787695734));
#75631=CARTESIAN_POINT('Ctrl Pts',(-7.23199366546304,-4.5266579896236,0.00374494774771174));
#75632=CARTESIAN_POINT('Origin',(-19.0048063345371,0.,0.));
#75633=CARTESIAN_POINT('',(-8.87980633453694,-4.52208054885539,0.00410638580840894));
#75634=CARTESIAN_POINT('',(-8.73199366546304,-4.51730023616471,-0.0021866156284378));
#75635=CARTESIAN_POINT('',(-19.0048063345371,-4.52375,5.14627461305311E-12));
#75636=CARTESIAN_POINT('Ctrl Pts',(-8.87980633453694,-4.52208054885539,
0.00410638580840929));
#75637=CARTESIAN_POINT('Ctrl Pts',(-8.85077690340124,-4.51238109141432,
-1.0967537268227));
#75638=CARTESIAN_POINT('Ctrl Pts',(-8.78199214812648,-3.55360792181159,
-3.72035082563007));
#75639=CARTESIAN_POINT('Ctrl Pts',(-8.67345206871266,0.841493716983345,
-5.28311065510666));
#75640=CARTESIAN_POINT('Ctrl Pts',(-8.55418609629549,4.8984412193819,-2.15049842829157));
#75641=CARTESIAN_POINT('Ctrl Pts',(-8.43492012387834,4.45870511426281,2.9562338496592));
#75642=CARTESIAN_POINT('Ctrl Pts',(-8.31565415146116,-0.0740445231469701,
5.3491950121879));
#75643=CARTESIAN_POINT('Ctrl Pts',(-8.21394955501404,-3.88140416868336,
3.20237992240633));
#75644=CARTESIAN_POINT('Ctrl Pts',(-8.15200028270597,-4.51430786880021,
0.842746453538187));
#75645=CARTESIAN_POINT('Ctrl Pts',(-8.12980633453695,-4.51668977813578,
-0.00142781023108107));
#75646=CARTESIAN_POINT('Ctrl Pts',(-8.73199366546304,-4.51730023616471,
-0.0021866156284378));
#75647=CARTESIAN_POINT('Ctrl Pts',(-8.71577080270775,-4.51998733949217,
-0.619035001797185));
#75648=CARTESIAN_POINT('Ctrl Pts',(-8.65979261581342,-4.1143840503259,-2.74413231667926));
#75649=CARTESIAN_POINT('Ctrl Pts',(-8.56405910478001,-0.872954921887009,
-5.27800344412176));
#75650=CARTESIAN_POINT('Ctrl Pts',(-8.44479313236285,3.96661430405479,-3.58961580321287));
#75651=CARTESIAN_POINT('Ctrl Pts',(-8.32552715994568,5.16490077910572,1.39397653990334));
#75652=CARTESIAN_POINT('Ctrl Pts',(-8.20626118752853,1.62189841803372,5.09792273121));
#75653=CARTESIAN_POINT('Ctrl Pts',(-8.09175002270096,-3.20937125987305,
4.16096954991165));
#75654=CARTESIAN_POINT('Ctrl Pts',(-8.01699418201248,-4.51861161310398,
1.31933937798815));
#75655=CARTESIAN_POINT('Ctrl Pts',(-7.98199366546304,-4.52867803382547,
-0.00298322746560407));
#75656=CARTESIAN_POINT('Origin',(-19.0048063345371,0.,0.));
#75657=CARTESIAN_POINT('',(-9.62980633453695,-4.53114288885854,-0.00052505224322001));
#75658=CARTESIAN_POINT('',(-9.48199366546304,-4.52065448282384,0.00386729026705834));
#75659=CARTESIAN_POINT('',(-19.0048063345371,-4.52375,5.14627461305311E-12));
#75660=CARTESIAN_POINT('Ctrl Pts',(-9.62980633453694,-4.53114288885854,
-0.000525052243220102));
#75661=CARTESIAN_POINT('Ctrl Pts',(-9.62906417237462,-4.53118872991189,
-0.0285236575162823));
#75662=CARTESIAN_POINT('Ctrl Pts',(-9.58856668607325,-4.51825661700592,
-1.55627717876711));
#75663=CARTESIAN_POINT('Ctrl Pts',(-9.50831387563282,-2.80981824212958,
-4.55239402029525));
#75664=CARTESIAN_POINT('Ctrl Pts',(-9.38904790321564,2.30850450978291,-4.82598972213328));
#75665=CARTESIAN_POINT('Ctrl Pts',(-9.26978193079849,5.30766038347549,-0.669411027328533));
#75666=CARTESIAN_POINT('Ctrl Pts',(-9.15051595838132,3.43447659405036,4.10167531561732));
#75667=CARTESIAN_POINT('Ctrl Pts',(-9.03124998596416,-1.59149680929566,
5.10749525460629));
#75668=CARTESIAN_POINT('Ctrl Pts',(-8.9410134446827,-4.28877837960027,2.3211131273353));
#75669=CARTESIAN_POINT('Ctrl Pts',(-8.89053222754029,-4.52566433739803,
0.410855926456967));
#75670=CARTESIAN_POINT('Ctrl Pts',(-8.87980633453694,-4.52208054885539,
0.00410638580840929));
#75671=CARTESIAN_POINT('Ctrl Pts',(-9.48199366546304,-4.52065448282384,
0.003867290267058));
#75672=CARTESIAN_POINT('Ctrl Pts',(-9.45430274754209,-4.51214545629191,
-1.04707296981455));
#75673=CARTESIAN_POINT('Ctrl Pts',(-9.38685650548208,-3.62320685191578,
-3.61980730776049));
#75674=CARTESIAN_POINT('Ctrl Pts',(-9.279654939283,0.663324621354469,-5.30842454015434));
#75675=CARTESIAN_POINT('Ctrl Pts',(-9.16038896686585,4.82333959217,-2.31403669599532));
#75676=CARTESIAN_POINT('Ctrl Pts',(-9.04112299444865,4.55561293942915,2.80459647684182));
#75677=CARTESIAN_POINT('Ctrl Pts',(-8.92185702203153,0.105913061027885,
5.34865899785279));
#75678=CARTESIAN_POINT('Ctrl Pts',(-8.81881391236962,-3.82252862056392,
3.30456340422465));
#75679=CARTESIAN_POINT('Ctrl Pts',(-8.7555261268468,-4.51340239419676,0.892597556938324));
#75680=CARTESIAN_POINT('Ctrl Pts',(-8.73199366546304,-4.51730023616471,
-0.0021866156284378));
#75681=CARTESIAN_POINT('Origin',(-19.0048063345371,0.,0.));
#75682=CARTESIAN_POINT('',(-10.3798063345369,-4.52050667523945,-0.00383117177063042));
#75683=CARTESIAN_POINT('',(-10.231993665463,-4.53116917314862,0.000422383571537207));
#75684=CARTESIAN_POINT('',(-19.0048063345371,-4.52375,5.14627461305311E-12));
#75685=CARTESIAN_POINT('Ctrl Pts',(-10.3798063345369,-4.52050667523944,
-0.00383117177062971));
#75686=CARTESIAN_POINT('Ctrl Pts',(-10.367596117209,-4.52421503063526,-0.467278015537651));
#75687=CARTESIAN_POINT('Ctrl Pts',(-10.3156305757419,-4.24527193127081,
-2.43530731245446));
#75688=CARTESIAN_POINT('Ctrl Pts',(-10.2239097101358,-1.39989788550755,
-5.1632989241352));
#75689=CARTESIAN_POINT('Ctrl Pts',(-10.1046437377186,3.5850651163716,-3.97072763875836));
#75690=CARTESIAN_POINT('Ctrl Pts',(-9.98537776530147,5.27900086719687,0.866902367028086));
#75691=CARTESIAN_POINT('Ctrl Pts',(-9.86611179288431,2.12690589100833,4.90873111920161));
#75692=CARTESIAN_POINT('Ctrl Pts',(-9.74758798262946,-2.9458872206108,4.4473195424606));
#75693=CARTESIAN_POINT('Ctrl Pts',(-9.66881949651368,-4.52873316692682,
1.4712747485241));
#75694=CARTESIAN_POINT('Ctrl Pts',(-9.62980633453694,-4.53114288885854,
-0.000525052243220102));
#75695=CARTESIAN_POINT('Ctrl Pts',(-10.231993665463,-4.53116917314862,0.000422383571537441));
#75696=CARTESIAN_POINT('Ctrl Pts',(-10.1928346923764,-4.52920551616272,
-1.47685525433921));
#75697=CARTESIAN_POINT('Ctrl Pts',(-10.1139203951507,-2.93581244463462,
-4.4575405446346));
#75698=CARTESIAN_POINT('Ctrl Pts',(-9.995250773786,2.14488029590958,-4.90090391336402));
#75699=CARTESIAN_POINT('Ctrl Pts',(-9.87598480136882,5.28214236395734,-0.847551000645274));
#75700=CARTESIAN_POINT('Ctrl Pts',(-9.75671882895166,3.57048986575489,3.98383894884689));
#75701=CARTESIAN_POINT('Ctrl Pts',(-9.6374528565345,-1.41881005763682,5.15813422393762));
#75702=CARTESIAN_POINT('Ctrl Pts',(-9.54587780203829,-4.2496605265107,2.42408697318163));
#75703=CARTESIAN_POINT('Ctrl Pts',(-9.49405807168114,-4.52436170383019,
0.461741971228011));
#75704=CARTESIAN_POINT('Ctrl Pts',(-9.48199366546304,-4.52065448282384,
0.003867290267058));
#75705=CARTESIAN_POINT('Origin',(-19.0048063345371,0.,0.));
#75706=CARTESIAN_POINT('',(-11.1298063345369,-4.51738211886999,0.00226454645098684));
#75707=CARTESIAN_POINT('',(-10.981993665463,-4.52191995054341,-0.00408866953903741));
#75708=CARTESIAN_POINT('',(-19.0048063345371,-4.52375,5.14627461305311E-12));
#75709=CARTESIAN_POINT('Ctrl Pts',(-11.1298063345369,-4.51738211886999,
0.00226454645098691));
#75710=CARTESIAN_POINT('Ctrl Pts',(-11.1061280620433,-4.51331604098809,
-0.89802300770951));
#75711=CARTESIAN_POINT('Ctrl Pts',(-11.0426944654106,-3.81596241879828,
-3.3156771965644));
#75712=CARTESIAN_POINT('Ctrl Pts',(-10.9395055446388,0.125513175958816,
-5.3482348782084));
#75713=CARTESIAN_POINT('Ctrl Pts',(-10.8202395722216,4.56586008070243,-2.78788299490349));
#75714=CARTESIAN_POINT('Ctrl Pts',(-10.7009735998044,4.81482706281336,2.3316968553018));
#75715=CARTESIAN_POINT('Ctrl Pts',(-10.5817076273873,0.643866774853417,
5.31081965858981));
#75716=CARTESIAN_POINT('Ctrl Pts',(-10.4746518722981,-3.63062580284369,
3.60882339659679));
#75717=CARTESIAN_POINT('Ctrl Pts',(-10.407351441348,-4.51214097275215,1.04166150619729));
#75718=CARTESIAN_POINT('Ctrl Pts',(-10.3798063345369,-4.52050667523944,
-0.00383117177062971));
#75719=CARTESIAN_POINT('Ctrl Pts',(-10.981993665463,-4.52191995054341,-0.00408866953903672));
#75720=CARTESIAN_POINT('Ctrl Pts',(-10.9711219613498,-4.52552666035439,
-0.416404890679838));
#75721=CARTESIAN_POINT('Ctrl Pts',(-10.9204949330975,-4.28461857606984,
-2.33232788952565));
#75722=CARTESIAN_POINT('Ctrl Pts',(-10.8301125807061,-1.57276909104567,
-5.11329326736293));
#75723=CARTESIAN_POINT('Ctrl Pts',(-10.710846608289,3.44948468012718,-4.08906176199085));
#75724=CARTESIAN_POINT('Ctrl Pts',(-10.5915806358718,5.30517167611101,0.688857125097259));
#75725=CARTESIAN_POINT('Ctrl Pts',(-10.4723146634547,2.29080359893313,4.83441718544467));
#75726=CARTESIAN_POINT('Ctrl Pts',(-10.3530486910375,-2.82648222901952,
4.54206658480968));
#75727=CARTESIAN_POINT('Ctrl Pts',(-10.272941691707,-4.52084542429402,1.54516401016659));
#75728=CARTESIAN_POINT('Ctrl Pts',(-10.2325900165155,-4.53119907763328,
0.0229198089290014));
#75729=CARTESIAN_POINT('Ctrl Pts',(-10.231993665463,-4.53116917314862,0.000422383571537441));
#75730=CARTESIAN_POINT('Origin',(-19.0048063345371,0.,0.));
#75731=CARTESIAN_POINT('',(-11.8798063345369,-4.52881345908333,0.00291265612866996));
#75732=CARTESIAN_POINT('',(-11.731993665463,-4.51674360781622,0.00151377565128424));
#75733=CARTESIAN_POINT('',(-19.0048063345371,-4.52375,5.14627461305311E-12));
#75734=CARTESIAN_POINT('Ctrl Pts',(-11.8798063345369,-4.52881345908333,
0.00291265612866994));
#75735=CARTESIAN_POINT('Ctrl Pts',(-11.8446600068776,-4.51888726912132,
-1.32481461068629));
#75736=CARTESIAN_POINT('Ctrl Pts',(-11.7697583550792,-3.20025743132486,
-4.17153219074509));
#75737=CARTESIAN_POINT('Ctrl Pts',(-11.6551013791418,1.64056947847539,-5.09194478133052));
#75738=CARTESIAN_POINT('Ctrl Pts',(-11.5358354067246,5.16997442825406,-1.37503973797965));
#75739=CARTESIAN_POINT('Ctrl Pts',(-11.4165694343074,3.95343302047925,3.60412780328452));
#75740=CARTESIAN_POINT('Ctrl Pts',(-11.2973034618903,-0.892290949753927,
5.2747688793739));
#75741=CARTESIAN_POINT('Ctrl Pts',(-11.2017157619668,-4.11948975774644,
2.73291356932791));
#75742=CARTESIAN_POINT('Ctrl Pts',(-11.1458833861823,-4.52014290068459,
0.613540960632567));
#75743=CARTESIAN_POINT('Ctrl Pts',(-11.1298063345369,-4.51738211886999,
0.00226454645098691));
#75744=CARTESIAN_POINT('Ctrl Pts',(-11.731993665463,-4.51674360781622,0.00151377565128417));
#75745=CARTESIAN_POINT('Ctrl Pts',(-11.7096539061841,-4.51419998793741,
-0.848181357999456));
#75746=CARTESIAN_POINT('Ctrl Pts',(-11.6475588227661,-3.87511238866226,
-3.21352454637504));
#75747=CARTESIAN_POINT('Ctrl Pts',(-11.5457084152091,-0.0544412345818395,
-5.34943051209986));
#75748=CARTESIAN_POINT('Ctrl Pts',(-11.4264424427919,4.46950872374863,-2.93987455857264));
#75749=CARTESIAN_POINT('Ctrl Pts',(-11.3071764703748,4.89052762470212,2.16843496647541));
#75750=CARTESIAN_POINT('Ctrl Pts',(-11.1879104979576,0.822127460035971,
5.28615901115948));
#75751=CARTESIAN_POINT('Ctrl Pts',(-11.0795162296537,-3.56132121802685,
3.70942426675612));
#75752=CARTESIAN_POINT('Ctrl Pts',(-11.0108772854889,-4.51233775122686,
1.0913407992777));
#75753=CARTESIAN_POINT('Ctrl Pts',(-10.981993665463,-4.52191995054341,-0.00408866953903672));
#75754=CARTESIAN_POINT('Origin',(-19.0048063345371,0.,0.));
#75755=CARTESIAN_POINT('',(-12.6298063345369,-4.52649620861785,-0.00378695143178565));
#75756=CARTESIAN_POINT('',(-12.4819936654631,-4.52748577852528,0.00349000897288482));
#75757=CARTESIAN_POINT('',(-19.0048063345371,-4.52375,5.14627461305311E-12));
#75758=CARTESIAN_POINT('Ctrl Pts',(-12.6298063345369,-4.52649620861785,
-0.0037869514317854));
#75759=CARTESIAN_POINT('Ctrl Pts',(-12.622947275851,-4.52882314301935,-0.263247936212846));
#75760=CARTESIAN_POINT('Ctrl Pts',(-12.576332893026,-4.39030829601886,-2.02406958410072));
#75761=CARTESIAN_POINT('Ctrl Pts',(-12.4899631860619,-2.07957366092086,
-4.92896979688741));
#75762=CARTESIAN_POINT('Ctrl Pts',(-12.3706972136447,3.02027981942101,-4.41557240708635));
#75763=CARTESIAN_POINT('Ctrl Pts',(-12.2514312412276,5.34756910110119,0.151243442078761));
#75764=CARTESIAN_POINT('Ctrl Pts',(-12.1321652688104,2.76588321291629,4.57922044919569));
#75765=CARTESIAN_POINT('Ctrl Pts',(-12.0128992963933,-2.35483522599469,
4.80355294841628));
#75766=CARTESIAN_POINT('Ctrl Pts',(-11.9287796516354,-4.44186617927913,
1.85165188822665));
#75767=CARTESIAN_POINT('Ctrl Pts',(-11.8844153310167,-4.53011515338936,
0.177027299288359));
#75768=CARTESIAN_POINT('Ctrl Pts',(-11.8798063345369,-4.52881345908333,
0.00291265612866994));
#75769=CARTESIAN_POINT('Ctrl Pts',(-12.481993665463,-4.52748577852528,0.00349000897288478));
#75770=CARTESIAN_POINT('Ctrl Pts',(-12.4481858510185,-4.51659720762945,
-1.27465003716645));
#75771=CARTESIAN_POINT('Ctrl Pts',(-12.3746227124348,-3.28263402910187,
-4.07417368335456));
#75772=CARTESIAN_POINT('Ctrl Pts',(-12.2613042497121,1.4683779898736,-5.14424306683332));
#75773=CARTESIAN_POINT('Ctrl Pts',(-12.142038277295,5.12080107761086,-1.54814953261863));
#75774=CARTESIAN_POINT('Ctrl Pts',(-12.0227723048778,4.07241808607112,3.46911827184497));
#75775=CARTESIAN_POINT('Ctrl Pts',(-11.9035063324606,-0.714373682966412,
5.30179600634471));
#75776=CARTESIAN_POINT('Ctrl Pts',(-11.8065801193224,-4.07160180796638,
2.83586945730652));
#75777=CARTESIAN_POINT('Ctrl Pts',(-11.7494092303232,-4.51872655563701,
0.663916647888202));
#75778=CARTESIAN_POINT('Ctrl Pts',(-11.731993665463,-4.51674360781622,0.00151377565128417));
#75779=CARTESIAN_POINT('Origin',(-19.0048063345371,0.,0.));
#75780=CARTESIAN_POINT('',(-13.3798063345369,-4.51646009003207,-0.000966303587493708));
#75781=CARTESIAN_POINT('',(-13.2319936654631,-4.52792820117867,-0.00332346547265827));
#75782=CARTESIAN_POINT('',(-19.0048063345371,-4.52375,5.14627461305311E-12));
#75783=CARTESIAN_POINT('Ctrl Pts',(-13.3798063345369,-4.51646009003207,
-0.000966303587493431));
#75784=CARTESIAN_POINT('Ctrl Pts',(-13.3614792206853,-4.51778745205074,
-0.69814919617005));
#75785=CARTESIAN_POINT('Ctrl Pts',(-13.3033967826947,-4.0376662333295,-2.90593474512968));
#75786=CARTESIAN_POINT('Ctrl Pts',(-13.2055590205649,-0.592734148285034,
-5.31676932913924));
#75787=CARTESIAN_POINT('Ctrl Pts',(-13.0862930481478,4.15081895382183,-3.37491805566053));
#75788=CARTESIAN_POINT('Ctrl Pts',(-12.9670270757306,5.08399264919423,1.66504913223642));
#75789=CARTESIAN_POINT('Ctrl Pts',(-12.8477611033134,1.35014976061496,5.17653025623679));
#75790=CARTESIAN_POINT('Ctrl Pts',(-12.7353541895822,-3.3370920331084,4.00738784074087));
#75791=CARTESIAN_POINT('Ctrl Pts',(-12.66270259999,-4.51533615659485,1.24059625344786));
#75792=CARTESIAN_POINT('Ctrl Pts',(-12.6298063345369,-4.52649620861785,
-0.0037869514317854));
#75793=CARTESIAN_POINT('Ctrl Pts',(-13.2319936654631,-4.52792820117867,
-0.00332346547265792));
#75794=CARTESIAN_POINT('Ctrl Pts',(-13.2264731199919,-4.52964693741261,
-0.211980413649894));
#75795=CARTESIAN_POINT('Ctrl Pts',(-13.1811972503816,-4.42162610491374,
-1.92145771095745));
#75796=CARTESIAN_POINT('Ctrl Pts',(-13.0961660566323,-2.24417885919362,
-4.85623639249116));
#75797=CARTESIAN_POINT('Ctrl Pts',(-12.9769000842151,2.8700569434679,-4.51465876817511));
#75798=CARTESIAN_POINT('Ctrl Pts',(-12.8576341117979,5.34963052761172,-0.0287031331433309));
#75799=CARTESIAN_POINT('Ctrl Pts',(-12.7383681393808,2.91833658830642,4.48360147751333));
#75800=CARTESIAN_POINT('Ctrl Pts',(-12.6191021669636,-2.19193944145102,
4.88003812862352));
#75801=CARTESIAN_POINT('Ctrl Pts',(-12.533644008991,-4.41184422699395,1.95417554456908));
#75802=CARTESIAN_POINT('Ctrl Pts',(-12.4879411751575,-4.52940130847082,
0.228341879470367));
#75803=CARTESIAN_POINT('Ctrl Pts',(-12.481993665463,-4.52748577852528,0.00349000897288478));
#75804=CARTESIAN_POINT('Origin',(-19.0048063345371,0.,0.));
#75805=CARTESIAN_POINT('',(-14.1298063345369,-4.52294015312425,0.00416476062241385));
#75806=CARTESIAN_POINT('',(-13.9819936654631,-4.51691917766224,-0.00176125576838326));
#75807=CARTESIAN_POINT('',(-19.0048063345371,-4.52375,5.14627461305311E-12));
#75808=CARTESIAN_POINT('Ctrl Pts',(-14.1298063345369,-4.52294015312425,
0.00416476062241395));
#75809=CARTESIAN_POINT('Ctrl Pts',(-14.1000111655197,-4.51268424282815,
-1.12518759832097));
#75810=CARTESIAN_POINT('Ctrl Pts',(-14.0304606723633,-3.51256915117181,
-3.77762082095125));
#75811=CARTESIAN_POINT('Ctrl Pts',(-13.9211548550679,0.943005562874773,
-5.26593869864046));
#75812=CARTESIAN_POINT('Ctrl Pts',(-13.8018888826508,4.93891810628447,-2.05583506379208));
#75813=CARTESIAN_POINT('Ctrl Pts',(-13.6826229102336,4.40098996586505,3.04148930462108));
#75814=CARTESIAN_POINT('Ctrl Pts',(-13.5633569378164,-0.176970207163579,
5.34677953683851));
#75815=CARTESIAN_POINT('Ctrl Pts',(-13.4624180792509,-3.91396229489176,
3.1438056354711));
#75816=CARTESIAN_POINT('Ctrl Pts',(-13.4012345448244,-4.51490812758485,
0.814185593869427));
#75817=CARTESIAN_POINT('Ctrl Pts',(-13.3798063345369,-4.51646009003207,
-0.000966303587493431));
#75818=CARTESIAN_POINT('Ctrl Pts',(-13.9819936654631,-4.51691917766224,
-0.00176125576838361));
#75819=CARTESIAN_POINT('Ctrl Pts',(-13.9650050648262,-4.51917472294271,
-0.647861788429469));
#75820=CARTESIAN_POINT('Ctrl Pts',(-13.9082611400502,-4.08712657467319,
-2.80303613492246));
#75821=CARTESIAN_POINT('Ctrl Pts',(-13.8117618911353,-0.771223875207531,
-5.29382511857655));
#75822=CARTESIAN_POINT('Ctrl Pts',(-13.6924959187181,4.03495798434998,-3.51261792917751));
#75823=CARTESIAN_POINT('Ctrl Pts',(-13.5732299463009,5.13711878645237,1.49311125696483));
#75824=CARTESIAN_POINT('Ctrl Pts',(-13.4539639738838,1.52349413715743,5.12819035000159));
#75825=CARTESIAN_POINT('Ctrl Pts',(-13.3402185469378,-3.25667002467314,
4.1053241526965));
#75826=CARTESIAN_POINT('Ctrl Pts',(-13.2662284441309,-4.51726973366597,
1.29062918388309));
#75827=CARTESIAN_POINT('Ctrl Pts',(-13.2319936654631,-4.52792820117867,
-0.00332346547265792));
#75828=CARTESIAN_POINT('Origin',(-19.0048063345371,0.,0.));
#75829=CARTESIAN_POINT('',(-14.879806334537,-4.53091903216787,-0.00105619164529906));
#75830=CARTESIAN_POINT('',(-14.7319936654631,-4.521456298353,0.00402490267532751));
#75831=CARTESIAN_POINT('',(-19.0048063345371,-4.52375,5.14627461305311E-12));
#75832=CARTESIAN_POINT('Ctrl Pts',(-14.8798063345369,-4.53091903216787,
-0.00105619164529849));
#75833=CARTESIAN_POINT('Ctrl Pts',(-14.878298434493,-4.53109805835402,-0.0579503522764566));
#75834=CARTESIAN_POINT('Ctrl Pts',(-14.8370352103101,-4.50431938173549,
-1.61466921124215));
#75835=CARTESIAN_POINT('Ctrl Pts',(-14.7560166619881,-2.72169207944861,
-4.60562287829862));
#75836=CARTESIAN_POINT('Ctrl Pts',(-14.6367506895709,2.40094789974828,-4.78067139956327));
#75837=CARTESIAN_POINT('Ctrl Pts',(-14.5174847171537,5.31955958788271,-0.56714695851215));
#75838=CARTESIAN_POINT('Ctrl Pts',(-14.3982187447365,3.35490834716323,4.16700850147134));
#75839=CARTESIAN_POINT('Ctrl Pts',(-14.2789527723194,-1.68949024264872,
5.07592283106375));
#75840=CARTESIAN_POINT('Ctrl Pts',(-14.1894819689195,-4.31022186693971,
2.26223150191539));
#75841=CARTESIAN_POINT('Ctrl Pts',(-14.1397664896587,-4.52636857661816,
0.38169323430466));
#75842=CARTESIAN_POINT('Ctrl Pts',(-14.1298063345369,-4.52294015312425,
0.00416476062241395));
#75843=CARTESIAN_POINT('Ctrl Pts',(-14.7319936654631,-4.521456298353,0.00402490267532758));
#75844=CARTESIAN_POINT('Ctrl Pts',(-14.7035370096605,-4.51223610990917,
-1.07549240604431));
#75845=CARTESIAN_POINT('Ctrl Pts',(-14.6353250297189,-3.58372170086442,
-3.67739134091624));
#75846=CARTESIAN_POINT('Ctrl Pts',(-14.5273577256382,0.765356598558913,
-5.29467656481004));
#75847=CARTESIAN_POINT('Ctrl Pts',(-14.4080917532211,4.86697750131595,-2.22078829592513));
#75848=CARTESIAN_POINT('Ctrl Pts',(-14.2888257808039,4.50079794053571,2.89174489712377));
#75849=CARTESIAN_POINT('Ctrl Pts',(-14.1695598083868,0.00296436731219236,
5.34970670821892));
#75850=CARTESIAN_POINT('Ctrl Pts',(-14.0672824366065,-3.85651800034967,
3.24614022654441));
#75851=CARTESIAN_POINT('Ctrl Pts',(-14.0047603889652,-4.51389648162949,
0.864089469439338));
#75852=CARTESIAN_POINT('Ctrl Pts',(-13.9819936654631,-4.51691917766224,
-0.00176125576838361));
#75853=CARTESIAN_POINT('Origin',(-19.0048063345371,0.,0.));
#75854=CARTESIAN_POINT('',(-15.6298063345369,-4.51976043794902,-0.00361086820214561));
#75855=CARTESIAN_POINT('',(-15.4819936654631,-4.5312138402642,-0.000120197794654664));
#75856=CARTESIAN_POINT('',(-19.0048063345371,-4.52375,5.14627461305311E-12));
#75857=CARTESIAN_POINT('Ctrl Pts',(-15.6298063345369,-4.51976043794902,
-0.00361086820214504));
#75858=CARTESIAN_POINT('Ctrl Pts',(-15.6168303793274,-4.52343268604556,
-0.496326928866944));
#75859=CARTESIAN_POINT('Ctrl Pts',(-15.5640990999787,-4.22180986129563,
-2.49423832903335));
#75860=CARTESIAN_POINT('Ctrl Pts',(-15.4716124964911,-1.30027644702517,
-5.18928239612476));
#75861=CARTESIAN_POINT('Ctrl Pts',(-15.3523465240739,3.66081343996144,-3.90100162460633));
#75862=CARTESIAN_POINT('Ctrl Pts',(-15.2330805516567,5.26134075862523,0.968330387076498));
#75863=CARTESIAN_POINT('Ctrl Pts',(-15.1138145792395,2.03204885203783,4.94875210508029));
#75864=CARTESIAN_POINT('Ctrl Pts',(-14.9960565068663,-2.99821549744162,
4.39341674690176));
#75865=CARTESIAN_POINT('Ctrl Pts',(-14.9180537586321,-4.52637808763146,
1.44204681706245));
#75866=CARTESIAN_POINT('Ctrl Pts',(-14.8798063345369,-4.53091903216787,
-0.00105619164529849));
#75867=CARTESIAN_POINT('Ctrl Pts',(-15.4819936654631,-4.5312138402642,-0.000120197794654437));
#75868=CARTESIAN_POINT('Ctrl Pts',(-15.4818242786339,-4.53121632572514,
-0.00651016932136081));
#75869=CARTESIAN_POINT('Ctrl Pts',(-15.4418995676657,-4.52830675455073,
-1.51263300533729));
#75870=CARTESIAN_POINT('Ctrl Pts',(-15.3622195325584,-2.87505846220515,
-4.51147531916218));
#75871=CARTESIAN_POINT('Ctrl Pts',(-15.2429535601412,2.2387956178267,-4.85872047690402));
#75872=CARTESIAN_POINT('Ctrl Pts',(-15.1236875877241,5.29747440746447,-0.745745015197441));
#75873=CARTESIAN_POINT('Ctrl Pts',(-15.0044216153069,3.49316406084406,4.05181138485548));
#75874=CARTESIAN_POINT('Ctrl Pts',(-14.8851556428897,-1.51780995936451,
5.1298755888585));
#75875=CARTESIAN_POINT('Ctrl Pts',(-14.7943463262751,-4.27229562126168,
2.36517103447762));
#75876=CARTESIAN_POINT('Ctrl Pts',(-14.7432923337996,-4.52511715899487,
0.43264547282851));
#75877=CARTESIAN_POINT('Ctrl Pts',(-14.7319936654631,-4.521456298353,0.00402490267532758));
#75878=CARTESIAN_POINT('Origin',(-19.0048063345371,0.,0.));
#75879=CARTESIAN_POINT('',(-16.379806334537,-4.51785206555557,0.00265012365101876));
#75880=CARTESIAN_POINT('',(-16.2319936654631,-4.52109632398741,-0.0039620509408117));
#75881=CARTESIAN_POINT('',(-19.0048063345371,-4.52375,5.14627461305311E-12));
#75882=CARTESIAN_POINT('Ctrl Pts',(-16.379806334537,-4.51785206555557,0.00265012365101888));
#75883=CARTESIAN_POINT('Ctrl Pts',(-16.3553623241617,-4.51290234764468,
-0.926504029521305));
#75884=CARTESIAN_POINT('Ctrl Pts',(-16.2911629896474,-3.78099521940542,
-3.37397142963533));
#75885=CARTESIAN_POINT('Ctrl Pts',(-16.187208330994,0.228419052524531,-5.34483459461538));
#75886=CARTESIAN_POINT('Ctrl Pts',(-16.0679423585769,4.61866000512981,-2.69949887735067));
#75887=CARTESIAN_POINT('Ctrl Pts',(-15.9486763861597,4.76906677072755,2.42391962238011));
#75888=CARTESIAN_POINT('Ctrl Pts',(-15.8294104137425,0.541545441910157,
5.32222750447519));
#75889=CARTESIAN_POINT('Ctrl Pts',(-15.723120396535,-3.66906666373755,3.55104739187141));
#75890=CARTESIAN_POINT('Ctrl Pts',(-15.6565857034664,-4.51218176763232,
1.01324106700467));
#75891=CARTESIAN_POINT('Ctrl Pts',(-15.6298063345369,-4.51976043794902,
-0.00361086820214504));
#75892=CARTESIAN_POINT('Ctrl Pts',(-16.2319936654631,-4.52109632398741,
-0.00396205094081122));
#75893=CARTESIAN_POINT('Ctrl Pts',(-16.2203562234682,-4.52478620761938,
-0.445522898085508));
#75894=CARTESIAN_POINT('Ctrl Pts',(-16.1689634573343,-4.26236780789856,
-2.39123315065092));
#75895=CARTESIAN_POINT('Ctrl Pts',(-16.0778153670614,-1.47407708230512,
-5.14261359698791));
#75896=CARTESIAN_POINT('Ctrl Pts',(-15.9585493946442,3.52753486740744,-4.02192246785722));
#75897=CARTESIAN_POINT('Ctrl Pts',(-15.839283422227,5.29093324565558,0.790821500180201));
#75898=CARTESIAN_POINT('Ctrl Pts',(-15.7200174498099,2.197346173644,4.87760609314791));
#75899=CARTESIAN_POINT('Ctrl Pts',(-15.6009208642219,-2.90610737191627,
4.48738784408032));
#75900=CARTESIAN_POINT('Ctrl Pts',(-15.5215796027729,-4.53063298458979,
1.49322502577473));
#75901=CARTESIAN_POINT('Ctrl Pts',(-15.4819936654631,-4.5312138402642,-0.000120197794654437));
#75902=CARTESIAN_POINT('Origin',(-19.0048063345371,0.,0.));
#75903=CARTESIAN_POINT('',(-17.129806334537,-4.52905226269683,0.00222857838524445));
#75904=CARTESIAN_POINT('',(-16.9819936654631,-4.51703452062264,0.00191132365274405));
#75905=CARTESIAN_POINT('',(-19.0048063345371,-4.52375,5.14627461305311E-12));
#75906=CARTESIAN_POINT('Ctrl Pts',(-17.129806334537,-4.52905226269683,0.0022285783852446));
#75907=CARTESIAN_POINT('Ctrl Pts',(-17.093894268996,-4.51989244089427,-1.35398501844981));
#75908=CARTESIAN_POINT('Ctrl Pts',(-17.018226879316,-3.1525253686288,-4.22635735705538));
#75909=CARTESIAN_POINT('Ctrl Pts',(-16.902804165497,1.73863948785637,-5.05968774485838));
#75910=CARTESIAN_POINT('Ctrl Pts',(-16.7835381930798,5.19527552722027,-1.27515938975536));
#75911=CARTESIAN_POINT('Ctrl Pts',(-16.6642722206627,3.88345012932081,3.67946867571279));
#75912=CARTESIAN_POINT('Ctrl Pts',(-16.5450062482455,-0.993689040191803,
5.25665841728971));
#75913=CARTESIAN_POINT('Ctrl Pts',(-16.4501842862036,-4.14585089210754,
2.67398054345583));
#75914=CARTESIAN_POINT('Ctrl Pts',(-16.3951176483008,-4.52095248495535,
0.584656535682572));
#75915=CARTESIAN_POINT('Ctrl Pts',(-16.379806334537,-4.51785206555557,0.00265012365101888));
#75916=CARTESIAN_POINT('Ctrl Pts',(-16.9819936654631,-4.51703452062264,
0.00191132365274384));
#75917=CARTESIAN_POINT('Ctrl Pts',(-16.9588881683026,-4.51364627034173,
-0.876727737145359));
#75918=CARTESIAN_POINT('Ctrl Pts',(-16.896027347003,-3.84165527310814,-3.27192923320261));
#75919=CARTESIAN_POINT('Ctrl Pts',(-16.7934112015644,0.0485614395649859,
-5.3495343788269));
#75920=CARTESIAN_POINT('Ctrl Pts',(-16.6741452291472,4.52523009731703,-2.85329470276329));
#75921=CARTESIAN_POINT('Ctrl Pts',(-16.5548792567301,4.84790632702384,2.26213327989446));
#75922=CARTESIAN_POINT('Ctrl Pts',(-16.4356132843129,0.720241778271576,
5.30100788941611));
#75923=CARTESIAN_POINT('Ctrl Pts',(-16.3279847538905,-3.60129660722932,
3.65193354570378));
#75924=CARTESIAN_POINT('Ctrl Pts',(-16.2601115476073,-4.51218098734078,
1.06291809892601));
#75925=CARTESIAN_POINT('Ctrl Pts',(-16.2319936654631,-4.52109632398741,
-0.00396205094081122));
#75926=CARTESIAN_POINT('Origin',(38.546,1.12989188470299E-15,0.));
#75927=CARTESIAN_POINT('',(38.546,4.53891924175741,1.9850259738362));
#75928=CARTESIAN_POINT('Ctrl Pts',(38.546,-0.439158351705697,-4.5083570246951));
#75929=CARTESIAN_POINT('Ctrl Pts',(38.546,-0.315853056119089,-4.52699458320461));
#75930=CARTESIAN_POINT('Ctrl Pts',(38.546,-0.192031275270563,-4.54020498535423));
#75931=CARTESIAN_POINT('Ctrl Pts',(38.546,-0.0679863494789869,-4.54781023322234));
#75932=CARTESIAN_POINT('Ctrl Pts',(38.546,0.0658300049648387,-4.55601457159295));
#75933=CARTESIAN_POINT('Ctrl Pts',(38.546,0.199906495945809,-4.55769712636147));
#75934=CARTESIAN_POINT('Ctrl Pts',(38.546,0.333895251847595,-4.55311715047026));
#75935=CARTESIAN_POINT('Ctrl Pts',(38.546,0.421702187996495,-4.55011575197278));
#75936=CARTESIAN_POINT('Ctrl Pts',(38.546,0.509471668919712,-4.54442374836765));
#75937=CARTESIAN_POINT('Ctrl Pts',(38.546,0.597106546689854,-4.53610218299441));
#75938=CARTESIAN_POINT('Ctrl Pts',(38.546,0.633311340086029,-4.53266427604758));
#75939=CARTESIAN_POINT('Ctrl Pts',(38.546,0.669493157857147,-4.52877745241455));
#75940=CARTESIAN_POINT('Ctrl Pts',(38.546,0.705645122236047,-4.52444556954959));
#75941=CARTESIAN_POINT('Ctrl Pts',(38.546,0.735430140612607,-4.52087660136336));
#75942=CARTESIAN_POINT('Ctrl Pts',(38.546,0.765199499756815,-4.51700477895578));
#75943=CARTESIAN_POINT('Ctrl Pts',(38.546,0.794920189293162,-4.5128365307021));
#75944=CARTESIAN_POINT('Ctrl Pts',(38.546,0.929985258158801,-4.49389401132535));
#75945=CARTESIAN_POINT('Ctrl Pts',(38.546,1.06415017772404,-4.46882312852544));
#75946=CARTESIAN_POINT('Ctrl Pts',(38.546,1.19705809126121,-4.43789314039624));
#75947=CARTESIAN_POINT('Ctrl Pts',(38.546,1.33345806832171,-4.4061504882168));
#75948=CARTESIAN_POINT('Ctrl Pts',(38.546,1.46853485839017,-4.3682367144278));
#75949=CARTESIAN_POINT('Ctrl Pts',(38.546,1.60190114888884,-4.32438793860729));
#75950=CARTESIAN_POINT('Ctrl Pts',(38.546,1.66024890098201,-4.30520409918582));
#75951=CARTESIAN_POINT('Ctrl Pts',(38.546,1.71826916481067,-4.28488357481551));
#75952=CARTESIAN_POINT('Ctrl Pts',(38.546,1.77592884056993,-4.26344303157349));
#75953=CARTESIAN_POINT('Ctrl Pts',(38.546,1.8222598517875,-4.24621501153391));
#75954=CARTESIAN_POINT('Ctrl Pts',(38.546,1.8683580417243,-4.22826381145395));
#75955=CARTESIAN_POINT('Ctrl Pts',(38.546,1.91420593282979,-4.20959724038542));
#75956=CARTESIAN_POINT('Ctrl Pts',(38.546,1.93303706195004,-4.2019303095507));
#75957=CARTESIAN_POINT('Ctrl Pts',(38.546,1.95181787751382,-4.19414596487753));
#75958=CARTESIAN_POINT('Ctrl Pts',(38.546,1.97054439427792,-4.18624627462939));
#75959=CARTESIAN_POINT('Ctrl Pts',(38.546,2.10072143930887,-4.1313317197169));
#75960=CARTESIAN_POINT('Ctrl Pts',(38.546,2.22831997826692,-4.07082932523913));
#75961=CARTESIAN_POINT('Ctrl Pts',(38.546,2.35296605824652,-4.00501001895691));
#75962=CARTESIAN_POINT('Ctrl Pts',(38.546,2.47876377876209,-3.9385825894094));
#75963=CARTESIAN_POINT('Ctrl Pts',(38.546,2.60155501516022,-3.86673927649386));
#75964=CARTESIAN_POINT('Ctrl Pts',(38.546,2.72094480205364,-3.78970660262367));
#75965=CARTESIAN_POINT('Ctrl Pts',(38.546,2.84027235032137,-3.71271408635724));
#75966=CARTESIAN_POINT('Ctrl Pts',(38.546,2.95620277917153,-3.63053727474296));
#75967=CARTESIAN_POINT('Ctrl Pts',(38.546,3.06831947638516,-3.54335537619024));
#75968=CARTESIAN_POINT('Ctrl Pts',(38.546,3.15240699929538,-3.47796895227571));
#75969=CARTESIAN_POINT('Ctrl Pts',(38.546,3.2343489187559,-3.40976617475385));
#75970=CARTESIAN_POINT('Ctrl Pts',(38.546,3.31395719113316,-3.33880703264479));
#75971=CARTESIAN_POINT('Ctrl Pts',(38.546,3.34819221866253,-3.30829150817704));
#75972=CARTESIAN_POINT('Ctrl Pts',(38.546,3.38199551452986,-3.27726606885898));
#75973=CARTESIAN_POINT('Ctrl Pts',(38.546,3.41535137166061,-3.24573478649975));
#75974=CARTESIAN_POINT('Ctrl Pts',(38.546,3.43218348133969,-3.22982339795673));
#75975=CARTESIAN_POINT('Ctrl Pts',(38.546,3.44890367494083,-3.21378110636634));
#75976=CARTESIAN_POINT('Ctrl Pts',(38.546,3.46549235688335,-3.19762579924582));
#75977=CARTESIAN_POINT('Ctrl Pts',(38.546,3.56835841884713,-3.09744708528517));
#75978=CARTESIAN_POINT('Ctrl Pts',(38.546,3.66631150069133,-2.99279463917215));
#75979=CARTESIAN_POINT('Ctrl Pts',(38.546,3.75896065749294,-2.88389381695821));
#75980=CARTESIAN_POINT('Ctrl Pts',(38.546,3.82831127839855,-2.80237834613921));
#75981=CARTESIAN_POINT('Ctrl Pts',(38.546,3.89468982964041,-2.71848149692477));
#75982=CARTESIAN_POINT('Ctrl Pts',(38.546,3.95792179330259,-2.63228181070258));
#75983=CARTESIAN_POINT('Ctrl Pts',(38.546,4.04051693559048,-2.51968566570969));
#75984=CARTESIAN_POINT('Ctrl Pts',(38.546,4.11774512193109,-2.40316146256433));
#75985=CARTESIAN_POINT('Ctrl Pts',(38.546,4.18956529902346,-2.28317878216882));
#75986=CARTESIAN_POINT('Ctrl Pts',(38.546,4.2623473162119,-2.1615892531479));
#75987=CARTESIAN_POINT('Ctrl Pts',(38.546,4.32957582585562,-2.03644727806392));
#75988=CARTESIAN_POINT('Ctrl Pts',(38.546,4.39116358165225,-1.9082119883273));
#75989=CARTESIAN_POINT('Ctrl Pts',(38.546,4.40867475231375,-1.87175100652405));
#75990=CARTESIAN_POINT('Ctrl Pts',(38.546,4.42572961893407,-1.83503980875703));
#75991=CARTESIAN_POINT('Ctrl Pts',(38.546,4.44232547369155,-1.79808864718056));
#75992=CARTESIAN_POINT('Ctrl Pts',(38.546,4.45192170739655,-1.77672234894881));
#75993=CARTESIAN_POINT('Ctrl Pts',(38.546,4.46136446421361,-1.75527581657772));
#75994=CARTESIAN_POINT('Ctrl Pts',(38.546,4.4706531714735,-1.73375101734231));
#75995=CARTESIAN_POINT('Ctrl Pts',(38.546,4.47839968625891,-1.71579995366198));
#75996=CARTESIAN_POINT('Ctrl Pts',(38.546,4.48603931914584,-1.69779368007736));
#75997=CARTESIAN_POINT('Ctrl Pts',(38.546,4.49356556988639,-1.67974851790699));
#75998=CARTESIAN_POINT('Ctrl Pts',(38.546,4.54834464674398,-1.54840857727591));
#75999=CARTESIAN_POINT('Ctrl Pts',(38.546,4.59720230371699,-1.41482472346982));
#76000=CARTESIAN_POINT('Ctrl Pts',(38.546,4.64012638128586,-1.27949345669834));
#76001=CARTESIAN_POINT('Ctrl Pts',(38.546,4.68454708660772,-1.13944361375309));
#76002=CARTESIAN_POINT('Ctrl Pts',(38.546,4.72261371185113,-0.997521695858663));
#76003=CARTESIAN_POINT('Ctrl Pts',(38.546,4.75426513105171,-0.854245649721898));
#76004=CARTESIAN_POINT('Ctrl Pts',(38.546,4.78591655025229,-0.710969603585134));
#76005=CARTESIAN_POINT('Ctrl Pts',(38.546,4.81115300645672,-0.566338522023502));
#76006=CARTESIAN_POINT('Ctrl Pts',(38.546,4.82986142094086,-0.420850963889773));
#76007=CARTESIAN_POINT('Ctrl Pts',(38.546,4.84288525531898,-0.319570020877905));
#76008=CARTESIAN_POINT('Ctrl Pts',(38.546,4.85274434453973,-0.217873614789138));
#76009=CARTESIAN_POINT('Ctrl Pts',(38.546,4.85943963746551,-0.115893038039486));
#76010=CARTESIAN_POINT('Ctrl Pts',(38.546,4.86237760912286,-0.071142786271284));
#76011=CARTESIAN_POINT('Ctrl Pts',(38.546,4.86470620625745,-0.0263378083986588));
#76012=CARTESIAN_POINT('Ctrl Pts',(38.546,4.86642471852824,0.0185107941749964));
#76013=CARTESIAN_POINT('Ctrl Pts',(38.546,4.8673843344193,0.0435542183347263));
#76014=CARTESIAN_POINT('Ctrl Pts',(38.546,4.86815371130291,0.0686112446241784));
#76015=CARTESIAN_POINT('Ctrl Pts',(38.546,4.86873265976743,0.0936799341927062));
#76016=CARTESIAN_POINT('Ctrl Pts',(38.546,4.86919802311952,0.113830345023657));
#76017=CARTESIAN_POINT('Ctrl Pts',(38.546,4.86954030391283,0.13398943210598));
#76018=CARTESIAN_POINT('Ctrl Pts',(38.546,4.86975936328296,0.154138793044496));
#76019=CARTESIAN_POINT('Ctrl Pts',(38.546,4.87134037559417,0.299562326800043));
#76020=CARTESIAN_POINT('Ctrl Pts',(38.546,4.86651295009269,0.44468557075459));
#76021=CARTESIAN_POINT('Ctrl Pts',(38.546,4.85537168171244,0.589123037842825));
#76022=CARTESIAN_POINT('Ctrl Pts',(38.546,4.84413015250928,0.734860304811507));
#76023=CARTESIAN_POINT('Ctrl Pts',(38.546,4.82646070429186,0.879900105190756));
#76024=CARTESIAN_POINT('Ctrl Pts',(38.546,4.80240862941678,1.02385544469749));
#76025=CARTESIAN_POINT('Ctrl Pts',(38.546,4.7784458282956,1.16727646716007));
#76026=CARTESIAN_POINT('Ctrl Pts',(38.546,4.74814767146142,1.30962178718956));
#76027=CARTESIAN_POINT('Ctrl Pts',(38.546,4.7115074706548,1.45050682382756));
#76028=CARTESIAN_POINT('Ctrl Pts',(38.546,4.67545543043744,1.58913032738593));
#76029=CARTESIAN_POINT('Ctrl Pts',(38.546,4.63326321279241,1.72634071218179));
#76030=CARTESIAN_POINT('Ctrl Pts',(38.546,4.5848756392546,1.8617596047089));
#76031=CARTESIAN_POINT('Ctrl Pts',(38.546,4.57013310101999,1.90301850766277));
#76032=CARTESIAN_POINT('Ctrl Pts',(38.546,4.55481512189451,1.94411098781377));
#76033=CARTESIAN_POINT('Ctrl Pts',(38.546,4.53891924175741,1.9850259738362));
#76034=CARTESIAN_POINT('',(38.546,-4.954,-6.06690024297599E-16));
#76035=CARTESIAN_POINT('Origin',(38.546,0.,0.));
#76036=CARTESIAN_POINT('',(38.546,1.34632304271355,4.77431539461067));
#76037=CARTESIAN_POINT('Origin',(38.546,0.,0.));
#76038=CARTESIAN_POINT('Ctrl Pts',(38.546,1.34632304271247,4.77431539461098));
#76039=CARTESIAN_POINT('Ctrl Pts',(38.546,1.21424233318388,4.80662176345812));
#76040=CARTESIAN_POINT('Ctrl Pts',(38.546,1.08105150480208,4.83309789730618));
#76041=CARTESIAN_POINT('Ctrl Pts',(38.546,0.947020732932665,4.85348970562246));
#76042=CARTESIAN_POINT('Ctrl Pts',(38.546,0.803943619664192,4.87525784906835));
#76043=CARTESIAN_POINT('Ctrl Pts',(38.546,0.659908771978632,4.89009318781608));
#76044=CARTESIAN_POINT('Ctrl Pts',(38.546,0.515330126718157,4.89819217175583));
#76045=CARTESIAN_POINT('Ctrl Pts',(38.546,0.424258338069233,4.90329381696977));
#76046=CARTESIAN_POINT('Ctrl Pts',(38.546,0.332970701700517,4.90572146609836));
#76047=CARTESIAN_POINT('Ctrl Pts',(38.546,0.241571546653192,4.9055137924178));
#76048=CARTESIAN_POINT('Ctrl Pts',(38.546,0.187651338017814,4.90539127697246));
#76049=CARTESIAN_POINT('Ctrl Pts',(38.546,0.133692339195287,4.9043514370587));
#76050=CARTESIAN_POINT('Ctrl Pts',(38.546,0.0797162708863841,4.90240097324179));
#76051=CARTESIAN_POINT('Ctrl Pts',(38.546,0.0592483719030999,4.90166135107912));
#76052=CARTESIAN_POINT('Ctrl Pts',(38.546,0.0387799975818231,4.90079080921751));
#76053=CARTESIAN_POINT('Ctrl Pts',(38.546,0.0183214479839144,4.89979031654226));
#76054=CARTESIAN_POINT('Ctrl Pts',(38.546,-0.126232375798732,4.89272114278774));
#76055=CARTESIAN_POINT('Ctrl Pts',(38.546,-0.270424963023004,4.87916423615376));
#76056=CARTESIAN_POINT('Ctrl Pts',(38.546,-0.413845925691374,4.85932065155221));
#76057=CARTESIAN_POINT('Ctrl Pts',(38.546,-0.556818723029428,4.83953907466893));
#76058=CARTESIAN_POINT('Ctrl Pts',(38.546,-0.699025445885051,4.81350970909549));
#76059=CARTESIAN_POINT('Ctrl Pts',(38.546,-0.840049999303419,4.78138245765063));
#76060=CARTESIAN_POINT('Ctrl Pts',(38.546,-0.903801000427365,4.76685913959484));
#76061=CARTESIAN_POINT('Ctrl Pts',(38.546,-0.967310223053341,4.75108905211055));
#76062=CARTESIAN_POINT('Ctrl Pts',(38.546,-1.03053797068624,4.73408300031222));
#76063=CARTESIAN_POINT('Ctrl Pts',(38.546,-1.06559199633794,4.72465469393898));
#76064=CARTESIAN_POINT('Ctrl Pts',(38.546,-1.10055948881135,4.71484645759226));
#76065=CARTESIAN_POINT('Ctrl Pts',(38.546,-1.13543354587295,4.70465989520712));
#76066=CARTESIAN_POINT('Ctrl Pts',(38.546,-1.1551184438112,4.69891002100868));
#76067=CARTESIAN_POINT('Ctrl Pts',(38.546,-1.17477357027183,4.69303960478021));
#76068=CARTESIAN_POINT('Ctrl Pts',(38.546,-1.19439766842355,4.68704891182773));
#76069=CARTESIAN_POINT('Ctrl Pts',(38.546,-1.2137571243417,4.68113900681013));
#76070=CARTESIAN_POINT('Ctrl Pts',(38.546,-1.23307759653258,4.67511472144436));
#76071=CARTESIAN_POINT('Ctrl Pts',(38.546,-1.25235612728143,4.66897721777225));
#76072=CARTESIAN_POINT('Ctrl Pts',(38.546,-1.39105596230319,4.62482080575842));
#76073=CARTESIAN_POINT('Ctrl Pts',(38.546,-1.5276178035149,4.57479853248734));
#76074=CARTESIAN_POINT('Ctrl Pts',(38.546,-1.66163493395825,4.51909969878119));
#76075=CARTESIAN_POINT('Ctrl Pts',(38.546,-1.79558046144293,4.46343062396687));
#76076=CARTESIAN_POINT('Ctrl Pts',(38.546,-1.92698476075658,4.40209070867796));
#76077=CARTESIAN_POINT('Ctrl Pts',(38.546,-2.05542255410814,4.33522083355556));
#76078=CARTESIAN_POINT('Ctrl Pts',(38.546,-2.18368858884634,4.26844038286756));
#76079=CARTESIAN_POINT('Ctrl Pts',(38.546,-2.30899679754021,4.19614442386914));
#76080=CARTESIAN_POINT('Ctrl Pts',(38.546,-2.43089310525813,4.11843031770512));
#76081=CARTESIAN_POINT('Ctrl Pts',(38.546,-2.52231533604658,4.0601447380821));
#76082=CARTESIAN_POINT('Ctrl Pts',(38.546,-2.61181781860713,3.99881054397038));
#76083=CARTESIAN_POINT('Ctrl Pts',(38.546,-2.69919385199506,3.93445456336783));
#76084=CARTESIAN_POINT('Ctrl Pts',(38.546,-2.7345326321001,3.90842612331654));
#76085=CARTESIAN_POINT('Ctrl Pts',(38.546,-2.76952341085071,3.88190326087209));
#76086=CARTESIAN_POINT('Ctrl Pts',(38.546,-2.80415179400507,3.85488722970614));
#76087=CARTESIAN_POINT('Ctrl Pts',(38.546,-2.81829779538271,3.84385094157254));
#76088=CARTESIAN_POINT('Ctrl Pts',(38.546,-2.83238385045348,3.83273192268361));
#76089=CARTESIAN_POINT('Ctrl Pts',(38.546,-2.84640731961621,3.82153155251358));
#76090=CARTESIAN_POINT('Ctrl Pts',(38.546,-2.95689883089296,3.73328335853356));
#76091=CARTESIAN_POINT('Ctrl Pts',(38.546,-3.06309443210339,3.64031882545039));
#76092=CARTESIAN_POINT('Ctrl Pts',(38.546,-3.16460343412711,3.54276990989711));
#76093=CARTESIAN_POINT('Ctrl Pts',(38.546,-3.25260642961082,3.45820010225709));
#76094=CARTESIAN_POINT('Ctrl Pts',(38.546,-3.33708685923698,3.37018388722644));
#76095=CARTESIAN_POINT('Ctrl Pts',(38.546,-3.41776880234159,3.27878373378786));
#76096=CARTESIAN_POINT('Ctrl Pts',(38.546,-3.51096857413409,3.17320281797835));
#76097=CARTESIAN_POINT('Ctrl Pts',(38.546,-3.59910092973385,3.06310654550583));
#76098=CARTESIAN_POINT('Ctrl Pts',(38.546,-3.68202759143973,2.94896297151972));
#76099=CARTESIAN_POINT('Ctrl Pts',(38.546,-3.76531917476244,2.83431710482445));
#76100=CARTESIAN_POINT('Ctrl Pts',(38.546,-3.84335944226955,2.71558740333836));
#76101=CARTESIAN_POINT('Ctrl Pts',(38.546,-3.91596031882729,2.59322728048773));
#76102=CARTESIAN_POINT('Ctrl Pts',(38.546,-3.93941378432771,2.55369926022173));
#76103=CARTESIAN_POINT('Ctrl Pts',(38.546,-3.96229920896436,2.5137922632784));
#76104=CARTESIAN_POINT('Ctrl Pts',(38.546,-3.9846091093253,2.47352133654474));
#76105=CARTESIAN_POINT('Ctrl Pts',(38.546,-3.9934143104391,2.45762733418739));
#76106=CARTESIAN_POINT('Ctrl Pts',(38.546,-4.0021298559497,2.44167664182989));
#76107=CARTESIAN_POINT('Ctrl Pts',(38.546,-4.01075526095843,2.42567018232057));
#76108=CARTESIAN_POINT('Ctrl Pts',(38.546,-4.01985169352743,2.40878962083419));
#76109=CARTESIAN_POINT('Ctrl Pts',(38.546,-4.02884402453685,2.39185413189062));
#76110=CARTESIAN_POINT('Ctrl Pts',(38.546,-4.03772966494529,2.37486939831507));
#76111=CARTESIAN_POINT('Ctrl Pts',(38.546,-4.10267026727469,2.25073666526475));
#76112=CARTESIAN_POINT('Ctrl Pts',(38.546,-4.16195655546587,2.12390033921895));
#76113=CARTESIAN_POINT('Ctrl Pts',(38.546,-4.21548626120384,1.99483096966602));
#76114=CARTESIAN_POINT('Ctrl Pts',(38.546,-4.26923983167619,1.86522182355849));
#76115=CARTESIAN_POINT('Ctrl Pts',(38.546,-4.31718883006406,1.73336008190174));
#76116=CARTESIAN_POINT('Ctrl Pts',(38.546,-4.35918181423245,1.59970128041928));
#76117=CARTESIAN_POINT('Ctrl Pts',(38.546,-4.39954043011255,1.47124448376979));
#76118=CARTESIAN_POINT('Ctrl Pts',(38.546,-4.43439753246674,1.34112700894506));
#76119=CARTESIAN_POINT('Ctrl Pts',(38.546,-4.46357390460294,1.20974588256244));
#76120=CARTESIAN_POINT('Ctrl Pts',(38.546,-4.48425134443962,1.11663542579388));
#76121=CARTESIAN_POINT('Ctrl Pts',(38.546,-4.50207458172136,1.02289014857479));
#76122=CARTESIAN_POINT('Ctrl Pts',(38.546,-4.51701982161582,0.928629909937474));
#76123=CARTESIAN_POINT('Ctrl Pts',(38.546,-4.52402075405636,0.884474742995445));
#76124=CARTESIAN_POINT('Ctrl Pts',(38.546,-4.53038999373665,0.8402065928306));
#76125=CARTESIAN_POINT('Ctrl Pts',(38.546,-4.53612425080577,0.795837921409192));
#76126=CARTESIAN_POINT('Ctrl Pts',(38.546,-4.53952194720462,0.769548330047427));
#76127=CARTESIAN_POINT('Ctrl Pts',(38.546,-4.54269669918852,0.743223449100096));
#76128=CARTESIAN_POINT('Ctrl Pts',(38.546,-4.54564773289263,0.716865893342667));
#76129=CARTESIAN_POINT('Ctrl Pts',(38.546,-4.54745751221922,0.700701605065332));
#76130=CARTESIAN_POINT('Ctrl Pts',(38.546,-4.54918297077606,0.684526320540122));
#76131=CARTESIAN_POINT('Ctrl Pts',(38.546,-4.55082307057052,0.668350423530228));
#76132=CARTESIAN_POINT('Ctrl Pts',(38.546,-4.56547759744107,0.52381646395733));
#76133=CARTESIAN_POINT('Ctrl Pts',(38.546,-4.57334695024406,0.379020687625459));
#76134=CARTESIAN_POINT('Ctrl Pts',(38.546,-4.57444969521142,0.234390006360559));
#76135=CARTESIAN_POINT('Ctrl Pts',(38.546,-4.57549951960631,0.0967001307002065));
#76136=CARTESIAN_POINT('Ctrl Pts',(38.546,-4.57041614699662,-0.0408408986859376));
#76137=CARTESIAN_POINT('Ctrl Pts',(38.546,-4.55916271844398,-0.177865018424011));
#76138=CARTESIAN_POINT('Ctrl Pts',(38.546,-4.5480089654111,-0.313675468008928));
#76139=CARTESIAN_POINT('Ctrl Pts',(38.546,-4.53079389772483,-0.448978801903289));
#76140=CARTESIAN_POINT('Ctrl Pts',(38.546,-4.50743176272214,-0.583406337128876));
#76141=CARTESIAN_POINT('Ctrl Pts',(38.546,-4.48453671791127,-0.715146199194071));
#76142=CARTESIAN_POINT('Ctrl Pts',(38.546,-4.45573780575909,-0.846045505627378));
#76143=CARTESIAN_POINT('Ctrl Pts',(38.546,-4.42090797245811,-0.97573816109587));
#76144=CARTESIAN_POINT('Ctrl Pts',(38.546,-4.41413948486699,-1.00094135749399));
#76145=CARTESIAN_POINT('Ctrl Pts',(38.546,-4.407143104959,-1.02609891192132));
#76146=CARTESIAN_POINT('Ctrl Pts',(38.546,-4.39991769847472,-1.05120802372743));
#76147=CARTESIAN_POINT('Ctrl Pts',(-17.8668049533188,-1.93258782773145,
4.09016116438023));
#76148=CARTESIAN_POINT('Ctrl Pts',(-17.8469272912493,-2.61370891938372,
3.76833366711637));
#76149=CARTESIAN_POINT('Ctrl Pts',(-17.8071719671103,-3.80128785052217,
2.77774777382202));
#76150=CARTESIAN_POINT('Ctrl Pts',(-17.7276613188322,-4.98891923544753,
-0.109469461415501));
#76151=CARTESIAN_POINT('Ctrl Pts',(-17.6282730084845,-3.45849333686121,
-4.08082754129702));
#76152=CARTESIAN_POINT('Ctrl Pts',(-17.5090070360674,1.56940258829812,-5.11725866595573));
#76153=CARTESIAN_POINT('Ctrl Pts',(-17.3897410636502,5.14844039432527,-1.44815814548532));
#76154=CARTESIAN_POINT('Ctrl Pts',(-17.270475091233,4.00553813139823,3.54623540470151));
#76155=CARTESIAN_POINT('Ctrl Pts',(-17.1512091188158,-0.816602122674766,
5.28738771244033));
#76156=CARTESIAN_POINT('Ctrl Pts',(-17.0319431463987,-4.88794592317846,
2.17368458761069));
#76157=CARTESIAN_POINT('Ctrl Pts',(-16.9126771739815,-4.47285648319269,
-2.93483056265198));
#76158=CARTESIAN_POINT('Ctrl Pts',(-16.7934112015644,0.0485614395649859,
-5.3495343788269));
#76159=CARTESIAN_POINT('Ctrl Pts',(-16.6741452291472,4.52523009731703,-2.85329470276329));
#76160=CARTESIAN_POINT('Ctrl Pts',(-16.5548792567301,4.84790632702384,2.26213327989446));
#76161=CARTESIAN_POINT('Ctrl Pts',(-16.4356132843129,0.720241778271576,
5.30100788941611));
#76162=CARTESIAN_POINT('Ctrl Pts',(-16.3163473118957,-4.06856724720163,
3.47362574065601));
#76163=CARTESIAN_POINT('Ctrl Pts',(-16.1970813394785,-5.12251561539824,
-1.54247163636852));
#76164=CARTESIAN_POINT('Ctrl Pts',(-16.0778153670614,-1.47407708230512,
-5.14261359698791));
#76165=CARTESIAN_POINT('Ctrl Pts',(-15.9585493946442,3.52753486740744,-4.02192246785722));
#76166=CARTESIAN_POINT('Ctrl Pts',(-15.839283422227,5.29093324565558,0.790821500180201));
#76167=CARTESIAN_POINT('Ctrl Pts',(-15.7200174498099,2.197346173644,4.87760609314791));
#76168=CARTESIAN_POINT('Ctrl Pts',(-15.6007514773927,-2.91336583201067,
4.48683285057177));
#76169=CARTESIAN_POINT('Ctrl Pts',(-15.4814855049756,-5.34965909419724,
-0.022774426867852));
#76170=CARTESIAN_POINT('Ctrl Pts',(-15.3622195325584,-2.87505846220515,
-4.51147531916218));
#76171=CARTESIAN_POINT('Ctrl Pts',(-15.2429535601412,2.2387956178267,-4.85872047690402));
#76172=CARTESIAN_POINT('Ctrl Pts',(-15.1236875877241,5.29747440746447,-0.745745015197441));
#76173=CARTESIAN_POINT('Ctrl Pts',(-15.0044216153069,3.49316406084406,4.05181138485548));
#76174=CARTESIAN_POINT('Ctrl Pts',(-14.8851556428897,-1.51780995936451,
5.1298755888585));
#76175=CARTESIAN_POINT('Ctrl Pts',(-14.7658896704726,-5.13546091438147,
1.49880347624965));
#76176=CARTESIAN_POINT('Ctrl Pts',(-14.6466236980554,-4.03884831250948,
-3.50814409050182));
#76177=CARTESIAN_POINT('Ctrl Pts',(-14.5273577256382,0.765356598558913,
-5.29467656481004));
#76178=CARTESIAN_POINT('Ctrl Pts',(-14.4080917532211,4.86697750131595,-2.22078829592513));
#76179=CARTESIAN_POINT('Ctrl Pts',(-14.2888257808039,4.50079794053571,2.89174489712377));
#76180=CARTESIAN_POINT('Ctrl Pts',(-14.1695598083868,0.00296436731219236,
5.34970670821892));
#76181=CARTESIAN_POINT('Ctrl Pts',(-14.0502938359696,-4.49759044353025,
2.89673106351802));
#76182=CARTESIAN_POINT('Ctrl Pts',(-13.9310278635524,-4.8694356679322,-2.21539317675726));
#76183=CARTESIAN_POINT('Ctrl Pts',(-13.8117618911353,-0.771223875207531,
-5.29382511857655));
#76184=CARTESIAN_POINT('Ctrl Pts',(-13.6924959187181,4.03495798434998,-3.51261792917751));
#76185=CARTESIAN_POINT('Ctrl Pts',(-13.5732299463009,5.13711878645237,1.49311125696483));
#76186=CARTESIAN_POINT('Ctrl Pts',(-13.4539639738838,1.52349413715743,5.12819035000159));
#76187=CARTESIAN_POINT('Ctrl Pts',(-13.3346980014666,-3.48867155936125,
4.0556801405828));
#76188=CARTESIAN_POINT('Ctrl Pts',(-13.2154320290494,-5.29829760899626,
-0.73987370429712));
#76189=CARTESIAN_POINT('Ctrl Pts',(-13.0961660566323,-2.24417885919362,
-4.85623639249116));
#76190=CARTESIAN_POINT('Ctrl Pts',(-12.9769000842151,2.8700569434679,-4.51465876817511));
#76191=CARTESIAN_POINT('Ctrl Pts',(-12.8576341117979,5.34963052761172,-0.0287031331433309));
#76192=CARTESIAN_POINT('Ctrl Pts',(-12.7383681393808,2.91833658830642,4.48360147751333));
#76193=CARTESIAN_POINT('Ctrl Pts',(-12.6191021669636,-2.19193944145102,
4.88003812862352));
#76194=CARTESIAN_POINT('Ctrl Pts',(-12.4998361945465,-5.29005329274958,
0.796684888570813));
#76195=CARTESIAN_POINT('Ctrl Pts',(-12.3805702221293,-3.53199048313817,
-4.01801118450772));
#76196=CARTESIAN_POINT('Ctrl Pts',(-12.2613042497121,1.4683779898736,-5.14424306683332));
#76197=CARTESIAN_POINT('Ctrl Pts',(-12.142038277295,5.12080107761086,-1.54814953261863));
#76198=CARTESIAN_POINT('Ctrl Pts',(-12.0227723048778,4.07241808607112,3.46911827184497));
#76199=CARTESIAN_POINT('Ctrl Pts',(-11.9035063324606,-0.714373682966412,
5.30179600634471));
#76200=CARTESIAN_POINT('Ctrl Pts',(-11.7842403600435,-4.84538287016409,
2.26751747365443));
#76201=CARTESIAN_POINT('Ctrl Pts',(-11.6649743876263,-4.52841508905532,
-2.84830255292936));
#76202=CARTESIAN_POINT('Ctrl Pts',(-11.5457084152091,-0.0544412345818395,
-5.34943051209986));
#76203=CARTESIAN_POINT('Ctrl Pts',(-11.4264424427919,4.46950872374863,-2.93987455857264));
#76204=CARTESIAN_POINT('Ctrl Pts',(-11.3071764703748,4.89052762470212,2.16843496647541));
#76205=CARTESIAN_POINT('Ctrl Pts',(-11.1879104979576,0.822127460035971,
5.28615901115948));
#76206=CARTESIAN_POINT('Ctrl Pts',(-11.0686445255405,-4.00097137452672,
3.55128127751458));
#76207=CARTESIAN_POINT('Ctrl Pts',(-10.9493785531233,-5.15124826671406,
-1.44361073232473));
#76208=CARTESIAN_POINT('Ctrl Pts',(-10.8301125807061,-1.57276909104567,
-5.11329326736293));
#76209=CARTESIAN_POINT('Ctrl Pts',(-10.710846608289,3.44948468012718,-4.08906176199085));
#76210=CARTESIAN_POINT('Ctrl Pts',(-10.5915806358718,5.30517167611101,0.688857125097259));
#76211=CARTESIAN_POINT('Ctrl Pts',(-10.4723146634547,2.29080359893313,4.83441718544467));
#76212=CARTESIAN_POINT('Ctrl Pts',(-10.3530486910375,-2.82648222901952,
4.54206658480968));
#76213=CARTESIAN_POINT('Ctrl Pts',(-10.2337827186203,-5.34910666634805,
0.0801780757980781));
#76214=CARTESIAN_POINT('Ctrl Pts',(-10.1145167462031,-2.96134447573091,
-4.45531250844044));
#76215=CARTESIAN_POINT('Ctrl Pts',(-9.995250773786,2.14488029590958,-4.90090391336402));
#76216=CARTESIAN_POINT('Ctrl Pts',(-9.87598480136882,5.28214236395734,-0.847551000645274));
#76217=CARTESIAN_POINT('Ctrl Pts',(-9.75671882895166,3.57048986575489,3.98383894884689));
#76218=CARTESIAN_POINT('Ctrl Pts',(-9.6374528565345,-1.41881005763682,5.15813422393762));
#76219=CARTESIAN_POINT('Ctrl Pts',(-9.51818688411732,-5.10566709305165,
1.59735224253676));
#76220=CARTESIAN_POINT('Ctrl Pts',(-9.39892091170017,-4.10561078306872,
-3.42977123869183));
#76221=CARTESIAN_POINT('Ctrl Pts',(-9.279654939283,0.663324621354469,-5.30842454015434));
#76222=CARTESIAN_POINT('Ctrl Pts',(-9.16038896686585,4.82333959217,-2.31403669599532));
#76223=CARTESIAN_POINT('Ctrl Pts',(-9.04112299444865,4.55561293942915,2.80459647684182));
#76224=CARTESIAN_POINT('Ctrl Pts',(-8.92185702203153,0.105913061027885,
5.34865899785279));
#76225=CARTESIAN_POINT('Ctrl Pts',(-8.80259104961433,-4.44101316020701,
2.98274584278913));
#76226=CARTESIAN_POINT('Ctrl Pts',(-8.68332507719718,-4.91116675441572,
-2.12127597500409));
#76227=CARTESIAN_POINT('Ctrl Pts',(-8.56405910478001,-0.872954921887009,
-5.27800344412176));
#76228=CARTESIAN_POINT('Ctrl Pts',(-8.44479313236285,3.96661430405479,-3.58961580321287));
#76229=CARTESIAN_POINT('Ctrl Pts',(-8.32552715994568,5.16490077910572,1.39397653990334));
#76230=CARTESIAN_POINT('Ctrl Pts',(-8.20626118752853,1.62189841803372,5.09792273121));
#76231=CARTESIAN_POINT('Ctrl Pts',(-8.08699521511134,-3.40997840387161,
4.12206476622297));
#76232=CARTESIAN_POINT('Ctrl Pts',(-7.96772924269419,-5.31155452317641,
-0.637776762772118));
#76233=CARTESIAN_POINT('Ctrl Pts',(-7.84846327027703,-2.33721622703428,
-4.8121503467676));
#76234=CARTESIAN_POINT('Ctrl Pts',(-7.72919729785987,2.78264580301424,-4.56905383933861));
#76235=CARTESIAN_POINT('Ctrl Pts',(-7.60993132544269,5.34808751697683,-0.131645594550073));
#76236=CARTESIAN_POINT('Ctrl Pts',(-7.49066535302554,3.00407816434195,4.42661101005405));
#76237=CARTESIAN_POINT('Ctrl Pts',(-7.37139938060837,-2.09762255015898,
4.92131591028987));
#76238=CARTESIAN_POINT('Ctrl Pts',(-7.2521334081912,-5.27374234746165,0.898338635703456));
#76239=CARTESIAN_POINT('Ctrl Pts',(-7.13286743577404,-3.60865864715558,
-3.94929783887176));
#76240=CARTESIAN_POINT('Ctrl Pts',(-7.01360146335687,1.36911075397815,-5.17154777558412));
#76241=CARTESIAN_POINT('Ctrl Pts',(-6.89433549093971,5.09006036110679,-1.64640704933419));
#76242=CARTESIAN_POINT('Ctrl Pts',(-6.77506951852255,4.13842333057186,3.3901066338371));
#76243=CARTESIAN_POINT('Ctrl Pts',(-6.65580354610538,-0.612214140739847,
5.31456155272341));
#76244=CARTESIAN_POINT('Ctrl Pts',(-6.53653757368821,-4.80084970824945,
2.36034165548316));
#76245=CARTESIAN_POINT('Ctrl Pts',(-6.41727160127105,-4.58238897340408,
-2.76063071565767));
#76246=CARTESIAN_POINT('Ctrl Pts',(-6.29800562885389,-0.157375080700092,
-5.34739223694899));
#76247=CARTESIAN_POINT('Ctrl Pts',(-6.17873965643672,4.41210639136683,-3.02534094658233));
#76248=CARTESIAN_POINT('Ctrl Pts',(-6.05947368401956,4.93135114605077,2.07392056891087));
#76249=CARTESIAN_POINT('Ctrl Pts',(-5.94020771160239,0.923701554504711,
5.2693591726142));
#76250=CARTESIAN_POINT('Ctrl Pts',(-5.82094173918523,-3.93188995414451,
3.62761795677345));
#76251=CARTESIAN_POINT('Ctrl Pts',(-5.70167576676806,-5.17807505950615,
-1.34421327546196));
#76252=CARTESIAN_POINT('Ctrl Pts',(-5.5824097943509,-1.67087756910494,-5.08208016474257));
#76253=CARTESIAN_POINT('Ctrl Pts',(-5.46314382193374,3.37015638858599,-4.15468609744235));
#76254=CARTESIAN_POINT('Ctrl Pts',(-5.34387784951657,5.31744555918776,0.586637346988937));
#76255=CARTESIAN_POINT('Ctrl Pts',(-5.22461187709941,2.38341244602753,4.7894379382062));
#76256=CARTESIAN_POINT('Ctrl Pts',(-5.10534590468224,-2.73855172438397,
4.59561803293978));
#76257=CARTESIAN_POINT('Ctrl Pts',(-4.98607993226508,-5.34657317386386,
0.183100923884053));
#76258=CARTESIAN_POINT('Ctrl Pts',(-4.86681395984791,-3.04653369731289,
-4.39749963990275));
#76259=CARTESIAN_POINT('Ctrl Pts',(-4.74754798743075,2.05017057992043,-4.94127222939968));
#76260=CARTESIAN_POINT('Ctrl Pts',(-4.62828201501358,5.26485402104248,-0.949043091182221));
#76261=CARTESIAN_POINT('Ctrl Pts',(-4.50901604259642,3.64649329319062,3.91439105283614));
#76262=CARTESIAN_POINT('Ctrl Pts',(-4.38975007017925,-1.31928468068921,
5.18448247977621));
#76263=CARTESIAN_POINT('Ctrl Pts',(-4.27048409776209,-5.07398232684534,
1.69530941089495));
#76264=CARTESIAN_POINT('Ctrl Pts',(-4.15121812534492,-4.17085269037897,
-3.3501281299327));
#76265=CARTESIAN_POINT('Ctrl Pts',(-4.03195215292777,0.561046973578825,
-5.32020647580954));
#76266=CARTESIAN_POINT('Ctrl Pts',(-3.91268618051059,4.77791530080097,-2.40642806461773));
#76267=CARTESIAN_POINT('Ctrl Pts',(-3.79342020809343,4.60874071171544,2.71640934028442));
#76268=CARTESIAN_POINT('Ctrl Pts',(-3.67415423567627,0.208822528592261,
5.3456303466813));
#76269=CARTESIAN_POINT('Ctrl Pts',(-3.5548882632591,-4.38279109378327,3.06765592595745));
#76270=CARTESIAN_POINT('Ctrl Pts',(-3.43562229084194,-4.95107893068038,
-2.0263731329596));
#76271=CARTESIAN_POINT('Ctrl Pts',(-3.31635631842477,-0.97436265912244,
-5.26022699703307));
#76272=CARTESIAN_POINT('Ctrl Pts',(-3.19709034600761,3.89680154001646,-3.66528421947511));
#76273=CARTESIAN_POINT('Ctrl Pts',(-3.07782437359044,5.19076988807344,1.29432554671451));
#76274=CARTESIAN_POINT('Ctrl Pts',(-2.95855840117328,1.71970200914856,5.0657670348663));
#76275=CARTESIAN_POINT('Ctrl Pts',(-2.83929242875612,-3.33002232149737,
4.18692273515254));
#76276=CARTESIAN_POINT('Ctrl Pts',(-2.72002645633895,-5.32284423867826,
-0.53544361288319));
#76277=CARTESIAN_POINT('Ctrl Pts',(-2.60076048392179,-2.42938797848125,
-4.76628206276323));
#76278=CARTESIAN_POINT('Ctrl Pts',(-2.48149451150462,2.69420407591751,-4.62175670596335));
#76279=CARTESIAN_POINT('Ctrl Pts',(-2.36222853908746,5.34456377722621,-0.234539299413323));
#76280=CARTESIAN_POINT('Ctrl Pts',(-2.2429625666703,3.0887071435723,4.36798109348626));
#76281=CARTESIAN_POINT('Ctrl Pts',(-2.12369659425313,-2.00252877889888,
4.96077102288439));
#76282=CARTESIAN_POINT('Ctrl Pts',(-2.00443062183597,-5.25547820769376,
0.999659672220339));
#76283=CARTESIAN_POINT('Ctrl Pts',(-1.8851646494188,-3.68399030064885,-3.87912182285284));
#76284=CARTESIAN_POINT('Ctrl Pts',(-1.76589867700163,1.26933645129948,-5.19693713885497));
#76285=CARTESIAN_POINT('Ctrl Pts',(-1.64663270458447,5.05743447897554,-1.74405479921852));
#76286=CARTESIAN_POINT('Ctrl Pts',(-1.52736673216731,4.20289585976879,3.30983942869535));
#76287=CARTESIAN_POINT('Ctrl Pts',(-1.40810075975014,-0.509827857576372,
5.32535878673416));
#76288=CARTESIAN_POINT('Ctrl Pts',(-1.28883478733298,-4.75453849338273,
2.45229165613506));
#76289=CARTESIAN_POINT('Ctrl Pts',(-1.16956881491581,-4.63466571438527,
-2.67193644529762));
#76290=CARTESIAN_POINT('Ctrl Pts',(-1.05030284249865,-0.260250641047462,
-5.34337349018783));
#76291=CARTESIAN_POINT('Ctrl Pts',(-0.931036870081484,4.35306998183813,
-3.10968686285734));
#76292=CARTESIAN_POINT('Ctrl Pts',(-0.811770897664319,4.97034828165621,
1.97863806969469));
#76293=CARTESIAN_POINT('Ctrl Pts',(-0.692504925247154,1.02493354489289,
5.25060776295097));
#76294=CARTESIAN_POINT('Ctrl Pts',(-0.573238952829991,-3.86135231060077,
3.70261110369774));
#76295=CARTESIAN_POINT('Ctrl Pts',(-0.453972980412826,-5.20298408935945,
-1.24431797289934));
#76296=CARTESIAN_POINT('Ctrl Pts',(-0.33470700799566,-1.76836721737897,
-5.04898485205759));
#76297=CARTESIAN_POINT('Ctrl Pts',(-0.215441035578497,3.2895799187264,-4.21877169447693));
#76298=CARTESIAN_POINT('Ctrl Pts',(-0.0961750631613321,5.32775006176976,
0.484200300619735));
#76299=CARTESIAN_POINT('Ctrl Pts',(0.0230909092558323,2.4751385673978,4.74268486450319));
#76300=CARTESIAN_POINT('Ctrl Pts',(0.142356881672996,-2.64960696388247,
4.64746743815955));
#76301=CARTESIAN_POINT('Ctrl Pts',(0.261622854090164,-5.34205951311933,
0.285955958320836));
#76302=CARTESIAN_POINT('Ctrl Pts',(0.380888826507324,-3.13059459816773,
-4.33805810400583));
#76303=CARTESIAN_POINT('Ctrl Pts',(0.500154798924492,1.95470155837633,-4.9798104852985));
#76304=CARTESIAN_POINT('Ctrl Pts',(0.619420771341654,5.24561577554724,-1.05018369209291));
#76305=CARTESIAN_POINT('Ctrl Pts',(0.738686743758821,3.72114619758183,3.84349341459433));
#76306=CARTESIAN_POINT('Ctrl Pts',(0.857952716175984,-1.21927069064937,
5.20891059961017));
#76307=CARTESIAN_POINT('Ctrl Pts',(0.977218688593149,-5.040418349707,1.79263870083876));
#76308=CARTESIAN_POINT('Ctrl Pts',(1.09648466101031,-4.23454987177837,-3.26924426056382));
#76309=CARTESIAN_POINT('Ctrl Pts',(1.21575063342748,0.458561535247667,-5.33001800843103));
#76310=CARTESIAN_POINT('Ctrl Pts',(1.33501660584464,4.73072145051602,-2.49792818340231));
#76311=CARTESIAN_POINT('Ctrl Pts',(1.4542825782618,4.66016158094803,2.62721614856175));
#76312=CARTESIAN_POINT('Ctrl Pts',(1.57354855067898,0.311654656198974,5.34062187643698));
#76313=CARTESIAN_POINT('Ctrl Pts',(1.69281452309613,-4.32294580748887,3.1514298655249));
#76314=CARTESIAN_POINT('Ctrl Pts',(1.81208049551331,-4.98915741477735,-1.93071979903348));
#76315=CARTESIAN_POINT('Ctrl Pts',(1.93134646793046,-1.07540952932231,-5.24050236103854));
#76316=CARTESIAN_POINT('Ctrl Pts',(2.05061244034763,3.82554554823664,-3.73959515324518));
#76317=CARTESIAN_POINT('Ctrl Pts',(2.16987841276479,5.21471653241851,1.19419518435166));
#76318=CARTESIAN_POINT('Ctrl Pts',(2.28914438518196,1.81686868775421,5.03173517022369));
#76319=CARTESIAN_POINT('Ctrl Pts',(2.40841035759912,-3.24883292494357,4.2502300264351));
#76320=CARTESIAN_POINT('Ctrl Pts',(2.52767633001628,-5.33216257421889,-0.43291215495413));
#76321=CARTESIAN_POINT('Ctrl Pts',(2.64694230243346,-2.52065997660762,-4.71864852835388));
#76322=CARTESIAN_POINT('Ctrl Pts',(2.76620827485062,2.60476451764482,-4.67274784890289));
#76323=CARTESIAN_POINT('Ctrl Pts',(2.88547424726778,5.33906061341968,-0.337346139800582));
#76324=CARTESIAN_POINT('Ctrl Pts',(3.00474021968495,3.17219218262773,4.3077334421112));
#76325=CARTESIAN_POINT('Ctrl Pts',(3.1240061921021,-1.90669334680315,4.99838885372723));
#76326=CARTESIAN_POINT('Ctrl Pts',(3.24327216451928,-5.2352676377918,1.10061047264574));
#76327=CARTESIAN_POINT('Ctrl Pts',(3.36253813693643,-3.7579575436257,-3.8075091269903));
#76328=CARTESIAN_POINT('Ctrl Pts',(3.48180410935361,1.16909203446164,-5.22040175338702));
#76329=CARTESIAN_POINT('Ctrl Pts',(3.60107008177076,5.0229355146086,-1.84105661724222));
#76330=CARTESIAN_POINT('Ctrl Pts',(3.72033605418794,4.2658117954781,3.2283463843534));
#76331=CARTESIAN_POINT('Ctrl Pts',(3.83960202660509,-0.407252753478724,
5.33418370949033));
#76332=CARTESIAN_POINT('Ctrl Pts',(3.95886799902227,-4.7064663774845,2.54333342081128));
#76333=CARTESIAN_POINT('Ctrl Pts',(4.07813397143942,-4.68522595067329,-2.58225259084879));
#76334=CARTESIAN_POINT('Ctrl Pts',(4.1973999438566,-0.363029814411452,-5.33737576020804));
#76335=CARTESIAN_POINT('Ctrl Pts',(4.31666591627375,4.29242136001334,-3.19288106886381));
#76336=CARTESIAN_POINT('Ctrl Pts',(4.43593188869093,5.0075045884559,1.88262275785692));
#76337=CARTESIAN_POINT('Ctrl Pts',(4.55519786110808,1.12578593870418,5.22991172698201));
#76338=CARTESIAN_POINT('Ctrl Pts',(4.67446383352525,-3.78938456836793,3.77623294366524));
#76339=CARTESIAN_POINT('Ctrl Pts',(4.79372980594241,-5.22596613091239,-1.14396182207461));
#76340=CARTESIAN_POINT('Ctrl Pts',(4.91299577835959,-1.86520192939329,-5.01401958655883));
#76341=CARTESIAN_POINT('Ctrl Pts',(5.03226175077674,3.20778511302202,-4.28129481821586));
#76342=CARTESIAN_POINT('Ctrl Pts',(5.15152772319392,5.33608136745939,0.381583924793045));
#76343=CARTESIAN_POINT('Ctrl Pts',(5.27079369561107,2.56594799116161,4.69417527990397));
#76344=CARTESIAN_POINT('Ctrl Pts',(5.39005966802824,-2.5596808892866,4.69759559741243));
#76345=CARTESIAN_POINT('Ctrl Pts',(5.5093256404454,-5.33556735580349,0.388705085498125));
#76346=CARTESIAN_POINT('Ctrl Pts',(5.62859161286257,-3.21349604532058,-4.27700991564396));
#76347=CARTESIAN_POINT('Ctrl Pts',(5.74785758527973,1.85850858938807,-5.01650440794967));
#76348=CARTESIAN_POINT('Ctrl Pts',(5.86712355769689,5.22443475258933,-1.1509353447283));
#76349=CARTESIAN_POINT('Ctrl Pts',(5.98638953011406,3.79442093031935,3.77117229192225));
#76350=CARTESIAN_POINT('Ctrl Pts',(6.10565550253122,-1.11880512891234,5.2314095361888));
#76351=CARTESIAN_POINT('Ctrl Pts',(6.2249214749484,-5.00498759246291,1.88930406528444));
#76352=CARTESIAN_POINT('Ctrl Pts',(6.34418744736554,-4.29667873624274,-3.18714958690789));
#76353=CARTESIAN_POINT('Ctrl Pts',(6.46345341978273,0.355906263086912,-5.33785550419859));
#76354=CARTESIAN_POINT('Ctrl Pts',(6.58271939219988,4.68177552013038,-2.58850316416958));
#76355=CARTESIAN_POINT('Ctrl Pts',(6.70198536461705,4.70985650278392,2.5370499354549));
#76356=CARTESIAN_POINT('Ctrl Pts',(6.8212513370342,0.41437135872153,5.33363544206753));
#76357=CARTESIAN_POINT('Ctrl Pts',(6.94051730945138,-4.2614994657519,3.23403663479625));
#76358=CARTESIAN_POINT('Ctrl Pts',(7.05978328186854,-5.02538810387791,-1.83435139959879));
#76359=CARTESIAN_POINT('Ctrl Pts',(7.1790492542857,-1.17605810855195,-5.21883684139645));
#76360=CARTESIAN_POINT('Ctrl Pts',(7.29831522670288,3.75287271923664,-3.81252108256694));
#76361=CARTESIAN_POINT('Ctrl Pts',(7.41758119912002,5.23673184321061,1.09362253730968));
#76362=CARTESIAN_POINT('Ctrl Pts',(7.53684717153721,1.91336246699203,4.99583974139622));
#76363=CARTESIAN_POINT('Ctrl Pts',(7.65611314395436,-3.16644028368856,4.31196319344709));
#76364=CARTESIAN_POINT('Ctrl Pts',(7.77537911637153,-5.33950607863965,-0.330220362754721));
#76365=CARTESIAN_POINT('Ctrl Pts',(7.89464508878868,-2.6109984177212,-4.66926738519707));
#76366=CARTESIAN_POINT('Ctrl Pts',(8.01391106120587,2.51436025322183,-4.72200838296865));
#76367=CARTESIAN_POINT('Ctrl Pts',(8.13317703362301,5.33158006372075,-0.440028039951035));
#76368=CARTESIAN_POINT('Ctrl Pts',(8.25244300604019,3.25450236181101,4.2458903693777));
#76369=CARTESIAN_POINT('Ctrl Pts',(8.37170897845735,-1.81015174768696,5.0341554705982));
#76370=CARTESIAN_POINT('Ctrl Pts',(8.49097495087451,-5.21311812298558,1.20115364862579));
#76371=CARTESIAN_POINT('Ctrl Pts',(8.61024092329168,-3.83053298142016,-3.73448627391507));
#76372=CARTESIAN_POINT('Ctrl Pts',(8.72950689570885,1.06841463020081,-5.2419329287755));
#76373=CARTESIAN_POINT('Ctrl Pts',(8.848772868126,4.98657624511604,-1.93737657760491));
#76374=CARTESIAN_POINT('Ctrl Pts',(8.96803884054318,4.32714783601959,3.14565768274914));
#76375=CARTESIAN_POINT('Ctrl Pts',(9.08730481296034,-0.304526818381393,
5.34103305257461));
#76376=CARTESIAN_POINT('Ctrl Pts',(9.2065707853775,-4.65665116464621,2.63343323108956));
#76377=CARTESIAN_POINT('Ctrl Pts',(9.32583675779467,-4.73405095667114,-2.49161236781501));
#76378=CARTESIAN_POINT('Ctrl Pts',(9.44510273021184,-0.46567453527804,-5.32940126834165));
#76379=CARTESIAN_POINT('Ctrl Pts',(9.56436870262899,4.23018298784551,-3.27489275261803));
#76380=CARTESIAN_POINT('Ctrl Pts',(9.68363467504617,5.04280630516079,1.78591019383345));
#76381=CARTESIAN_POINT('Ctrl Pts',(9.80290064746333,1.2262213840307,5.20727872973531));
#76382=CARTESIAN_POINT('Ctrl Pts',(9.92216661988049,-3.71601338157262,3.84845620993417));
#76383=CARTESIAN_POINT('Ctrl Pts',(10.0414325922977,-5.24701267248705,-1.04318199110605));
#76384=CARTESIAN_POINT('Ctrl Pts',(10.1606985647148,-1.96134584123722,-4.97719731805657));
#76385=CARTESIAN_POINT('Ctrl Pts',(10.279964537132,3.12480226517166,-4.34223231246161));
#76386=CARTESIAN_POINT('Ctrl Pts',(10.3992305095491,5.34243639065652,0.278826224728918));
#76387=CARTESIAN_POINT('Ctrl Pts',(10.5184964819663,2.65580708494681,4.64392715052188));
#76388=CARTESIAN_POINT('Ctrl Pts',(10.6377624543835,-2.46880680580944,4.74598394512631));
#76389=CARTESIAN_POINT('Ctrl Pts',(10.7570284268006,-5.32709910636557,0.491310251029656));
#76390=CARTESIAN_POINT('Ctrl Pts',(10.8762943992178,-3.29520733521441,-4.21437768475455));
#76391=CARTESIAN_POINT('Ctrl Pts',(10.995560371635,1.76162729918915,-5.05134040731361));
#76392=CARTESIAN_POINT('Ctrl Pts',(11.1148263440521,5.20131879681764,-1.2512607344911));
#76393=CARTESIAN_POINT('Ctrl Pts',(11.2340923164693,3.86629035321667,3.69745446982539));
#76394=CARTESIAN_POINT('Ctrl Pts',(11.3533582888864,-1.01792520411819,5.25197095675792));
#76395=CARTESIAN_POINT('Ctrl Pts',(11.4726242613037,-4.96770317732397,1.98526970304111));
#76396=CARTESIAN_POINT('Ctrl Pts',(11.5918902337208,-4.35721627359315,-3.10387451372362));
#76397=CARTESIAN_POINT('Ctrl Pts',(11.711156206138,0.25311917672245,-5.34371606040058));
#76398=CARTESIAN_POINT('Ctrl Pts',(11.8304221785551,4.63109563736341,-2.67811946137613));
#76399=CARTESIAN_POINT('Ctrl Pts',(11.9496881509723,4.7578070721057,2.44594409511522));
#76400=CARTESIAN_POINT('Ctrl Pts',(12.0689541233894,0.51693459378251,5.32467363108372));
#76401=CARTESIAN_POINT('Ctrl Pts',(12.1882200958066,-4.19847482597077,3.31544563935193));
#76402=CARTESIAN_POINT('Ctrl Pts',(12.3074860682238,-5.05975757950666,-1.73730362586189));
#76403=CARTESIAN_POINT('Ctrl Pts',(12.4267520406409,-1.27627112038846,-5.19523846219496));
#76404=CARTESIAN_POINT('Ctrl Pts',(12.5460180130581,3.67880996828069,-3.88403499843739));
#76405=CARTESIAN_POINT('Ctrl Pts',(12.6652839854753,5.25680766681221,0.992644853889018));
#76406=CARTESIAN_POINT('Ctrl Pts',(12.7845499578925,2.00914760921968,4.95809404269169));
#76407=CARTESIAN_POINT('Ctrl Pts',(12.9038159303096,-3.08287491284709,4.37209937256074));
#76408=CARTESIAN_POINT('Ctrl Pts',(13.0230819027268,-5.34487203218452,-0.227406269436635));
#76409=CARTESIAN_POINT('Ctrl Pts',(13.1423478751439,-2.70036984388385,-4.61815692219858));
#76410=CARTESIAN_POINT('Ctrl Pts',(13.2616138475611,2.42302476496527,-4.76952006392394));
#76411=CARTESIAN_POINT('Ctrl Pts',(13.3808798199783,5.32212489864176,-0.542546970376561));
#76412=CARTESIAN_POINT('Ctrl Pts',(13.5001457923954,3.33560719654819,4.18247477961839));
#76413=CARTESIAN_POINT('Ctrl Pts',(13.6194117648126,-1.71293973690343,5.06805762689664));
#76414=CARTESIAN_POINT('Ctrl Pts',(13.7386777372298,-5.18903786661671,1.30125196277481));
#76415=CARTESIAN_POINT('Ctrl Pts',(13.8579437096469,-3.90168973483795,-3.66008030852715));
#76416=CARTESIAN_POINT('Ctrl Pts',(13.9772096820641,0.96734152561576,-5.26152269068825));
#76417=CARTESIAN_POINT('Ctrl Pts',(14.0964756544813,4.94837013659463,-2.03297900704013));
#76418=CARTESIAN_POINT('Ctrl Pts',(14.2157416268984,4.38688126484615,3.06180394864691));
#76419=CARTESIAN_POINT('Ctrl Pts',(14.3350075993156,-0.201688098081399,
5.3459042792497));
#76420=CARTESIAN_POINT('Ctrl Pts',(14.4542735717327,-4.60511130453659,2.72255771741147));
#76421=CARTESIAN_POINT('Ctrl Pts',(14.5735395441499,-4.78112264944524,-2.40004934590306));
#76422=CARTESIAN_POINT('Ctrl Pts',(14.6928055165671,-0.568146787928893,
-5.31945296803855));
#76423=CARTESIAN_POINT('Ctrl Pts',(14.8120714889842,4.16637791607122,-3.35569154009744));
#76424=CARTESIAN_POINT('Ctrl Pts',(14.9313374614014,5.07624035735161,1.68853619629629));
#76425=CARTESIAN_POINT('Ctrl Pts',(15.0506034338186,1.32620268338616,5.18271715361618));
#76426=CARTESIAN_POINT('Ctrl Pts',(15.1698694062357,-3.64126592412445,3.91925415374118));
#76427=CARTESIAN_POINT('Ctrl Pts',(15.2891353786529,-5.26611591924131,-0.942015805027344));
#76428=CARTESIAN_POINT('Ctrl Pts',(15.4084013510701,-2.05676334484598,-4.93853168412494));
#76429=CARTESIAN_POINT('Ctrl Pts',(15.5276673234872,3.0406621088803,-4.40156160827348));
#76430=CARTESIAN_POINT('Ctrl Pts',(15.6469332959044,5.34681277770121,0.175965257988861));
#76431=CARTESIAN_POINT('Ctrl Pts',(15.7661992683216,2.74468256834738,4.5919590863615));
#76432=CARTESIAN_POINT('Ctrl Pts',(15.8854652407387,-2.3770183697707,4.79261456008932));
#76433=CARTESIAN_POINT('Ctrl Pts',(16.0047312131559,-5.31665790112462,0.593733453847086));
#76434=CARTESIAN_POINT('Ctrl Pts',(16.123997185573,-3.37569820508123,-4.15018460794448));
#76435=CARTESIAN_POINT('Ctrl Pts',(16.2432631579902,1.66409356894118,-5.08430558145515));
#76436=CARTESIAN_POINT('Ctrl Pts',(16.3625291304074,5.17627646950703,-1.35112270465559));
#76437=CARTESIAN_POINT('Ctrl Pts',(16.4817951028246,3.93672784856066,3.62236725059386));
#76438=CARTESIAN_POINT('Ctrl Pts',(16.6010610752417,-0.916668278371397,
5.27058724614582));
#76439=CARTESIAN_POINT('Ctrl Pts',(16.7203270476589,-4.92857891302596,2.08050007207014));
#76440=CARTESIAN_POINT('Ctrl Pts',(16.839593020076,-4.41614006301782,-3.01944988294506));
#76441=CARTESIAN_POINT('Ctrl Pts',(16.9588589924932,0.150238344599186,-5.34759750650883));
#76442=CARTESIAN_POINT('Ctrl Pts',(17.0781249649104,4.57870057212474,-2.76674388453876));
#76443=CARTESIAN_POINT('Ctrl Pts',(17.1973909373275,4.80399552983808,2.35393236969624));
#76444=CARTESIAN_POINT('Ctrl Pts',(17.3166569097447,0.619306375843183,5.31373976260104));
#76445=CARTESIAN_POINT('Ctrl Pts',(17.4359228821619,-4.13389523008567,3.39562672837916));
#76446=CARTESIAN_POINT('Ctrl Pts',(17.555188854579,-5.09225311251117,-1.63961242064348));
#76447=CARTESIAN_POINT('Ctrl Pts',(17.6744548269962,-1.37601144972682,-5.1697159633802));
#76448=CARTESIAN_POINT('Ctrl Pts',(17.7937207994134,3.60338472540743,-3.95411041480993));
#76449=CARTESIAN_POINT('Ctrl Pts',(17.9129867718305,5.27493656789836,0.891299532400152));
#76450=CARTESIAN_POINT('Ctrl Pts',(18.0322527442477,2.10418863924757,4.91851205368746));
#76451=CARTESIAN_POINT('Ctrl Pts',(18.1515187166648,-2.99816776186809,4.43061629161259));
#76452=CARTESIAN_POINT('Ctrl Pts',(18.270784689082,-5.34825844750761,-0.124507953446764));
#76453=CARTESIAN_POINT('Ctrl Pts',(18.3900506614992,-2.78874115530351,-4.5653360687384));
#76454=CARTESIAN_POINT('Ctrl Pts',(18.5093166339163,2.33079188008128,-4.81526529524129));
#76455=CARTESIAN_POINT('Ctrl Pts',(18.6285826063335,5.31069862001794,-0.644864961947463));
#76456=CARTESIAN_POINT('Ctrl Pts',(18.7478485787507,3.41547664867964,4.11751015956628));
#76457=CARTESIAN_POINT('Ctrl Pts',(18.8671145511678,-1.61509331810011,5.10008276654765));
#76458=CARTESIAN_POINT('Ctrl Pts',(18.986380523585,-5.16303578710043,1.40086834246771));
#76459=CARTESIAN_POINT('Ctrl Pts',(19.1056464960022,-3.971401450112,-3.58431878797852));
#76460=CARTESIAN_POINT('Ctrl Pts',(19.2249124684193,0.865910154356953,-5.27916378381931));
#76461=CARTESIAN_POINT('Ctrl Pts',(19.3441784408365,4.9083313391403,-2.12782849802824));
#76462=CARTESIAN_POINT('Ctrl Pts',(19.4634444132536,4.4449899589576,2.97681623829445));
#76463=CARTESIAN_POINT('Ctrl Pts',(19.5827103856708,-0.0987746801464204,
5.3487955853977));
#76464=CARTESIAN_POINT('Ctrl Pts',(19.701976358088,-4.55186588556823,2.81067387144225));
#76465=CARTESIAN_POINT('Ctrl Pts',(19.8212423305052,-4.82642359542294,-2.30759743658899));
#76466=CARTESIAN_POINT('Ctrl Pts',(19.9405083029223,-0.670408620522066,
-5.30753454377244));
#76467=CARTESIAN_POINT('Ctrl Pts',(20.0597742753395,4.10102977567299,-3.43524750649084));
#76468=CARTESIAN_POINT('Ctrl Pts',(20.1790402477567,5.10779436232139,1.59053682888681));
#76469=CARTESIAN_POINT('Ctrl Pts',(20.2983062201738,1.42569280748336,5.15623609530228));
#76470=CARTESIAN_POINT('Ctrl Pts',(20.417572192591,-3.56516987965126,3.98860055420888));
#76471=CARTESIAN_POINT('Ctrl Pts',(20.5368381650081,-5.28326879605584,-0.840500731962909));
#76472=CARTESIAN_POINT('Ctrl Pts',(20.6561041374253,-2.1514191011895,-4.89803700505059));
#76473=CARTESIAN_POINT('Ctrl Pts',(20.7753701098425,2.95539580647574,-4.45926073232701));
#76474=CARTESIAN_POINT('Ctrl Pts',(20.8946360822597,5.34920890774529,0.0730391203798664));
#76475=CARTESIAN_POINT('Ctrl Pts',(21.0139020546768,2.83254152524977,4.53829033442592));
#76476=CARTESIAN_POINT('Ctrl Pts',(21.133168027094,-2.28434957613141,4.83747017208749));
#76477=CARTESIAN_POINT('Ctrl Pts',(21.2524339995111,-5.30424760710754,0.69593676027454));
#76478=CARTESIAN_POINT('Ctrl Pts',(21.3716999719283,-3.45493884415087,-4.08445445989859));
#76479=CARTESIAN_POINT('Ctrl Pts',(21.4909659443455,1.56594352144461,-5.11538772132217));
#76480=CARTESIAN_POINT('Ctrl Pts',(21.6102319167626,5.14931704538713,-1.45048427012945));
#76481=CARTESIAN_POINT('Ctrl Pts',(21.7294978891798,4.00570732897041,3.54593844369029));
#76482=CARTESIAN_POINT('Ctrl Pts',(21.848763861597,-0.81507185340302,5.28725150958398));
#76483=CARTESIAN_POINT('Ctrl Pts',(21.9680298340141,-4.88762928971471,2.17495990264885));
#76484=CARTESIAN_POINT('Ctrl Pts',(22.0872958064313,-4.4734282813765,-2.93390696225849));
#76485=CARTESIAN_POINT('Ctrl Pts',(22.2065617788485,0.0473018698816033,
-5.34949840498282));
#76486=CARTESIAN_POINT('Ctrl Pts',(22.3258277512656,4.5246097295625,-2.85434361052691));
#76487=CARTESIAN_POINT('Ctrl Pts',(22.4450937236827,4.84840476952531,2.26104883685696));
#76488=CARTESIAN_POINT('Ctrl Pts',(22.5643596961,0.72144879027182,5.30083788611039));
#76489=CARTESIAN_POINT('Ctrl Pts',(22.6836256685171,-4.06778459593354,3.47455020583862));
#76490=CARTESIAN_POINT('Ctrl Pts',(22.8028916409343,-5.12286266777649,-1.54131396506679));
#76491=CARTESIAN_POINT('Ctrl Pts',(22.9221576133515,-1.47524215652576,-5.14227879751937));
#76492=CARTESIAN_POINT('Ctrl Pts',(23.0414235857686,3.52662492527076,-4.02272137840373));
#76493=CARTESIAN_POINT('Ctrl Pts',(23.1606895581858,5.29111183221057,0.789624107312617));
#76494=CARTESIAN_POINT('Ctrl Pts',(23.2799555306029,2.19845035747676,4.87710843405375));
#76495=CARTESIAN_POINT('Ctrl Pts',(23.3992215030201,-2.91235020307306,4.48749227815132));
#76496=CARTESIAN_POINT('Ctrl Pts',(23.5184874754372,-5.34966407040875,-0.0215635244252718));
#76497=CARTESIAN_POINT('Ctrl Pts',(23.6377534478544,-2.87607962259252,-4.51082438766087));
#76498=CARTESIAN_POINT('Ctrl Pts',(23.7570194202716,2.2376957581383,-4.85922713461897));
#76499=CARTESIAN_POINT('Ctrl Pts',(23.8762853926887,5.2973054597101,-0.746944119953741));
#76500=CARTESIAN_POINT('Ctrl Pts',(23.9955513651059,3.49408113758448,4.05102056965703));
#76501=CARTESIAN_POINT('Ctrl Pts',(24.1148173375231,-1.51664872988588,5.13021902865199));
#76502=CARTESIAN_POINT('Ctrl Pts',(24.2340833099402,-5.13512151462232,1.49996589356924));
#76503=CARTESIAN_POINT('Ctrl Pts',(24.3533492823574,-4.03964230866261,-3.50722977146794));
#76504=CARTESIAN_POINT('Ctrl Pts',(24.4726152547746,0.764158082763927,-5.29484967457566));
#76505=CARTESIAN_POINT('Ctrl Pts',(24.5918812271917,4.86647468160752,-2.22188992190905));
#76506=CARTESIAN_POINT('Ctrl Pts',(24.7111471996089,4.50145239709396,2.89072602792189));
#76507=CARTESIAN_POINT('Ctrl Pts',(24.8304131720261,0.00417532019002488,
5.34970590018823));
#76508=CARTESIAN_POINT('Ctrl Pts',(24.9496791444432,-4.49693462782816,2.89774905829474));
#76509=CARTESIAN_POINT('Ctrl Pts',(25.0689451168604,-4.86993701684925,-2.21429088055959));
#76510=CARTESIAN_POINT('Ctrl Pts',(25.1882110892776,-0.772422159146575,
-5.29365040967637));
#76511=CARTESIAN_POINT('Ctrl Pts',(25.3074770616947,4.03416276912766,-3.51353118728043));
#76512=CARTESIAN_POINT('Ctrl Pts',(25.4267430341119,5.13745663366157,1.49194838686019));
#76513=CARTESIAN_POINT('Ctrl Pts',(25.546009006529,1.52465490894722,5.12784536237498));
#76514=CARTESIAN_POINT('Ctrl Pts',(25.6652749789462,-3.48775343124658,4.05646972805612));
#76515=CARTESIAN_POINT('Ctrl Pts',(25.7845409513634,-5.2984649501547,-0.738674369252185));
#76516=CARTESIAN_POINT('Ctrl Pts',(25.9038069237805,-2.24527805335948,-4.85572827852936));
#76517=CARTESIAN_POINT('Ctrl Pts',(26.0230728961977,2.86903493736783,-4.51530831505123));
#76518=CARTESIAN_POINT('Ctrl Pts',(26.1423388686148,5.34962389335311,-0.0299140681537413));
#76519=CARTESIAN_POINT('Ctrl Pts',(26.2616048410321,2.91935141602282,4.48294077158877));
#76520=CARTESIAN_POINT('Ctrl Pts',(26.3808708134492,-2.19083474590394,4.88053416830044));
#76521=CARTESIAN_POINT('Ctrl Pts',(26.5001367858664,-5.28987282061753,0.797882318077011));
#76522=CARTESIAN_POINT('Ctrl Pts',(26.6194027582835,-3.53289990469077,-4.01721158457497));
#76523=CARTESIAN_POINT('Ctrl Pts',(26.7386687307007,1.4672135077607,-5.14457531526681));
#76524=CARTESIAN_POINT('Ctrl Pts',(26.8579347031179,5.12045050920806,-1.54930863115098));
#76525=CARTESIAN_POINT('Ctrl Pts',(26.977200675535,4.073203247058,3.46819635545099));
#76526=CARTESIAN_POINT('Ctrl Pts',(27.0964666479522,-0.713173556682066,
5.30195757526005));
#76527=CARTESIAN_POINT('Ctrl Pts',(27.2157326203693,-4.8448694735804,2.2686142104326));
#76528=CARTESIAN_POINT('Ctrl Pts',(27.3349985927865,-4.5290597112821,-2.8472774335229));
#76529=CARTESIAN_POINT('Ctrl Pts',(27.4542645652037,-0.0556521236575815,
-5.34941805180156));
#76530=CARTESIAN_POINT('Ctrl Pts',(27.5735305376208,4.46884314287686,-2.94088619571898));
#76531=CARTESIAN_POINT('Ctrl Pts',(27.692796510038,4.89101834366639,2.16732789714115));
#76532=CARTESIAN_POINT('Ctrl Pts',(27.8120624824552,0.823324007385604,5.2859727799782));
#76533=CARTESIAN_POINT('Ctrl Pts',(27.9313284548724,-4.00016740839022,3.55218684146269));
#76534=CARTESIAN_POINT('Ctrl Pts',(28.0505944272895,-5.15157490868226,-1.44244466515798));
#76535=CARTESIAN_POINT('Ctrl Pts',(28.1698603997067,-1.57392648948877,-5.11293712629961));
#76536=CARTESIAN_POINT('Ctrl Pts',(28.2891263721238,3.44855899679427,-4.08984247831593));
#76537=CARTESIAN_POINT('Ctrl Pts',(28.408392344541,5.30532746904341,0.687656235354114));
#76538=CARTESIAN_POINT('Ctrl Pts',(28.5276583169582,2.291897852936,4.83389851812331));
#76539=CARTESIAN_POINT('Ctrl Pts',(28.6469242893753,-2.82545402003632,4.54270626746531));
#76540=CARTESIAN_POINT('Ctrl Pts',(28.7661902617925,-5.34908838029851,0.0813888909092254));
#76541=CARTESIAN_POINT('Ctrl Pts',(28.8854562342096,-2.96235289888958,-4.45464206802835));
#76542=CARTESIAN_POINT('Ctrl Pts',(29.0047222066268,2.14377087841479,-4.90138930025648));
#76543=CARTESIAN_POINT('Ctrl Pts',(29.123988179044,5.28195037803777,-0.848746638140402));
#76544=CARTESIAN_POINT('Ctrl Pts',(29.2432541514612,3.57139155113628,3.98303063511691));
#76545=CARTESIAN_POINT('Ctrl Pts',(29.3625201238783,-1.41764243240855,5.15845525187946));
#76546=CARTESIAN_POINT('Ctrl Pts',(29.4817860962955,-5.10530538757201,1.5985079140987));
#76547=CARTESIAN_POINT('Ctrl Pts',(29.6010520687126,-4.10638703665957,-3.42884180984799));
#76548=CARTESIAN_POINT('Ctrl Pts',(29.7203180411298,0.662122995951101,-5.30857455349746));
#76549=CARTESIAN_POINT('Ctrl Pts',(29.839584013547,4.8228156661174,-2.31512844189271));
#76550=CARTESIAN_POINT('Ctrl Pts',(29.9588499859641,4.55624766770592,2.8035652020832));
#76551=CARTESIAN_POINT('Ctrl Pts',(30.0781159583813,0.107123774146093,5.34863488647531));
#76552=CARTESIAN_POINT('Ctrl Pts',(30.1973819307985,-4.44033787577436,2.98375102861677));
#76553=CARTESIAN_POINT('Ctrl Pts',(30.3166479032156,-4.91164679800034,-2.12016423503002));
#76554=CARTESIAN_POINT('Ctrl Pts',(30.4359138756328,-0.874149621850558,
-5.27780570790802));
#76555=CARTESIAN_POINT('Ctrl Pts',(30.55517984805,3.96580166144261,-3.59051358915504));
#76556=CARTESIAN_POINT('Ctrl Pts',(30.6744458204671,5.16521618558982,1.39280738364225));
#76557=CARTESIAN_POINT('Ctrl Pts',(30.7937117928843,1.62305233596266,5.09755546968683));
#76558=CARTESIAN_POINT('Ctrl Pts',(30.9129777653015,-3.40904525103163,4.12283653911075));
#76559=CARTESIAN_POINT('Ctrl Pts',(31.0322437377186,-5.31169875345763,-0.636574429524205));
#76560=CARTESIAN_POINT('Ctrl Pts',(31.1515097101358,-2.33830543955411,-4.81162117411165));
#76561=CARTESIAN_POINT('Ctrl Pts',(31.270775682553,2.78161148635255,-4.56968359854373));
#76562=CARTESIAN_POINT('Ctrl Pts',(31.3900416549701,5.34805758082949,-0.132856177649306));
#76563=CARTESIAN_POINT('Ctrl Pts',(31.5093076273873,3.00508008957021,4.42593089723243));
#76564=CARTESIAN_POINT('Ctrl Pts',(31.6285735998045,-2.09650851344057,4.92179059945456));
#76565=CARTESIAN_POINT('Ctrl Pts',(31.7478395722216,-5.27353886553098,0.8995323704801));
#76566=CARTESIAN_POINT('Ctrl Pts',(31.8671055446388,-3.60955251287627,-3.94848088618859));
#76567=CARTESIAN_POINT('Ctrl Pts',(31.986371517056,1.36794009374822,-5.17185755330946));
#76568=CARTESIAN_POINT('Ctrl Pts',(32.1056374894731,5.08968755204155,-1.64755918691883));
#76569=CARTESIAN_POINT('Ctrl Pts',(32.2249034618903,4.13919060489128,3.3891697786018));
#76570=CARTESIAN_POINT('Ctrl Pts',(32.3441694343074,-0.611011127479355,
5.31469999660417));
#76571=CARTESIAN_POINT('Ctrl Pts',(32.4634354067246,-4.80031530123962,2.36142830941194));
#76572=CARTESIAN_POINT('Ctrl Pts',(32.5827013791417,-4.58301374895963,-2.75959338103551));
#76573=CARTESIAN_POINT('Ctrl Pts',(32.701967351559,-0.15858550575743,-5.34735647672489));
#76574=CARTESIAN_POINT('Ctrl Pts',(32.821233323976,4.41142146589973,-3.02633958801825));
#76575=CARTESIAN_POINT('Ctrl Pts',(32.9404992963933,4.93182046980722,2.07280426123612));
#76576=CARTESIAN_POINT('Ctrl Pts',(33.0597652688104,0.924894296461516,5.26914994967698));
#76577=CARTESIAN_POINT('Ctrl Pts',(33.1790312412276,-3.93106871030145,3.6285078815811));
#76578=CARTESIAN_POINT('Ctrl Pts',(33.2982972136447,-5.17837920130185,-1.34304113836196));
#76579=CARTESIAN_POINT('Ctrl Pts',(33.417563186062,-1.67202789967526,-5.08170181676528));
#76580=CARTESIAN_POINT('Ctrl Pts',(33.536829158479,3.36921585264198,-4.15544885543223));
#76581=CARTESIAN_POINT('Ctrl Pts',(33.6560951308963,5.31757821346333,0.585433681563546));
#76582=CARTESIAN_POINT('Ctrl Pts',(33.7753611033134,2.38449651621095,4.78889830921323));
#76583=CARTESIAN_POINT('Ctrl Pts',(33.8946270757306,-2.73751139581363,4.59623781038317));
#76584=CARTESIAN_POINT('Ctrl Pts',(34.0138930481477,-5.34653159039126,0.184311162880282));
#76585=CARTESIAN_POINT('Ctrl Pts',(34.1331590205649,-3.04752903183865,-4.39680991764522));
#76586=CARTESIAN_POINT('Ctrl Pts',(34.252424992982,2.04905202712797,-4.94173617688352));
#76587=CARTESIAN_POINT('Ctrl Pts',(34.3716909653993,5.26463906194561,-0.95023481270979));
#76588=CARTESIAN_POINT('Ctrl Pts',(34.4909569378164,3.64737925647783,3.91356553684459));
#76589=CARTESIAN_POINT('Ctrl Pts',(34.6102229102336,-1.31811109383836,5.18478097860004));
#76590=CARTESIAN_POINT('Ctrl Pts',(34.7294888826507,-5.0735984487402,1.69645790782622));
#76591=CARTESIAN_POINT('Ctrl Pts',(34.8487548550679,-4.17161091433314,-3.34918393505835));
#76592=CARTESIAN_POINT('Ctrl Pts',(34.968020827485,0.559842683756944,-5.32033333739675));
#76593=CARTESIAN_POINT('Ctrl Pts',(35.0872867999022,4.7773704624956,-2.40750952598498));
#76594=CARTESIAN_POINT('Ctrl Pts',(35.2065527723194,4.60935547635934,2.71536604189249));
#76595=CARTESIAN_POINT('Ctrl Pts',(35.3258187447365,0.210032554159402,5.34558294083782));
#76596=CARTESIAN_POINT('Ctrl Pts',(35.4450847171537,-4.38209659193005,3.06864793069408));
#76597=CARTESIAN_POINT('Ctrl Pts',(35.5643506895709,-4.951537488818,-2.02525236124853));
#76598=CARTESIAN_POINT('Ctrl Pts',(35.6836166619881,-0.975553337067666,
-5.26000630617043));
#76599=CARTESIAN_POINT('Ctrl Pts',(35.8028826344052,3.89597177940602,-3.66616620183877));
#76600=CARTESIAN_POINT('Ctrl Pts',(35.9221486068224,5.19106272102259,1.29315053937908));
#76601=CARTESIAN_POINT('Ctrl Pts',(36.0414145792395,1.72084867623149,5.06537763153141));
#76602=CARTESIAN_POINT('Ctrl Pts',(36.1606805516567,-3.32907454724463,4.18767641509399));
#76603=CARTESIAN_POINT('Ctrl Pts',(36.2799465240739,-5.322965195057,-0.53423874092893));
#76604=CARTESIAN_POINT('Ctrl Pts',(36.399212496491,-2.4304670141352,-4.76573200043202));
#76605=CARTESIAN_POINT('Ctrl Pts',(36.5184784689082,2.69315822717824,-4.62236649547752));
#76606=CARTESIAN_POINT('Ctrl Pts',(36.6377444413254,5.34450979925368,-0.235748984964162));
#76607=CARTESIAN_POINT('Ctrl Pts',(36.7570104137425,3.08969722168957,4.36728164088206));
#76608=CARTESIAN_POINT('Ctrl Pts',(36.8762763861597,-2.00140852293053,4.96122453667856));
#76609=CARTESIAN_POINT('Ctrl Pts',(36.9955423585768,-5.25524664538787,1.00084860358074));
#76610=CARTESIAN_POINT('Ctrl Pts',(37.114808330994,-3.68487805339145,-3.87828655393761));
#76611=CARTESIAN_POINT('Ctrl Pts',(37.2340743034112,1.26817861053563,-5.1972267358067));
#76612=CARTESIAN_POINT('Ctrl Pts',(37.3533402758283,5.05700430786462,-1.745194981863));
#76613=CARTESIAN_POINT('Ctrl Pts',(37.4726062482455,4.20371193315622,3.30887930675979));
#76614=CARTESIAN_POINT('Ctrl Pts',(37.5918722206627,-0.508749602332581,
5.32549053072501));
#76615=CARTESIAN_POINT('Ctrl Pts',(37.7111381930799,-4.75374167366011,2.45333653102065));
#76616=CARTESIAN_POINT('Ctrl Pts',(37.830404165497,-4.63572933387,-2.67082784760058));
#76617=CARTESIAN_POINT('Ctrl Pts',(37.9496701379142,-0.260588162173769,
-5.34342727819689));
#76618=CARTESIAN_POINT('Ctrl Pts',(38.0689361103313,4.35070685430609,-3.11045822607375));
#76619=CARTESIAN_POINT('Ctrl Pts',(38.1882020827485,4.97397191480465,1.9771100447851));
#76620=CARTESIAN_POINT('Ctrl Pts',(38.3074680551657,1.01988032406546,5.25111166397229));
#76621=CARTESIAN_POINT('Ctrl Pts',(38.4068563655133,-3.03575591970712,3.96049046164289));
#76622=CARTESIAN_POINT('Ctrl Pts',(38.4863670137914,-4.54515679744195,1.22768957972598));
#76623=CARTESIAN_POINT('Ctrl Pts',(38.5261223379305,-4.57497191465336,-0.318504194825992));
#76624=CARTESIAN_POINT('Ctrl Pts',(38.546,-4.39991769847472,-1.05120802372743));
#76625=CARTESIAN_POINT('Ctrl Pts',(-17.7840033022126,-1.9938567537982,4.21983174306485));
#76626=CARTESIAN_POINT('Ctrl Pts',(-17.764125640143,-2.69657146060628,3.88780133297438));
#76627=CARTESIAN_POINT('Ctrl Pts',(-17.724370316004,-3.92180026446256,2.86581084683925));
#76628=CARTESIAN_POINT('Ctrl Pts',(-17.6448596677259,-5.14708318505065,
-0.112939977084765));
#76629=CARTESIAN_POINT('Ctrl Pts',(-17.5454713573783,-3.56813811963232,
-4.21020221567445));
#76630=CARTESIAN_POINT('Ctrl Pts',(-17.426205384961,1.6191574350232,-5.27949136677745));
#76631=CARTESIAN_POINT('Ctrl Pts',(-17.3069394125439,5.3116616510009,-1.49406917373198));
#76632=CARTESIAN_POINT('Ctrl Pts',(-17.1876734401267,4.13252590194496,3.65866187852482));
#76633=CARTESIAN_POINT('Ctrl Pts',(-17.0684074677096,-0.842490899558503,
5.45501402271219));
#76634=CARTESIAN_POINT('Ctrl Pts',(-16.9491414952924,-5.04290871094292,
2.24259701600285));
#76635=CARTESIAN_POINT('Ctrl Pts',(-16.8298755228753,-4.61465967021616,
-3.02787363897754));
#76636=CARTESIAN_POINT('Ctrl Pts',(-16.7106095504581,0.0501009852498292,
-5.5191309278913));
#76637=CARTESIAN_POINT('Ctrl Pts',(-16.5913435780409,4.66869368758116,-2.94375284374969));
#76638=CARTESIAN_POINT('Ctrl Pts',(-16.4720776056238,5.00159973752036,2.33384980148805));
#76639=CARTESIAN_POINT('Ctrl Pts',(-16.3528116332066,0.743075638461223,
5.46906600082232));
#76640=CARTESIAN_POINT('Ctrl Pts',(-16.2335456607894,-4.19755323287798,
3.58375026676195));
#76641=CARTESIAN_POINT('Ctrl Pts',(-16.1142796883723,-5.28491497754428,
-1.59137268981239));
#76642=CARTESIAN_POINT('Ctrl Pts',(-15.9950137159551,-1.52080981986866,
-5.30565012642365));
#76643=CARTESIAN_POINT('Ctrl Pts',(-15.8757477435379,3.63936847718576,-4.14942967182103));
#76644=CARTESIAN_POINT('Ctrl Pts',(-15.7564817711208,5.45867196013972,0.815892952732853));
#76645=CARTESIAN_POINT('Ctrl Pts',(-15.6372157987036,2.26700874645107,5.03224107677712));
#76646=CARTESIAN_POINT('Ctrl Pts',(-15.5179498262864,-3.00572841093485,
4.62907913105125));
#76647=CARTESIAN_POINT('Ctrl Pts',(-15.3986838538693,-5.5192595971191,-0.0234964456327061));
#76648=CARTESIAN_POINT('Ctrl Pts',(-15.2794178814521,-2.96620658071756,
-4.65450284102427));
#76649=CARTESIAN_POINT('Ctrl Pts',(-15.160151909035,2.30977226438264,-5.01275672892111));
#76650=CARTESIAN_POINT('Ctrl Pts',(-15.0408859366178,5.46542049672021,-0.769387405749975));
#76651=CARTESIAN_POINT('Ctrl Pts',(-14.9216199642006,3.60390801126691,4.18026615861146));
#76652=CARTESIAN_POINT('Ctrl Pts',(-14.8023539917834,-1.56592916246069,
5.29250828460176));
#76653=CARTESIAN_POINT('Ctrl Pts',(-14.6830880193663,-5.29827068197203,
1.54632011588519));
#76654=CARTESIAN_POINT('Ctrl Pts',(-14.5638220469491,-4.16689211735099,
-3.61936295353509));
#76655=CARTESIAN_POINT('Ctrl Pts',(-14.444556074532,0.789620736094701,-5.46253395392374));
#76656=CARTESIAN_POINT('Ctrl Pts',(-14.3252901021148,5.02127552618045,-2.29119405547708));
#76657=CARTESIAN_POINT('Ctrl Pts',(-14.2060241296976,4.64348695694276,2.98342202649576));
#76658=CARTESIAN_POINT('Ctrl Pts',(-14.0867581572805,0.00305834679333195,
5.51930872065043));
#76659=CARTESIAN_POINT('Ctrl Pts',(-13.9674921848633,-4.64017777250366,
2.98856626956584));
#76660=CARTESIAN_POINT('Ctrl Pts',(-13.8482262124461,-5.02381162417254,
-2.28562789458371));
#76661=CARTESIAN_POINT('Ctrl Pts',(-13.728960240029,-0.795674023300409,
-5.46165551424887));
#76662=CARTESIAN_POINT('Ctrl Pts',(-13.6096942676118,4.16287845392856,-3.62397862653602));
#76663=CARTESIAN_POINT('Ctrl Pts',(-13.4904282951946,5.29998111364186,1.54044743589541));
#76664=CARTESIAN_POINT('Ctrl Pts',(-13.3711623227775,1.57179354601877,5.29076961853536));
#76665=CARTESIAN_POINT('Ctrl Pts',(-13.2518963503603,-3.59927308379099,
4.18425756568985));
#76666=CARTESIAN_POINT('Ctrl Pts',(-13.1326303779432,-5.46626979625021,
-0.763329956394489));
#76667=CARTESIAN_POINT('Ctrl Pts',(-13.013364405526,-2.31532617091257,-5.01019389145924));
#76668=CARTESIAN_POINT('Ctrl Pts',(-12.8940984331088,2.96104649858842,-4.65778721507616));
#76669=CARTESIAN_POINT('Ctrl Pts',(-12.7748324606917,5.51923012488573,-0.0296131099717272));
#76670=CARTESIAN_POINT('Ctrl Pts',(-12.6555664882745,3.01085675535932,4.6257453136155));
#76671=CARTESIAN_POINT('Ctrl Pts',(-12.5363005158573,-2.26143060436429,
5.03475021519175));
#76672=CARTESIAN_POINT('Ctrl Pts',(-12.4170345434402,-5.45776411004393,
0.821942228410921));
#76673=CARTESIAN_POINT('Ctrl Pts',(-12.297768571023,-3.64396534951881,-4.14539438886518));
#76674=CARTESIAN_POINT('Ctrl Pts',(-12.1785025986058,1.51493004883248,-5.30733125543085));
#76675=CARTESIAN_POINT('Ctrl Pts',(-12.0592366261887,5.28314608368199,-1.59723059268359));
#76676=CARTESIAN_POINT('Ctrl Pts',(-11.9399706537715,4.20152615507953,3.57909989744786));
#76677=CARTESIAN_POINT('Ctrl Pts',(-11.8207046813543,-0.737021506645064,
5.46987910346027));
#76678=CARTESIAN_POINT('Ctrl Pts',(-11.7014387089372,-4.99899627938499,
2.33940469060478));
#76679=CARTESIAN_POINT('Ctrl Pts',(-11.58217273652,-4.67197965326751,-2.93860242754666));
#76680=CARTESIAN_POINT('Ctrl Pts',(-11.4629067641029,-0.056167187694204,
-5.51902376827236));
#76681=CARTESIAN_POINT('Ctrl Pts',(-11.3436407916857,4.61120577659153,-3.03307754494631));
#76682=CARTESIAN_POINT('Ctrl Pts',(-11.2243748192685,5.04557226027564,2.23718096587329));
#76683=CARTESIAN_POINT('Ctrl Pts',(-11.1051088468514,0.848191406958907,
5.45374636785483));
#76684=CARTESIAN_POINT('Ctrl Pts',(-10.9858428744342,-4.1278143649581,3.66386772088927));
#76685=CARTESIAN_POINT('Ctrl Pts',(-10.866576902017,-5.31455854150475,-1.48937759371077));
#76686=CARTESIAN_POINT('Ctrl Pts',(-10.7473109295999,-1.62263066617103,
-5.27540025295996));
#76687=CARTESIAN_POINT('Ctrl Pts',(-10.6280449571827,3.55884386101522,-4.2186974862679));
#76688=CARTESIAN_POINT('Ctrl Pts',(-10.5087789847655,5.47336179224965,0.71069599609851));
#76689=CARTESIAN_POINT('Ctrl Pts',(-10.3895130123484,2.36342905704779,4.98768294902862));
#76690=CARTESIAN_POINT('Ctrl Pts',(-10.2702470399312,-2.91609033284473,
4.68606394305692));
#76691=CARTESIAN_POINT('Ctrl Pts',(-10.150981067514,-5.5186896556229,0.0827199652415343));
#76692=CARTESIAN_POINT('Ctrl Pts',(-10.0317150950969,-3.05522812393436,
-4.59655949797773));
#76693=CARTESIAN_POINT('Ctrl Pts',(-9.91244912267972,2.21287954043883,-5.05627750892255));
#76694=CARTESIAN_POINT('Ctrl Pts',(-9.79318315026254,5.44960238069073,-0.874420951314895));
#76695=CARTESIAN_POINT('Ctrl Pts',(-9.67391717784538,3.68368527993848,4.11013878915217));
#76696=CARTESIAN_POINT('Ctrl Pts',(-9.55465120542822,-1.46379066202483,
5.32166280456567));
#76697=CARTESIAN_POINT('Ctrl Pts',(-9.43538523301106,-5.26753230567291,
1.64799317851164));
#76698=CARTESIAN_POINT('Ctrl Pts',(-9.31611926059388,-4.23577116176733,
-3.53850544338552));
#76699=CARTESIAN_POINT('Ctrl Pts',(-9.19685328817674,0.684354034145503,
-5.47671778200023));
#76700=CARTESIAN_POINT('Ctrl Pts',(-9.07758731575955,4.97625416227462,-2.38739871411816));
#76701=CARTESIAN_POINT('Ctrl Pts',(-8.95832134334239,4.70003975841694,2.89351073559937));
#76702=CARTESIAN_POINT('Ctrl Pts',(-8.83905537092524,0.109270827962002,
5.51822779467152));
#76703=CARTESIAN_POINT('Ctrl Pts',(-8.71978939850806,-4.58180681681053,
3.07730797957519));
#76704=CARTESIAN_POINT('Ctrl Pts',(-8.60052342609089,-5.06686571332418,
-2.18852689059757));
#76705=CARTESIAN_POINT('Ctrl Pts',(-8.48125745367375,-0.900630254309538,
-5.44533224447794));
#76706=CARTESIAN_POINT('Ctrl Pts',(-8.36199148125656,4.09236807060697,-3.7034175679236));
#76707=CARTESIAN_POINT('Ctrl Pts',(-8.24272550883941,5.32864388016197,1.43816984606865));
#76708=CARTESIAN_POINT('Ctrl Pts',(-8.12345953642224,1.67331754260636,5.25954242395045));
#76709=CARTESIAN_POINT('Ctrl Pts',(-8.00419356400508,-3.5180851153586,4.25274678635124));
#76710=CARTESIAN_POINT('Ctrl Pts',(-7.88492759158791,-5.47994699502656,
-0.657996230557716));
#76711=CARTESIAN_POINT('Ctrl Pts',(-7.76566161917075,-2.41131310695906,
-4.96471018368004));
#76712=CARTESIAN_POINT('Ctrl Pts',(-7.64639564675358,2.8708641584899,-4.71390677583113));
#76713=CARTESIAN_POINT('Ctrl Pts',(-7.52712967433642,5.5176381961095,-0.135819161248244));
#76714=CARTESIAN_POINT('Ctrl Pts',(-7.40786370191926,3.09931660075761,4.56694807458954));
#76715=CARTESIAN_POINT('Ctrl Pts',(-7.28859772950209,-2.1641235800721,5.07733662838151));
#76716=CARTESIAN_POINT('Ctrl Pts',(-7.16933175708492,-5.44093605806279,
0.926818709241918));
#76717=CARTESIAN_POINT('Ctrl Pts',(-7.05006578466777,-3.72306412807567,
-4.07450262068451));
#76718=CARTESIAN_POINT('Ctrl Pts',(-6.93079981225059,1.41251573892071,-5.33550160669358));
#76719=CARTESIAN_POINT('Ctrl Pts',(-6.81153383983344,5.25143079274477,-1.69860317223912));
#76720=CARTESIAN_POINT('Ctrl Pts',(-6.69226786741626,4.26962396706275,3.49758334963045));
#76721=CARTESIAN_POINT('Ctrl Pts',(-6.57300189499911,-0.631623195473639,
5.4830493565778));
#76722=CARTESIAN_POINT('Ctrl Pts',(-6.45373592258193,-4.95305128046833,
2.43517168199283));
#76723=CARTESIAN_POINT('Ctrl Pts',(-6.33446995016478,-4.72766467430163,
-2.8481511257462));
#76724=CARTESIAN_POINT('Ctrl Pts',(-6.2152039777476,-0.162364350551328,
-5.51692087358507));
#76725=CARTESIAN_POINT('Ctrl Pts',(-6.09593800533044,4.55198361526935,-3.12125347801937));
#76726=CARTESIAN_POINT('Ctrl Pts',(-5.97667203291329,5.0876900117107,2.13967017375761));
#76727=CARTESIAN_POINT('Ctrl Pts',(-5.85740606049611,0.952985709893719,
5.43641392320959));
#76728=CARTESIAN_POINT('Ctrl Pts',(-5.73814008807895,-4.05654285293957,
3.74262450561013));
#76729=CARTESIAN_POINT('Ctrl Pts',(-5.61887411566179,-5.34223582541585,
-1.38682893443001));
#76730=CARTESIAN_POINT('Ctrl Pts',(-5.49960814324461,-1.72384948209047,
-5.24319759982638));
#76731=CARTESIAN_POINT('Ctrl Pts',(-5.38034217082747,3.47700062078207,-4.28640231322372));
#76732=CARTESIAN_POINT('Ctrl Pts',(-5.26107619841028,5.48602479483962,0.605235539384232));
#76733=CARTESIAN_POINT('Ctrl Pts',(-5.14181022599314,2.45897388693394,4.94127772252337));
#76734=CARTESIAN_POINT('Ctrl Pts',(-5.02254425357596,-2.82537216313636,
4.74131313535636));
#76735=CARTESIAN_POINT('Ctrl Pts',(-4.9032782811588,-5.51607584370304,0.188905781395227));
#76736=CARTESIAN_POINT('Ctrl Pts',(-4.78401230874163,-3.14311810355895,
-4.53691378525191));
#76737=CARTESIAN_POINT('Ctrl Pts',(-4.66474633632447,2.11516723770901,-5.09792562364841));
#76738=CARTESIAN_POINT('Ctrl Pts',(-4.54548036390731,5.43176594459808,-0.979130650543266));
#76739=CARTESIAN_POINT('Ctrl Pts',(-4.42621439149014,3.76209824773743,4.0384891831104));
#76740=CARTESIAN_POINT('Ctrl Pts',(-4.30694841907298,-1.36111002720254,
5.34884638044292));
#76741=CARTESIAN_POINT('Ctrl Pts',(-4.18768244665581,-5.23484303577975,
1.74905588775117));
#76742=CARTESIAN_POINT('Ctrl Pts',(-4.06841647423865,-4.30308143644391,
-3.45633740526884));
#76743=CARTESIAN_POINT('Ctrl Pts',(-3.94915050182148,0.578833873119023,
-5.48887324093558));
#76744=CARTESIAN_POINT('Ctrl Pts',(-3.82988452940432,4.92938978238305,-2.48271917080172));
#76745=CARTESIAN_POINT('Ctrl Pts',(-3.71061855698715,4.75485184305665,2.80252779795483));
#76746=CARTESIAN_POINT('Ctrl Pts',(-3.59135258456999,0.215442839390763,
5.51510312602438));
#76747=CARTESIAN_POINT('Ctrl Pts',(-3.47208661215283,-4.52173893337813,
3.16490997124739));
#76748=CARTESIAN_POINT('Ctrl Pts',(-3.35282063973566,-5.10804322725765,
-2.09061533912767));
#76749=CARTESIAN_POINT('Ctrl Pts',(-3.2335546673185,-1.00525292597957,-5.42699222982105));
#76750=CARTESIAN_POINT('Ctrl Pts',(-3.11428869490133,4.02034202910876,-3.7814849036735));
#76751=CARTESIAN_POINT('Ctrl Pts',(-2.99502272248417,5.35533311875175,1.33535961258734));
#76752=CARTESIAN_POINT('Ctrl Pts',(-2.875756750067,1.77422180573573,5.2263672939988));
#76753=CARTESIAN_POINT('Ctrl Pts',(-2.75649077764984,-3.43559418140904,
4.31966095062996));
#76754=CARTESIAN_POINT('Ctrl Pts',(-2.63722480523267,-5.49159462892905,
-0.552418807831753));
#76755=CARTESIAN_POINT('Ctrl Pts',(-2.51795883281551,-2.50640698393315,
-4.91738773523297));
#76756=CARTESIAN_POINT('Ctrl Pts',(-2.39869286039835,2.77961855900976,-4.76828048400439));
#76757=CARTESIAN_POINT('Ctrl Pts',(-2.27942688798118,5.51400274306588,-0.241974910250199));
#76758=CARTESIAN_POINT('Ctrl Pts',(-2.16016091556402,3.18662857663998,4.5064594109201));
#76759=CARTESIAN_POINT('Ctrl Pts',(-2.04089494314685,-2.06601504634835,
5.11804258833305));
#76760=CARTESIAN_POINT('Ctrl Pts',(-1.92162897072969,-5.42209288938195,
1.03135193151629));
#76761=CARTESIAN_POINT('Ctrl Pts',(-1.80236299831252,-3.80078402465012,
-4.00210181101047));
#76762=CARTESIAN_POINT('Ctrl Pts',(-1.68309702589536,1.30957828666277,-5.3616958901853));
#76763=CARTESIAN_POINT('Ctrl Pts',(-1.56383105347819,5.21777057068265,-1.79934665349586));
#76764=CARTESIAN_POINT('Ctrl Pts',(-1.44456508106103,4.33614047199418,3.41477142937312));
#76765=CARTESIAN_POINT('Ctrl Pts',(-1.32529910864386,-0.525990954986324,
5.49418889582449));
#76766=CARTESIAN_POINT('Ctrl Pts',(-1.2060331362267,-4.90527185890021,2.53003677799559));
#76767=CARTESIAN_POINT('Ctrl Pts',(-1.08676716380953,-4.78159874734929,
-2.75664497661135));
#76768=CARTESIAN_POINT('Ctrl Pts',(-0.967501191392371,-0.268501379800935,
-5.51277472029953));
#76769=CARTESIAN_POINT('Ctrl Pts',(-0.848235218975206,4.49107557157286,
-3.20827341698774));
#76770=CARTESIAN_POINT('Ctrl Pts',(-0.72896924655804,5.12792347540635,2.04136692882621));
#76771=CARTESIAN_POINT('Ctrl Pts',(-0.609703274140877,1.05742706300564,
5.41706803669216));
#76772=CARTESIAN_POINT('Ctrl Pts',(-0.490437301723711,-3.98376895104567,
3.81999516392536));
#76773=CARTESIAN_POINT('Ctrl Pts',(-0.371171329306549,-5.36793454745627,
-1.28376664622291));
#76774=CARTESIAN_POINT('Ctrl Pts',(-0.251905356889381,-1.82442984943385,
-5.20905306483082));
#76775=CARTESIAN_POINT('Ctrl Pts',(-0.132639384472219,3.39386963117249,
-4.35251961906362));
#76776=CARTESIAN_POINT('Ctrl Pts',(-0.0133734120550536,5.49665598156906,
0.499550926342804));
#76777=CARTESIAN_POINT('Ctrl Pts',(0.105892560362111,2.55360800599929,4.89304243384675));
#76778=CARTESIAN_POINT('Ctrl Pts',(0.225158532779274,-2.73360758255891,
4.79480632479614));
#76779=CARTESIAN_POINT('Ctrl Pts',(0.344424505196442,-5.51141908615201,
0.295021634000305));
#76780=CARTESIAN_POINT('Ctrl Pts',(0.463690477613603,-3.22984399124939,
-4.4755877714462));
#76781=CARTESIAN_POINT('Ctrl Pts',(0.58295645003077,2.01667155712322,-5.13768565975176));
#76782=CARTESIAN_POINT('Ctrl Pts',(0.702222422447934,5.41191778806855,-1.08347771685263));
#76783=CARTESIAN_POINT('Ctrl Pts',(0.821488394865098,3.83911787679396,3.96534387358896));
#76784=CARTESIAN_POINT('Ctrl Pts',(0.940754367282264,-1.25792528876334,
5.37404894615022));
#76785=CARTESIAN_POINT('Ctrl Pts',(1.06002033969943,-5.20021497823882,1.84947081291638));
#76786=CARTESIAN_POINT('Ctrl Pts',(1.17928631211659,-4.36879801268882,-3.37288927064835));
#76787=CARTESIAN_POINT('Ctrl Pts',(1.29855228453375,0.473099333942919,-5.49899582905383));
#76788=CARTESIAN_POINT('Ctrl Pts',(1.41781825695092,4.88069974316303,-2.57712012231041));
#76789=CARTESIAN_POINT('Ctrl Pts',(1.53708422936808,4.80790291061196,2.71050691012911));
#76790=CARTESIAN_POINT('Ctrl Pts',(1.65635020178525,0.321535058949422,5.50993587200387));
#76791=CARTESIAN_POINT('Ctrl Pts',(1.77561617420242,-4.45999636905643,3.25133980010278));
#76792=CARTESIAN_POINT('Ctrl Pts',(1.89488214661958,-5.1473289153913,-1.99192950289544));
#76793=CARTESIAN_POINT('Ctrl Pts',(2.01414811903674,-1.10950329002883,-5.40664226273052));
#76794=CARTESIAN_POINT('Ctrl Pts',(2.13341409145391,3.94682700514964,-3.85815172059762));
#76795=CARTESIAN_POINT('Ctrl Pts',(2.25268006387108,5.38003894472928,1.23205481246771));
#76796=CARTESIAN_POINT('Ctrl Pts',(2.37194603628823,1.8744689642876,5.19125651549326));
#76797=CARTESIAN_POINT('Ctrl Pts',(2.4912120087054,-3.3518308334604,4.38497527605265));
#76798=CARTESIAN_POINT('Ctrl Pts',(2.61047798112256,-5.50120838411536,-0.446636790096184));
#76799=CARTESIAN_POINT('Ctrl Pts',(2.72974395353974,-2.6005725826633,-4.86824407256134));
#76800=CARTESIAN_POINT('Ctrl Pts',(2.84900992595689,2.68734349406327,-4.82088820163304));
#76801=CARTESIAN_POINT('Ctrl Pts',(2.96827589837406,5.50832511218907,-0.348041040907454));
#76802=CARTESIAN_POINT('Ctrl Pts',(3.08754187079122,3.27276034595634,4.44430172531797));
#76803=CARTESIAN_POINT('Ctrl Pts',(3.20680784320839,-1.96714133887937,5.1568530191));
#76804=CARTESIAN_POINT('Ctrl Pts',(3.32607381562555,-5.40124158279764,1.13550318008635));
#76805=CARTESIAN_POINT('Ctrl Pts',(3.44533978804272,-3.87709625473508,-3.92821877436172));
#76806=CARTESIAN_POINT('Ctrl Pts',(3.56460576045988,1.20615581619359,-5.38590440453517));
#76807=CARTESIAN_POINT('Ctrl Pts',(3.68387173287705,5.18217788396745,-1.8994237248827));
#76808=CARTESIAN_POINT('Ctrl Pts',(3.80313770529422,4.40105103467883,3.3306948070757));
#76809=CARTESIAN_POINT('Ctrl Pts',(3.92240367771138,-0.420163907365567,
5.50329359553678));
#76810=CARTESIAN_POINT('Ctrl Pts',(4.04166965012854,-4.85567571036938,2.6239648441733));
#76811=CARTESIAN_POINT('Ctrl Pts',(4.1609356225457,-4.83376189727187,-2.66411787055516));
#76812=CARTESIAN_POINT('Ctrl Pts',(4.28020159496287,-0.374538966305925,
-5.50658684399396));
#76813=CARTESIAN_POINT('Ctrl Pts',(4.39946756738004,4.42850420353529,-3.29410513296082));
#76814=CARTESIAN_POINT('Ctrl Pts',(4.5187335397972,5.16625775041094,1.94230763887896));
#76815=CARTESIAN_POINT('Ctrl Pts',(4.63799951221437,1.16147678517189,5.39571587328648));
#76816=CARTESIAN_POINT('Ctrl Pts',(4.75726548463153,-3.90951961197424,3.89595104067253));
#76817=CARTESIAN_POINT('Ctrl Pts',(4.8765314570487,-5.39164518979235,-1.1802288994588));
#76818=CARTESIAN_POINT('Ctrl Pts',(4.99579742946586,-1.92433451704137,-5.17297929381628));
#76819=CARTESIAN_POINT('Ctrl Pts',(5.11506340188302,3.30948168075747,-4.41702491644086));
#76820=CARTESIAN_POINT('Ctrl Pts',(5.23432937430019,5.5052514150489,0.393681298553378));
#76821=CARTESIAN_POINT('Ctrl Pts',(5.35359534671735,2.64729636534932,4.84299494752337));
#76822=CARTESIAN_POINT('Ctrl Pts',(5.47286131913452,-2.64083057723855,4.84652369952428));
#76823=CARTESIAN_POINT('Ctrl Pts',(5.59212729155168,-5.50472110765647,0.40102822176287));
#76824=CARTESIAN_POINT('Ctrl Pts',(5.71139326396885,-3.31537366702065,-4.41260416939415));
#76825=CARTESIAN_POINT('Ctrl Pts',(5.83065923638601,1.9174289777522,-5.17554289162062));
#76826=CARTESIAN_POINT('Ctrl Pts',(5.94992520880318,5.39006526210777,-1.18742350404059));
#76827=CARTESIAN_POINT('Ctrl Pts',(6.06919118122034,3.91471564195373,3.89072995084103));
#76828=CARTESIAN_POINT('Ctrl Pts',(6.18845715363751,-1.15427466242746,5.39726116761145));
#76829=CARTESIAN_POINT('Ctrl Pts',(6.30772312605466,-5.16366095797147,1.94920076412104));
#76830=CARTESIAN_POINT('Ctrl Pts',(6.42698909847183,-4.43289655157051,-3.28819194555351));
#76831=CARTESIAN_POINT('Ctrl Pts',(6.546255070889,0.367189576687042,-5.50708179733159));
#76832=CARTESIAN_POINT('Ctrl Pts',(6.66552104330615,4.83020207756152,-2.67056660610614));
#76833=CARTESIAN_POINT('Ctrl Pts',(6.78478701572333,4.85917331297616,2.61748215317485));
#76834=CARTESIAN_POINT('Ctrl Pts',(6.90405298814047,0.427508194096852,5.50272794636521));
#76835=CARTESIAN_POINT('Ctrl Pts',(7.02331896055767,-4.39660199095344,3.3365654558053));
#76836=CARTESIAN_POINT('Ctrl Pts',(7.14258493297481,-5.18470822779373,-1.89250593139799));
#76837=CARTESIAN_POINT('Ctrl Pts',(7.26185090539199,-1.21334273606982,-5.38428988006359));
#76838=CARTESIAN_POINT('Ctrl Pts',(7.38111687780915,3.87185022591093,-3.93338962420994));
#76839=CARTESIAN_POINT('Ctrl Pts',(7.50038285022631,5.40275220799211,1.12829370589621));
#76840=CARTESIAN_POINT('Ctrl Pts',(7.61964882264348,1.97402189051019,5.1542230921367));
#76841=CARTESIAN_POINT('Ctrl Pts',(7.73891479506064,-3.26682609428515,4.44866557266632));
#76842=CARTESIAN_POINT('Ctrl Pts',(7.8581807674778,-5.50878470001459,-0.34068935500509));
#76843=CARTESIAN_POINT('Ctrl Pts',(7.97744673989498,-2.69377502777718,-4.81729739661697));
#76844=CARTESIAN_POINT('Ctrl Pts',(8.09671271231213,2.5940731388404,-4.87171044481049));
#76845=CARTESIAN_POINT('Ctrl Pts',(8.21597868472929,5.50060740625855,-0.453978270341479));
#76846=CARTESIAN_POINT('Ctrl Pts',(8.33524465714647,3.35768000876078,4.38049803863634));
#76847=CARTESIAN_POINT('Ctrl Pts',(8.45451062956363,-1.86753907674248,5.19375354676834));
#76848=CARTESIAN_POINT('Ctrl Pts',(8.57377660198079,-5.37838986084429,1.23923388127339));
#76849=CARTESIAN_POINT('Ctrl Pts',(8.69304257439796,-3.95197255517013,-3.85288087421746));
#76850=CARTESIAN_POINT('Ctrl Pts',(8.81230854681512,1.10228663128005,-5.40811818382607));
#76851=CARTESIAN_POINT('Ctrl Pts',(8.93157451923229,5.14466591478258,-1.99879732164191));
#76852=CARTESIAN_POINT('Ctrl Pts',(9.05084049164945,4.46433161470217,3.24538462153554));
#76853=CARTESIAN_POINT('Ctrl Pts',(9.17010646406662,-0.314181246942596,
5.51036008367861));
#76854=CARTESIAN_POINT('Ctrl Pts',(9.28937243648378,-4.80428120341128,2.71692109312688));
#76855=CARTESIAN_POINT('Ctrl Pts',(9.40863840890095,-4.88413480481383,-2.57060407611415));
#76856=CARTESIAN_POINT('Ctrl Pts',(9.52790438131811,-0.480437837759446,
-5.49835953642338));
#76857=CARTESIAN_POINT('Ctrl Pts',(9.64717035373527,4.36429268522211,-3.37871683712107));
#76858=CARTESIAN_POINT('Ctrl Pts',(9.76643632615244,5.20267863916058,1.842528991726));
#76859=CARTESIAN_POINT('Ctrl Pts',(9.8857022985696,1.26509634031525,5.3723653410253));
#76860=CARTESIAN_POINT('Ctrl Pts',(10.0049682709868,-3.83382233486901,3.97046400467101));
#76861=CARTESIAN_POINT('Ctrl Pts',(10.1242342434039,-5.41335897090002,-1.07625404059861));
#76862=CARTESIAN_POINT('Ctrl Pts',(10.2435002158211,-2.02352648400704,-5.13498964714156));
#76863=CARTESIAN_POINT('Ctrl Pts',(10.3627661882383,3.22386802363844,-4.47989431503581));
#76864=CARTESIAN_POINT('Ctrl Pts',(10.4820321606554,5.5118079118561,0.287665866117311));
#76865=CARTESIAN_POINT('Ctrl Pts',(10.6012981330726,2.74000426636313,4.7911537992472));
#76866=CARTESIAN_POINT('Ctrl Pts',(10.7205641054897,-2.54707550826514,4.89644610538342));
#76867=CARTESIAN_POINT('Ctrl Pts',(10.8398300779069,-5.495984388894,0.506886283856618));
#76868=CARTESIAN_POINT('Ctrl Pts',(10.9590960503241,-3.39967545391932,-4.34798630583716));
#76869=CARTESIAN_POINT('Ctrl Pts',(11.0783620227413,1.81747625528963,-5.21148329836976));
#76870=CARTESIAN_POINT('Ctrl Pts',(11.1976279951584,5.36621646006394,-1.29092951452332));
#76871=CARTESIAN_POINT('Ctrl Pts',(11.3168939675756,3.98886354466695,3.81467504903838));
#76872=CARTESIAN_POINT('Ctrl Pts',(11.4361599399927,-1.05019653646226,5.41847444789871));
#76873=CARTESIAN_POINT('Ctrl Pts',(11.5554259124099,-5.12519451320274,2.04820880516737));
#76874=CARTESIAN_POINT('Ctrl Pts',(11.6746918848271,-4.49535331341717,-3.20227679866655));
#76875=CARTESIAN_POINT('Ctrl Pts',(11.7939578572442,0.261143826315328,-5.51312815103241));
#76876=CARTESIAN_POINT('Ctrl Pts',(11.9132238296614,4.77791548800185,-2.76302401314953));
#76877=CARTESIAN_POINT('Ctrl Pts',(12.0324898020786,4.90864406153351,2.5234879799398));
#76878=CARTESIAN_POINT('Ctrl Pts',(12.1517557744957,0.533322996396297,5.49348201865112));
#76879=CARTESIAN_POINT('Ctrl Pts',(12.2710217469129,-4.3315792779465,3.42055537399901));
#76880=CARTESIAN_POINT('Ctrl Pts',(12.3902877193301,-5.22016732058297,-1.79238144736173));
#76881=CARTESIAN_POINT('Ctrl Pts',(12.5095536917472,-1.3167328059034,-5.35994336029645));
#76882=CARTESIAN_POINT('Ctrl Pts',(12.6288196641644,3.79543945995277,-4.00717074923971));
#76883=CARTESIAN_POINT('Ctrl Pts',(12.7480856365815,5.42346449640753,1.02411472205801));
#76884=CARTESIAN_POINT('Ctrl Pts',(12.8673516089987,2.07284371376895,5.115280739707));
#76885=CARTESIAN_POINT('Ctrl Pts',(12.9866175814159,-3.18061144642024,4.51070825199652));
#76886=CARTESIAN_POINT('Ctrl Pts',(13.1058835538331,-5.51432077064615,-0.234615741476998));
#76887=CARTESIAN_POINT('Ctrl Pts',(13.2251495262502,-2.78597980061803,-4.76456657611972));
#76888=CARTESIAN_POINT('Ctrl Pts',(13.3444154986674,2.49984203714938,-4.92072839090208));
#76889=CARTESIAN_POINT('Ctrl Pts',(13.4636814710845,5.49085248362037,-0.55974736341345));
#76890=CARTESIAN_POINT('Ctrl Pts',(13.5829474435017,3.44135611402541,4.31507198134501));
#76891=CARTESIAN_POINT('Ctrl Pts',(13.7022134159189,-1.76724514884449,5.22873050477977));
#76892=CARTESIAN_POINT('Ctrl Pts',(13.8214793883361,-5.35354618693448,1.34250561715309));
#76893=CARTESIAN_POINT('Ctrl Pts',(13.9407453607532,-4.02538519460857,-3.77611601288347));
#76894=CARTESIAN_POINT('Ctrl Pts',(14.0600113331704,0.998009201135608,-5.42832900091525));
#76895=CARTESIAN_POINT('Ctrl Pts',(14.1792773055875,5.10524855614116,-2.09743063955568));
#76896=CARTESIAN_POINT('Ctrl Pts',(14.2985432780047,4.52595877533329,3.15887246841535));
#76897=CARTESIAN_POINT('Ctrl Pts',(14.4178092504219,-0.208082225682183,
5.51538574309033));
#76898=CARTESIAN_POINT('Ctrl Pts',(14.537075222839,-4.75110737260535,2.80887109738119));
#76899=CARTESIAN_POINT('Ctrl Pts',(14.6563411952562,-4.93269881375749,-2.47613822725719));
#76900=CARTESIAN_POINT('Ctrl Pts',(14.7756071676734,-0.586158773228975,
-5.48809584467104));
#76901=CARTESIAN_POINT('Ctrl Pts',(14.8948731400905,4.29846479814849,-3.46207719249681));
#76902=CARTESIAN_POINT('Ctrl Pts',(15.0141391125077,5.23717265273706,1.74206794160044));
#76903=CARTESIAN_POINT('Ctrl Pts',(15.1334050849249,1.36824735167569,5.34702508806171));
#76904=CARTESIAN_POINT('Ctrl Pts',(15.252671057342,-3.75670515513534,4.04350645914012));
#76905=CARTESIAN_POINT('Ctrl Pts',(15.3719370297592,-5.43306784881692,-0.971880577993402));
#76906=CARTESIAN_POINT('Ctrl Pts',(15.4912030021763,-2.12196901338186,-5.09509819473345));
#76907=CARTESIAN_POINT('Ctrl Pts',(15.6104689745935,3.13706036787251,-4.54110453040358));
#76908=CARTESIAN_POINT('Ctrl Pts',(15.7297349470107,5.51632304371251,0.181543893136862));
#76909=CARTESIAN_POINT('Ctrl Pts',(15.8490009194278,2.83169737354434,4.73753818901663));
#76910=CARTESIAN_POINT('Ctrl Pts',(15.968266891845,-2.45237709896633,4.94455505300465));
#76911=CARTESIAN_POINT('Ctrl Pts',(16.0875328642621,-5.48521216561456,0.612556614463475));
#76912=CARTESIAN_POINT('Ctrl Pts',(16.2067988366793,-3.4827181297554,-4.28175811278522));
#76913=CARTESIAN_POINT('Ctrl Pts',(16.3260648090965,1.71685040843935,-5.24549356903332));
#76914=CARTESIAN_POINT('Ctrl Pts',(16.4453307815136,5.34038021463043,-1.39395741359364));
#76915=CARTESIAN_POINT('Ctrl Pts',(16.5645967539308,4.06153412335787,3.73720733603697));
#76916=CARTESIAN_POINT('Ctrl Pts',(16.683862726348,-0.945729457464844,5.43768093041616));
#76917=CARTESIAN_POINT('Ctrl Pts',(16.8031286987652,-5.08482989044738,2.14645826722576));
#76918=CARTESIAN_POINT('Ctrl Pts',(16.9223946711823,-4.55614516660902,-3.11517564970488));
#76919=CARTESIAN_POINT('Ctrl Pts',(17.0416606435995,0.155001358158474,-5.51713265081576));
#76920=CARTESIAN_POINT('Ctrl Pts',(17.1609266160166,4.723859339457,-2.85445810071785));
#76921=CARTESIAN_POINT('Ctrl Pts',(17.2801925884338,4.9562968341919,2.42855920230665));
#76922=CARTESIAN_POINT('Ctrl Pts',(17.399458560851,0.63894027605163,5.48220151320319));
#76923=CARTESIAN_POINT('Ctrl Pts',(17.5187245332682,-4.26495231198646,3.50327844799843));
#76924=CARTESIAN_POINT('Ctrl Pts',(17.6379905056853,-5.25369306105365,-1.69159313310433));
#76925=CARTESIAN_POINT('Ctrl Pts',(17.7572564781025,-1.41963520776255,-5.33361172045822));
#76926=CARTESIAN_POINT('Ctrl Pts',(17.8765224505196,3.71762300692966,-4.07946776995188));
#76927=CARTESIAN_POINT('Ctrl Pts',(17.9957884229368,5.44216813892813,0.919556444903994));
#76928=CARTESIAN_POINT('Ctrl Pts',(18.115054395354,2.17089783420263,5.07444388097677));
#76929=CARTESIAN_POINT('Ctrl Pts',(18.2343203677711,-3.09321882050645,4.57108033578427));
#76930=CARTESIAN_POINT('Ctrl Pts',(18.3535863401883,-5.51781454565922,-0.128455235161643));
#76931=CARTESIAN_POINT('Ctrl Pts',(18.4728523126055,-2.87715275202947,-4.71007114056864));
#76932=CARTESIAN_POINT('Ctrl Pts',(18.5921182850226,2.40468508862193,-4.96792388551679));
#76933=CARTESIAN_POINT('Ctrl Pts',(18.7113842574398,5.4790639571286,-0.665309147256506));
#76934=CARTESIAN_POINT('Ctrl Pts',(18.830650229857,3.52375767128937,4.24804778477804));
#76935=CARTESIAN_POINT('Ctrl Pts',(18.9499162022741,-1.66629670025835,5.26177093899355));
#76936=CARTESIAN_POINT('Ctrl Pts',(19.0691821746913,-5.32671976222436,1.44528013978514));
#76937=CARTESIAN_POINT('Ctrl Pts',(19.1884481471084,-4.09730698378862,-3.69795262115746));
#76938=CARTESIAN_POINT('Ctrl Pts',(19.3077141195256,0.893362146171608,-5.4465293704814));
#76939=CARTESIAN_POINT('Ctrl Pts',(19.4269800919428,5.06394040674028,-2.19528714857806));
#76940=CARTESIAN_POINT('Ctrl Pts',(19.5462460643599,4.58590969220547,3.07119038854062));
#76941=CARTESIAN_POINT('Ctrl Pts',(19.6655120367771,-0.101906138644027,
5.51836871245802));
#76942=CARTESIAN_POINT('Ctrl Pts',(19.7847780091943,-4.69617391152509,2.89978080213661));
#76943=CARTESIAN_POINT('Ctrl Pts',(19.9040439816114,-4.97943593783279,-2.38075531055748));
#76944=CARTESIAN_POINT('Ctrl Pts',(20.0233099540286,-0.691662617683489,
-5.47579957001972));
#76945=CARTESIAN_POINT('Ctrl Pts',(20.1425759264457,4.23104492247119,-3.54415532556908));
#76946=CARTESIAN_POINT('Ctrl Pts',(20.2618418988629,5.26972701586384,1.64096169547102));
#76947=CARTESIAN_POINT('Ctrl Pts',(20.3811078712801,1.47089161602474,5.31970449946583));
#76948=CARTESIAN_POINT('Ctrl Pts',(20.5003738436973,-3.67819663405649,4.1150513519207));
#76949=CARTESIAN_POINT('Ctrl Pts',(20.6196398161144,-5.45076452412087,-0.867147167621348));
#76950=CARTESIAN_POINT('Ctrl Pts',(20.7389057885316,-2.21962564578078,-5.05331971087533));
#76951=CARTESIAN_POINT('Ctrl Pts',(20.8581717609487,3.04909086372826,-4.60063289259834));
#76952=CARTESIAN_POINT('Ctrl Pts',(20.9774377333659,5.51879513838413,0.0753546831722458));
#76953=CARTESIAN_POINT('Ctrl Pts',(21.0967037057831,2.92234172723827,4.68216797402346));
#76954=CARTESIAN_POINT('Ctrl Pts',(21.2159696782002,-2.35677042204708,4.99083272465557));
#76955=CARTESIAN_POINT('Ctrl Pts',(21.3352356506174,-5.47240842744157,0.718000077294374));
#76956=CARTESIAN_POINT('Ctrl Pts',(21.4545016230345,-3.56447093866641,-4.21394411865316));
#76957=CARTESIAN_POINT('Ctrl Pts',(21.5737675954518,1.6155887052047,-5.27756110749501));
#76958=CARTESIAN_POINT('Ctrl Pts',(21.6930335678689,5.31256609457409,-1.49646904361904));
#76959=CARTESIAN_POINT('Ctrl Pts',(21.8122995402861,4.13270046359602,3.6583555029442));
#76960=CARTESIAN_POINT('Ctrl Pts',(21.9315655127032,-0.840912116085472,
5.45487350181007));
#76961=CARTESIAN_POINT('Ctrl Pts',(22.0508314851204,-5.04258203923305,2.2439127624158));
#76962=CARTESIAN_POINT('Ctrl Pts',(22.1700974575376,-4.61524959614565,-3.02692075763577));
#76963=CARTESIAN_POINT('Ctrl Pts',(22.2893634299547,0.048801483367409,-5.51909381356669));
#76964=CARTESIAN_POINT('Ctrl Pts',(22.4086294023719,4.66805365227747,-2.94483500508725));
#76965=CARTESIAN_POINT('Ctrl Pts',(22.527895374789,5.00211398216874,2.33273097830009));
#76966=CARTESIAN_POINT('Ctrl Pts',(22.6471613472062,0.744320916421722,5.46889060789352));
#76967=CARTESIAN_POINT('Ctrl Pts',(22.7664273196234,-4.1967457691786,3.58470404030929));
#76968=CARTESIAN_POINT('Ctrl Pts',(22.8856932920405,-5.28527303254098,-1.59017831680098));
#76969=CARTESIAN_POINT('Ctrl Pts',(23.0049592644577,-1.52201183049409,-5.30530471279124));
#76970=CARTESIAN_POINT('Ctrl Pts',(23.1242252368749,3.63842968710919,-4.15025391026752));
#76971=CARTESIAN_POINT('Ctrl Pts',(23.243491209292,5.45885620843297,0.81465759886084));
#76972=CARTESIAN_POINT('Ctrl Pts',(23.3627571817092,2.26814793627769,5.03172764037246));
#76973=CARTESIAN_POINT('Ctrl Pts',(23.4820231541264,-3.00468058346354,4.62975946449548));
#76974=CARTESIAN_POINT('Ctrl Pts',(23.6012891265435,-5.51926473109169,-0.0222471538909869));
#76975=CARTESIAN_POINT('Ctrl Pts',(23.7205550989607,-2.96726011500245,-4.65383127300986));
#76976=CARTESIAN_POINT('Ctrl Pts',(23.8398210713778,2.30863753578895,-5.01327944923028));
#76977=CARTESIAN_POINT('Ctrl Pts',(23.959087043795,5.46524619280696,-0.77062452578279));
#76978=CARTESIAN_POINT('Ctrl Pts',(24.0783530162122,3.60485416213592,4.17945027216024));
#76979=CARTESIAN_POINT('Ctrl Pts',(24.1976189886294,-1.56473111846732,5.29286261248375));
#76980=CARTESIAN_POINT('Ctrl Pts',(24.3168849610465,-5.29792052220578,1.5475193853777));
#76981=CARTESIAN_POINT('Ctrl Pts',(24.4361509334637,-4.16771128560285,-3.61841964780034));
#76982=CARTESIAN_POINT('Ctrl Pts',(24.5554169058808,0.788384223695067,-5.46271255179668));
#76983=CARTESIAN_POINT('Ctrl Pts',(24.6746828782981,5.0207567655543,-2.29233060636324));
#76984=CARTESIAN_POINT('Ctrl Pts',(24.7939488507152,4.64416216176915,2.98237085603393));
#76985=CARTESIAN_POINT('Ctrl Pts',(24.9132148231324,0.00430769056925928,
5.51930788700271));
#76986=CARTESIAN_POINT('Ctrl Pts',(25.0324807955495,-4.63950116544441,2.98961653788056));
#76987=CARTESIAN_POINT('Ctrl Pts',(25.1517467679667,-5.02432886737874,-2.28449065223597));
#76988=CARTESIAN_POINT('Ctrl Pts',(25.2710127403838,-0.796910296493555,
-5.46147526654391));
#76989=CARTESIAN_POINT('Ctrl Pts',(25.390278712801,4.1620580279593,-3.62492083770507));
#76990=CARTESIAN_POINT('Ctrl Pts',(25.5095446852181,5.3003296716376,1.53924769926319));
#76991=CARTESIAN_POINT('Ctrl Pts',(25.6288106576354,1.57299111781316,5.29041369374921));
#76992=CARTESIAN_POINT('Ctrl Pts',(25.7480766300525,-3.59832584821597,4.18507218549331));
#76993=CARTESIAN_POINT('Ctrl Pts',(25.8673426024697,-5.46644244263356,-0.762092598772189));
#76994=CARTESIAN_POINT('Ctrl Pts',(25.9866085748868,-2.31646021288461,-5.00966966873574));
#76995=CARTESIAN_POINT('Ctrl Pts',(26.105874547304,2.95999209177915,-4.65845735456855));
#76996=CARTESIAN_POINT('Ctrl Pts',(26.2251405197212,5.5192232803009,-0.0308624353137705));
#76997=CARTESIAN_POINT('Ctrl Pts',(26.3444064921383,3.01190375620826,4.62506366129882));
#76998=CARTESIAN_POINT('Ctrl Pts',(26.4636724645555,-2.26029088660046,5.03526198083872));
#76999=CARTESIAN_POINT('Ctrl Pts',(26.5829384369726,-5.45757791639507,0.823177620083097));
#77000=CARTESIAN_POINT('Ctrl Pts',(26.7022044093898,-3.6449036025072,-4.1445694391768));
#77001=CARTESIAN_POINT('Ctrl Pts',(26.821470381807,1.51372864908642,-5.30767403715261));
#77002=CARTESIAN_POINT('Ctrl Pts',(26.9407363542241,5.28278440119203,-1.59842643817319));
#77003=CARTESIAN_POINT('Ctrl Pts',(27.0600023266413,4.20233620806344,3.57814875349353));
#77004=CARTESIAN_POINT('Ctrl Pts',(27.1792682990585,-0.735783332698646,
5.47004579460281));
#77005=CARTESIAN_POINT('Ctrl Pts',(27.2985342714756,-4.9984666065644,2.34053619728246));
#77006=CARTESIAN_POINT('Ctrl Pts',(27.4178002438929,-4.67264471198416,-2.93754480872971));
#77007=CARTESIAN_POINT('Ctrl Pts',(27.5370662163099,-0.0574164656453142,
-5.51901091294461));
#77008=CARTESIAN_POINT('Ctrl Pts',(27.6563321887272,4.61051909477695,-3.0341212540744));
#77009=CARTESIAN_POINT('Ctrl Pts',(27.7755981611443,5.04607853652714,2.23603879906599));
#77010=CARTESIAN_POINT('Ctrl Pts',(27.8948641335615,0.849425888507462,5.45355423257733));
#77011=CARTESIAN_POINT('Ctrl Pts',(28.0141301059786,-4.126984910644,3.66480199397535));
#77012=CARTESIAN_POINT('Ctrl Pts',(28.1333960783958,-5.31489553901918,-1.48817455865981));
#77013=CARTESIAN_POINT('Ctrl Pts',(28.252662050813,-1.62382475767335,-5.27503282113916));
#77014=CARTESIAN_POINT('Ctrl Pts',(28.3719280232301,3.5578888306985,-4.21950295368066));
#77015=CARTESIAN_POINT('Ctrl Pts',(28.4911939956473,5.47352252429297,0.709457034489319));
#77016=CARTESIAN_POINT('Ctrl Pts',(28.6104599680644,2.36455800223863,4.9871478383719));
#77017=CARTESIAN_POINT('Ctrl Pts',(28.7297259404816,-2.91502952650204,4.68672390560296));
#77018=CARTESIAN_POINT('Ctrl Pts',(28.8489919128988,-5.51867078984984,0.0839691668831474));
#77019=CARTESIAN_POINT('Ctrl Pts',(28.9682578853159,-3.05626851718156,-4.59586780256059));
#77020=CARTESIAN_POINT('Ctrl Pts',(29.0875238577331,2.21173495102714,-5.05677828405932));
#77021=CARTESIAN_POINT('Ctrl Pts',(29.2067898301503,5.4494043082322,-0.875654494163783));
#77022=CARTESIAN_POINT('Ctrl Pts',(29.3260558025674,3.68461555149545,4.10930484941263));
#77023=CARTESIAN_POINT('Ctrl Pts',(29.4453217749846,-1.46258601951706,5.32199401007199));
#77024=CARTESIAN_POINT('Ctrl Pts',(29.5645877474018,-5.26715913302683,1.64918548838541));
#77025=CARTESIAN_POINT('Ctrl Pts',(29.6838537198189,-4.2365720249636,-3.53754654881376));
#77026=CARTESIAN_POINT('Ctrl Pts',(29.8031196922361,0.683114313553423,-5.47687255122367));
#77027=CARTESIAN_POINT('Ctrl Pts',(29.9223856646533,4.97571362616884,-2.38852507168894));
#77028=CARTESIAN_POINT('Ctrl Pts',(30.0416516370704,4.70069460951519,2.89244676628684));
#77029=CARTESIAN_POINT('Ctrl Pts',(30.1609176094876,0.11051992437719,5.51820291888986));
#77030=CARTESIAN_POINT('Ctrl Pts',(30.2801835819047,-4.58111012380261,3.0783450328581));
#77031=CARTESIAN_POINT('Ctrl Pts',(30.3994495543219,-5.06736097575394,-2.18737990507693));
#77032=CARTESIAN_POINT('Ctrl Pts',(30.518715526739,-0.901862829904248,-5.44512823942338));
#77033=CARTESIAN_POINT('Ctrl Pts',(30.6379814991563,4.09152966474647,-3.70434381641723));
#77034=CARTESIAN_POINT('Ctrl Pts',(30.7572474715734,5.3289692859932,1.43696362398964));
#77035=CARTESIAN_POINT('Ctrl Pts',(30.8765134439906,1.67450804325163,5.25916351911732));
#77036=CARTESIAN_POINT('Ctrl Pts',(30.9957794164077,-3.51712237872867,4.25354302679248));
#77037=CARTESIAN_POINT('Ctrl Pts',(31.1150453888249,-5.48009579784741,-0.656755779680257));
#77038=CARTESIAN_POINT('Ctrl Pts',(31.2343113612421,-2.41243685083647,-4.9641642346376));
#77039=CARTESIAN_POINT('Ctrl Pts',(31.3535773336592,2.8697970508367,-4.71455650032301));
#77040=CARTESIAN_POINT('Ctrl Pts',(31.4728433060764,5.51760731089503,-0.137068123522462));
#77041=CARTESIAN_POINT('Ctrl Pts',(31.5921092784935,3.10035029007019,4.566246400118));
#77042=CARTESIAN_POINT('Ctrl Pts',(31.7113752509108,-2.1629742249933,5.07782636663992));
#77043=CARTESIAN_POINT('Ctrl Pts',(31.8306412233279,-5.44072612513458,0.928050289050349));
#77044=CARTESIAN_POINT('Ctrl Pts',(31.949907195745,-3.72398633206484,-4.07365976811063));
#77045=CARTESIAN_POINT('Ctrl Pts',(32.0691731681622,1.41130796519246,-5.33582120531725));
#77046=CARTESIAN_POINT('Ctrl Pts',(32.1884391405794,5.25104616449558,-1.69979183609775));
#77047=CARTESIAN_POINT('Ctrl Pts',(32.3077051129965,4.27041556631729,3.49661679322797));
#77048=CARTESIAN_POINT('Ctrl Pts',(32.4269710854137,-0.630382043025125,
5.48319218955167));
#77049=CARTESIAN_POINT('Ctrl Pts',(32.5462370578309,-4.95249993112703,2.43629278616405));
#77050=CARTESIAN_POINT('Ctrl Pts',(32.6655030302481,-4.72830925714705,-2.84708090445397));
#77051=CARTESIAN_POINT('Ctrl Pts',(32.7847690026652,-0.163613149773239,
-5.51688397965284));
#77052=CARTESIAN_POINT('Ctrl Pts',(32.9040349750824,4.5512769755768,-3.12228377943339));
#77053=CARTESIAN_POINT('Ctrl Pts',(33.0233009474995,5.08817421446106,2.13851847572625));
#77054=CARTESIAN_POINT('Ctrl Pts',(33.1425669199167,0.954216265406902,5.4361980672674));
#77055=CARTESIAN_POINT('Ctrl Pts',(33.2618328923338,-4.05569557316294,3.74354264374733));
#77056=CARTESIAN_POINT('Ctrl Pts',(33.381098864751,-5.3425496094337,-1.38561963701042));
#77057=CARTESIAN_POINT('Ctrl Pts',(33.5003648371682,-1.72503628164692,-5.24280725706473));
#77058=CARTESIAN_POINT('Ctrl Pts',(33.6196308095854,3.47603026698121,-4.28718925296732));
#77059=CARTESIAN_POINT('Ctrl Pts',(33.7388967820025,5.48616165466014,0.603993714095214));
#77060=CARTESIAN_POINT('Ctrl Pts',(33.8581627544197,2.46009232544721,4.94072098564613));
#77061=CARTESIAN_POINT('Ctrl Pts',(33.9774287268369,-2.82429885297868,4.74195256163424));
#77062=CARTESIAN_POINT('Ctrl Pts',(34.096694699254,-5.51603294190759,0.190154388657318));
#77063=CARTESIAN_POINT('Ctrl Pts',(34.2159606716712,-3.14414499322367,-4.53620219669603));
#77064=CARTESIAN_POINT('Ctrl Pts',(34.3352266440883,2.11401322338287,-5.09840427968194));
#77065=CARTESIAN_POINT('Ctrl Pts',(34.4544926165055,5.43154417064249,-0.980360153276489));
#77066=CARTESIAN_POINT('Ctrl Pts',(34.5737585889227,3.7630122987619,4.03763749574514));
#77067=CARTESIAN_POINT('Ctrl Pts',(34.6930245613398,-1.35989923407058,5.34915434258951));
#77068=CARTESIAN_POINT('Ctrl Pts',(34.812290533757,-5.23444698756834,1.75024079553662));
#77069=CARTESIAN_POINT('Ctrl Pts',(34.9315565061742,-4.30386369840905,-3.45536327653838));
#77070=CARTESIAN_POINT('Ctrl Pts',(35.0508224785913,0.577591403638233,-5.48900412442188));
#77071=CARTESIAN_POINT('Ctrl Pts',(35.1700884510085,4.92882767104235,-2.48383491779139));
#77072=CARTESIAN_POINT('Ctrl Pts',(35.2893544234257,4.75548609761399,2.80145142382315));
#77073=CARTESIAN_POINT('Ctrl Pts',(35.4086203958428,0.216691226457424,5.51505421727112));
#77074=CARTESIAN_POINT('Ctrl Pts',(35.52788636826,-4.52102241369882,3.16593342555851));
#77075=CARTESIAN_POINT('Ctrl Pts',(35.6471523406772,-5.10851632308625,-2.08945903553642));
#77076=CARTESIAN_POINT('Ctrl Pts',(35.7664183130943,-1.00648135204571,-5.42676454238525));
#77077=CARTESIAN_POINT('Ctrl Pts',(35.8856842855115,4.01948596255725,-3.782394847567));
#77078=CARTESIAN_POINT('Ctrl Pts',(36.0049502579287,5.35563523539815,1.33414735393709));
#77079=CARTESIAN_POINT('Ctrl Pts',(36.1242162303458,1.77540482566106,5.22596554539102));
#77080=CARTESIAN_POINT('Ctrl Pts',(36.243482202763,-3.43461635982299,4.32043852452331));
#77081=CARTESIAN_POINT('Ctrl Pts',(36.3627481751802,-5.49171941999376,-0.551175737763215));
#77082=CARTESIAN_POINT('Ctrl Pts',(36.4820141475973,-2.50752022830702,-4.91682023424888));
#77083=CARTESIAN_POINT('Ctrl Pts',(36.6012801200145,2.77853955367696,-4.76890960570523));
#77084=CARTESIAN_POINT('Ctrl Pts',(36.7205460924316,5.51394705382706,-0.243222946520996));
#77085=CARTESIAN_POINT('Ctrl Pts',(36.8398120648488,3.18765004325205,4.50573778353591));
#77086=CARTESIAN_POINT('Ctrl Pts',(36.959078037266,-2.06485927485046,5.11851047989713));
#77087=CARTESIAN_POINT('Ctrl Pts',(37.0783440096832,-5.42185398584499,1.03257855562554));
#77088=CARTESIAN_POINT('Ctrl Pts',(37.1976099821003,-3.80169992186118,-4.00124006152411));
#77089=CARTESIAN_POINT('Ctrl Pts',(37.3168759545175,1.30838373881677,-5.36199466824331));
#77090=CARTESIAN_POINT('Ctrl Pts',(37.4361419269346,5.21732676183604,-1.80052298340626));
#77091=CARTESIAN_POINT('Ctrl Pts',(37.5554078993518,4.33698241739598,3.41378086864505));
#77092=CARTESIAN_POINT('Ctrl Pts',(37.6746738717689,-0.524878515764003,
5.4943248165015));
#77093=CARTESIAN_POINT('Ctrl Pts',(37.7939398441862,-4.9044497775631,2.53111477860059));
#77094=CARTESIAN_POINT('Ctrl Pts',(37.9132058166033,-4.78269608681437,-2.75550123298751));
#77095=CARTESIAN_POINT('Ctrl Pts',(38.0324717890204,-0.268849601375951,
-5.51283021355248));
#77096=CARTESIAN_POINT('Ctrl Pts',(38.1517377614376,4.48863752569352,-3.20906923476978));
#77097=CARTESIAN_POINT('Ctrl Pts',(38.2710037338548,5.13166198877306,2.03979046086845));
#77098=CARTESIAN_POINT('Ctrl Pts',(38.3902697062719,1.0522136396721,5.41758791291211));
#77099=CARTESIAN_POINT('Ctrl Pts',(38.4896580166196,-3.1319986375449,4.08605008372047));
#77100=CARTESIAN_POINT('Ctrl Pts',(38.5691686648977,-4.689252124851,1.26661108229022));
#77101=CARTESIAN_POINT('Ctrl Pts',(38.6089239890367,-4.72001247217602,-0.328601748833628));
#77102=CARTESIAN_POINT('Ctrl Pts',(38.6288016511063,-4.53940850365245,-1.08453452292322));
#77103=CARTESIAN_POINT('Ctrl Pts',(-17.7012016511063,-2.05512567986496,
4.34950232174947));
#77104=CARTESIAN_POINT('Ctrl Pts',(-17.6813239890368,-2.77943400182884,
4.00726899883239));
#77105=CARTESIAN_POINT('Ctrl Pts',(-17.6415686648977,-4.04231267840295,
2.95387391985648));
#77106=CARTESIAN_POINT('Ctrl Pts',(-17.5620580166196,-5.30524713465376,
-0.116410492754025));
#77107=CARTESIAN_POINT('Ctrl Pts',(-17.462669706272,-3.67778290240344,-4.33957689005188));
#77108=CARTESIAN_POINT('Ctrl Pts',(-17.3434037338548,1.66891228174828,-5.44172406759916));
#77109=CARTESIAN_POINT('Ctrl Pts',(-17.2241377614376,5.47488290767653,-1.53998020197864));
#77110=CARTESIAN_POINT('Ctrl Pts',(-17.1048717890205,4.25951367249169,3.77108835234815));
#77111=CARTESIAN_POINT('Ctrl Pts',(-16.9856058166033,-0.86837967644224,
5.62264033298406));
#77112=CARTESIAN_POINT('Ctrl Pts',(-16.8663398441862,-5.1978714987074,2.31150944439501));
#77113=CARTESIAN_POINT('Ctrl Pts',(-16.747073871769,-4.75646285723963,-3.12091671530309));
#77114=CARTESIAN_POINT('Ctrl Pts',(-16.6278078993518,0.051640530934677,
-5.6887274769557));
#77115=CARTESIAN_POINT('Ctrl Pts',(-16.5085419269346,4.81215727784529,-3.03421098473609));
#77116=CARTESIAN_POINT('Ctrl Pts',(-16.3892759545175,5.15529314801688,2.40556632308164));
#77117=CARTESIAN_POINT('Ctrl Pts',(-16.2700099821003,0.765909498650872,
5.63712411222854));
#77118=CARTESIAN_POINT('Ctrl Pts',(-16.1507440096831,-4.32653921855433,
3.69387479286789));
#77119=CARTESIAN_POINT('Ctrl Pts',(-16.031478037266,-5.4473143396903,-1.64027374325625));
#77120=CARTESIAN_POINT('Ctrl Pts',(-15.9122120648488,-1.56754255743221,
-5.4686866558594));
#77121=CARTESIAN_POINT('Ctrl Pts',(-15.7929460924317,3.75120208696408,-4.27693687578484));
#77122=CARTESIAN_POINT('Ctrl Pts',(-15.6736801200145,5.62641067462387,0.840964405285497));
#77123=CARTESIAN_POINT('Ctrl Pts',(-15.5544141475974,2.33667131925813,5.18687606040634));
#77124=CARTESIAN_POINT('Ctrl Pts',(-15.4351481751802,-3.09809098985903,
4.77132541153072));
#77125=CARTESIAN_POINT('Ctrl Pts',(-15.315882202763,-5.68886010004097,-0.0242184643975601));
#77126=CARTESIAN_POINT('Ctrl Pts',(-15.1966162303458,-3.05735469922997,
-4.79753036288636));
#77127=CARTESIAN_POINT('Ctrl Pts',(-15.0773502579287,2.38074891093858,-5.1667929809382));
#77128=CARTESIAN_POINT('Ctrl Pts',(-14.9580842855115,5.63336658597595,-0.793029796302506));
#77129=CARTESIAN_POINT('Ctrl Pts',(-14.8388183130943,3.71465196168976,4.30872093236743));
#77130=CARTESIAN_POINT('Ctrl Pts',(-14.7195523406772,-1.61404836555687,
5.45514098034502));
#77131=CARTESIAN_POINT('Ctrl Pts',(-14.60028636826,-5.46108044956259,1.59383675552073));
#77132=CARTESIAN_POINT('Ctrl Pts',(-14.4810203958429,-4.29493592219251,
-3.73058181656837));
#77133=CARTESIAN_POINT('Ctrl Pts',(-14.3617544234257,0.813884873630489,
-5.63039134303743));
#77134=CARTESIAN_POINT('Ctrl Pts',(-14.2424884510085,5.17557355104494,-2.36159981502903));
#77135=CARTESIAN_POINT('Ctrl Pts',(-14.1232224785913,4.7861759733498,3.07509915586776));
#77136=CARTESIAN_POINT('Ctrl Pts',(-14.0039565061742,0.00315232627448166,
5.68891073308194));
#77137=CARTESIAN_POINT('Ctrl Pts',(-13.884690533757,-4.78276510147707,3.08040147561366));
#77138=CARTESIAN_POINT('Ctrl Pts',(-13.7654245613399,-5.17818758041288,
-2.35586261241017));
#77139=CARTESIAN_POINT('Ctrl Pts',(-13.6461585889227,-0.820124171393288,
-5.62948590992118));
#77140=CARTESIAN_POINT('Ctrl Pts',(-13.5268926165055,4.29079892350715,-3.73533932389453));
#77141=CARTESIAN_POINT('Ctrl Pts',(-13.4076266440884,5.46284344083135,1.58778361482599));
#77142=CARTESIAN_POINT('Ctrl Pts',(-13.2883606716712,1.62009295488011,5.45334888706914));
#77143=CARTESIAN_POINT('Ctrl Pts',(-13.169094699254,-3.70987460822074,4.3128349907969));
#77144=CARTESIAN_POINT('Ctrl Pts',(-13.0498287268369,-5.63424198350418,
-0.786786208491855));
#77145=CARTESIAN_POINT('Ctrl Pts',(-12.9305627544197,-2.38647348263151,
-5.16415139042731));
#77146=CARTESIAN_POINT('Ctrl Pts',(-12.8112967820026,3.05203605370893,-4.80091566197721));
#77147=CARTESIAN_POINT('Ctrl Pts',(-12.6920308095854,5.68882972215975,-0.0305230868001199));
#77148=CARTESIAN_POINT('Ctrl Pts',(-12.5727648371682,3.10337692241222,4.76788914971767));
#77149=CARTESIAN_POINT('Ctrl Pts',(-12.453498864751,-2.33092176727756,5.18946230175999));
#77150=CARTESIAN_POINT('Ctrl Pts',(-12.3342328923339,-5.62547492733827,
0.847199568251026));
#77151=CARTESIAN_POINT('Ctrl Pts',(-12.2149669199167,-3.75594021589945,
-4.27277759322264));
#77152=CARTESIAN_POINT('Ctrl Pts',(-12.0957009474995,1.56148210779135,-5.47041944402838));
#77153=CARTESIAN_POINT('Ctrl Pts',(-11.9764349750824,5.44549108975312,-1.64631165274856));
#77154=CARTESIAN_POINT('Ctrl Pts',(-11.8571690026652,4.33063422408794,3.68908152305075));
#77155=CARTESIAN_POINT('Ctrl Pts',(-11.7379030302481,-0.759669330323711,
5.63796220057583));
#77156=CARTESIAN_POINT('Ctrl Pts',(-11.6186370578309,-5.1526096886059,2.41129190755513));
#77157=CARTESIAN_POINT('Ctrl Pts',(-11.4993710854137,-4.8155442174797,-3.02890230216396));
#77158=CARTESIAN_POINT('Ctrl Pts',(-11.3801051129966,-0.0578931408065744,
-5.68861702444486));
#77159=CARTESIAN_POINT('Ctrl Pts',(-11.2608391405794,4.75290282943444,-3.12628053131998));
#77160=CARTESIAN_POINT('Ctrl Pts',(-11.1415731681623,5.20061689584915,2.30592696527117));
#77161=CARTESIAN_POINT('Ctrl Pts',(-11.0223071957451,0.874255353881844,
5.62133372455018));
#77162=CARTESIAN_POINT('Ctrl Pts',(-10.9030412233279,-4.25465735538948,
3.77645416426396));
#77163=CARTESIAN_POINT('Ctrl Pts',(-10.7837752509108,-5.47786881629542,
-1.53514445509681));
#77164=CARTESIAN_POINT('Ctrl Pts',(-10.6645092784936,-1.67249224129637,
-5.43750723855698));
#77165=CARTESIAN_POINT('Ctrl Pts',(-10.5452433060764,3.66820304190325,-4.34833321054495));
#77166=CARTESIAN_POINT('Ctrl Pts',(-10.4259773336592,5.64155190838829,0.73253486709976));
#77167=CARTESIAN_POINT('Ctrl Pts',(-10.3067113612421,2.43605451516245,5.14094871261257));
#77168=CARTESIAN_POINT('Ctrl Pts',(-10.1874453888249,-3.00569843666994,
4.83006130130418));
#77169=CARTESIAN_POINT('Ctrl Pts',(-10.0681794164078,-5.68827264489775,
0.0852618546849905));
#77170=CARTESIAN_POINT('Ctrl Pts',(-9.94891344399059,-3.1491117721378,-4.73780648751502));
#77171=CARTESIAN_POINT('Ctrl Pts',(-9.82964747157344,2.28087878496807,-5.21165110448109));
#77172=CARTESIAN_POINT('Ctrl Pts',(-9.71038149915626,5.61706239742414,-0.901290901984511));
#77173=CARTESIAN_POINT('Ctrl Pts',(-9.5911155267391,3.79688069412207,4.23643862945746));
#77174=CARTESIAN_POINT('Ctrl Pts',(-9.47184955432194,-1.50877126641284,
5.48519138519372));
#77175=CARTESIAN_POINT('Ctrl Pts',(-9.35258358190478,-5.42939751829416,
1.6986341144865));
#77176=CARTESIAN_POINT('Ctrl Pts',(-9.2333176094876,-4.36593154046596,-3.6472396480792));
#77177=CARTESIAN_POINT('Ctrl Pts',(-9.11405163707046,0.705383446936543,
-5.64501102384613));
#77178=CARTESIAN_POINT('Ctrl Pts',(-8.99478566465327,5.12916873237924,-2.460760732241));
#77179=CARTESIAN_POINT('Ctrl Pts',(-8.87551969223612,4.84446657740473,2.98242499435692));
#77180=CARTESIAN_POINT('Ctrl Pts',(-8.75625371981895,0.112628594896119,
5.68779659149025));
#77181=CARTESIAN_POINT('Ctrl Pts',(-8.63698774740179,-4.72260047341405,
3.17187011636125));
#77182=CARTESIAN_POINT('Ctrl Pts',(-8.51772177498462,-5.22256467223263,
-2.25577780619104));
#77183=CARTESIAN_POINT('Ctrl Pts',(-8.39845580256746,-0.928305586732074,
-5.61266104483412));
#77184=CARTESIAN_POINT('Ctrl Pts',(-8.27918983015029,4.21812183715915,-3.81721933263432));
#77185=CARTESIAN_POINT('Ctrl Pts',(-8.15992385773312,5.49238698121822,1.48236315223396));
#77186=CARTESIAN_POINT('Ctrl Pts',(-8.04065788531597,1.72473666717901,5.42116211669091));
#77187=CARTESIAN_POINT('Ctrl Pts',(-7.9213919128988,-3.62619182684559,4.38342880647951));
#77188=CARTESIAN_POINT('Ctrl Pts',(-7.80212594048163,-5.64833946687671,
-0.678215698343313));
#77189=CARTESIAN_POINT('Ctrl Pts',(-7.68285996806448,-2.48540998688384,
-5.11727002059248));
#77190=CARTESIAN_POINT('Ctrl Pts',(-7.5635939956473,2.95908251396557,-4.85875971232364));
#77191=CARTESIAN_POINT('Ctrl Pts',(-7.44432802323015,5.68718887524218,-0.139992727946421));
#77192=CARTESIAN_POINT('Ctrl Pts',(-7.32506205081298,3.19455503717327,4.70728513912503));
#77193=CARTESIAN_POINT('Ctrl Pts',(-7.20579607839581,-2.23062460998521,
5.23335734647315));
#77194=CARTESIAN_POINT('Ctrl Pts',(-7.08653010597865,-5.60812976866394,
0.955298782780381));
#77195=CARTESIAN_POINT('Ctrl Pts',(-6.96726413356148,-3.83746960899577,
-4.19970740249727));
#77196=CARTESIAN_POINT('Ctrl Pts',(-6.84799816114433,1.45592072386326,-5.49945543780306));
#77197=CARTESIAN_POINT('Ctrl Pts',(-6.72873218872714,5.41280122438276,-1.75079929514405));
#77198=CARTESIAN_POINT('Ctrl Pts',(-6.60946621631,4.40082460355363,3.60506006542379));
#77199=CARTESIAN_POINT('Ctrl Pts',(-6.49020024389281,-0.651032250207427,
5.65153716043219));
#77200=CARTESIAN_POINT('Ctrl Pts',(-6.37093427147566,-5.10525285268721,
2.51000170850249));
#77201=CARTESIAN_POINT('Ctrl Pts',(-6.2516682990585,-4.87294037519916,-2.93567153583473));
#77202=CARTESIAN_POINT('Ctrl Pts',(-6.13240232664133,-0.167353620402568,
-5.68644951022114));
#77203=CARTESIAN_POINT('Ctrl Pts',(-6.01313635422417,4.69186083917187,-3.21716600945641));
#77204=CARTESIAN_POINT('Ctrl Pts',(-5.893870381807,5.24402887737063,2.20541977860435));
#77205=CARTESIAN_POINT('Ctrl Pts',(-5.77460440938983,0.982269865282724,
5.60346867380498));
#77206=CARTESIAN_POINT('Ctrl Pts',(-5.65533843697268,-4.18119575173463,
3.85763105444682));
#77207=CARTESIAN_POINT('Ctrl Pts',(-5.5360724645555,-5.50639659132553,-1.42944459339804));
#77208=CARTESIAN_POINT('Ctrl Pts',(-5.41680649213835,-1.776821395076,-5.40431503491021));
#77209=CARTESIAN_POINT('Ctrl Pts',(-5.29754051972118,3.58384485297817,-4.41811852900509));
#77210=CARTESIAN_POINT('Ctrl Pts',(-5.17827454730401,5.65460403049147,0.62383373177952));
#77211=CARTESIAN_POINT('Ctrl Pts',(-5.05900857488685,2.53453532784034,5.09311750684054));
#77212=CARTESIAN_POINT('Ctrl Pts',(-4.93974260246969,-2.91219260188876,
4.88700823777294));
#77213=CARTESIAN_POINT('Ctrl Pts',(-4.82047663005252,-5.68557851354222,
0.1947106389064));
#77214=CARTESIAN_POINT('Ctrl Pts',(-4.70121065763536,-3.239702509805,-4.67632793060106));
#77215=CARTESIAN_POINT('Ctrl Pts',(-4.5819446852182,2.18016389549758,-5.25457901789715));
#77216=CARTESIAN_POINT('Ctrl Pts',(-4.46267871280102,5.59867786815369,-1.00921820990431));
#77217=CARTESIAN_POINT('Ctrl Pts',(-4.34341274038386,3.87770320228423,4.16258731338466));
#77218=CARTESIAN_POINT('Ctrl Pts',(-4.2241467679667,-1.40293537371587,5.51321028110963));
#77219=CARTESIAN_POINT('Ctrl Pts',(-4.10488079554954,-5.39570374471416,
1.8028023646074));
#77220=CARTESIAN_POINT('Ctrl Pts',(-3.98561482313236,-4.43531018250885,
-3.56254668060498));
#77221=CARTESIAN_POINT('Ctrl Pts',(-3.86634885071521,0.596620772659216,
-5.65754000606162));
#77222=CARTESIAN_POINT('Ctrl Pts',(-3.74708287829804,5.08086426396513,-2.55901027698571));
#77223=CARTESIAN_POINT('Ctrl Pts',(-3.62781690588088,4.90096297439784,2.88864625562525));
#77224=CARTESIAN_POINT('Ctrl Pts',(-3.50855093346371,0.222063150189269,
5.68457590536746));
#77225=CARTESIAN_POINT('Ctrl Pts',(-3.38928496104655,-4.66068677297299,
3.26216401653732));
#77226=CARTESIAN_POINT('Ctrl Pts',(-3.27001898862938,-5.26500752383492,
-2.15485754529572));
#77227=CARTESIAN_POINT('Ctrl Pts',(-3.15075301621222,-1.03614319283671,
-5.59375746260904));
#77228=CARTESIAN_POINT('Ctrl Pts',(-3.03148704379506,4.14388251820106,-3.89768558787187));
#77229=CARTESIAN_POINT('Ctrl Pts',(-2.91222107137789,5.51989634943005,1.37639367846015));
#77230=CARTESIAN_POINT('Ctrl Pts',(-2.79295509896073,1.82874160232291,5.38696755313132));
#77231=CARTESIAN_POINT('Ctrl Pts',(-2.67368912654356,-3.54116604132071,
4.45239916610736));
#77232=CARTESIAN_POINT('Ctrl Pts',(-2.55442315412639,-5.66034501917984,
-0.569394002780302));
#77233=CARTESIAN_POINT('Ctrl Pts',(-2.43515718170923,-2.58342598938507,
-5.06849340770272));
#77234=CARTESIAN_POINT('Ctrl Pts',(-2.31589120929207,2.86503304210203,-4.91480426204542));
#77235=CARTESIAN_POINT('Ctrl Pts',(-2.1966252368749,5.68344170890555,-0.249410521087079));
#77236=CARTESIAN_POINT('Ctrl Pts',(-2.07735926445774,3.28455000970767,4.64493772835394));
#77237=CARTESIAN_POINT('Ctrl Pts',(-1.95809329204057,-2.12950131379783,
5.2753141537817));
#77238=CARTESIAN_POINT('Ctrl Pts',(-1.83882731962341,-5.58870757107013,
1.06304419081225));
#77239=CARTESIAN_POINT('Ctrl Pts',(-1.71956134720624,-3.9175777486514,-4.1250817991681));
#77240=CARTESIAN_POINT('Ctrl Pts',(-1.60029537478908,1.34982012202607,-5.52645464151563));
#77241=CARTESIAN_POINT('Ctrl Pts',(-1.48102940237192,5.37810666238975,-1.85463850777319));
#77242=CARTESIAN_POINT('Ctrl Pts',(-1.36176342995475,4.46938508421958,3.51970343005089));
#77243=CARTESIAN_POINT('Ctrl Pts',(-1.24249745753759,-0.542154052396278,
5.66301900491482));
#77244=CARTESIAN_POINT('Ctrl Pts',(-1.12323148512042,-5.05600522441769,
2.60778189985613));
#77245=CARTESIAN_POINT('Ctrl Pts',(-1.00396551270326,-4.92853178031331,
-2.84135350792509));
#77246=CARTESIAN_POINT('Ctrl Pts',(-0.884699540286091,-0.276752118554405,
-5.68217595041124));
#77247=CARTESIAN_POINT('Ctrl Pts',(-0.765433567868929,4.62908116130758,
-3.30685997111815));
#77248=CARTESIAN_POINT('Ctrl Pts',(-0.646167595451762,5.28549866915649,
2.10409578795772));
#77249=CARTESIAN_POINT('Ctrl Pts',(-0.526901623034598,1.08992058111838,
5.58352831043335));
#77250=CARTESIAN_POINT('Ctrl Pts',(-0.407635650617434,-4.10618559149057,
3.93737922415298));
#77251=CARTESIAN_POINT('Ctrl Pts',(-0.28836967820027,-5.53288500555307,
-1.32321531954648));
#77252=CARTESIAN_POINT('Ctrl Pts',(-0.169103705783104,-1.88049248148874,
-5.36912127760405));
#77253=CARTESIAN_POINT('Ctrl Pts',(-0.0498377333659409,3.4981593436186,
-4.4862675436503));
#77254=CARTESIAN_POINT('Ctrl Pts',(0.0694282390512246,5.66556190136835,
0.514901552065876));
#77255=CARTESIAN_POINT('Ctrl Pts',(0.188694211468389,2.6320774446008,5.0434000031903));
#77256=CARTESIAN_POINT('Ctrl Pts',(0.307960183885553,-2.81760820123537,
4.94214521143273));
#77257=CARTESIAN_POINT('Ctrl Pts',(0.42722615630272,-5.68077865918469,0.30408730967977));
#77258=CARTESIAN_POINT('Ctrl Pts',(0.546492128719881,-3.32909338433106,
-4.61311743888657));
#77259=CARTESIAN_POINT('Ctrl Pts',(0.665758101137048,2.07864155587013,-5.29556083420501));
#77260=CARTESIAN_POINT('Ctrl Pts',(0.785024073554211,5.57821980058984,-1.11677174161236));
#77261=CARTESIAN_POINT('Ctrl Pts',(0.904290045971376,3.9570895560061,4.08719433258361));
#77262=CARTESIAN_POINT('Ctrl Pts',(1.02355601838854,-1.29657988687734,5.53918729269027));
#77263=CARTESIAN_POINT('Ctrl Pts',(1.1428219908057,-5.36001160677062,1.906302924994));
#77264=CARTESIAN_POINT('Ctrl Pts',(1.26208796322287,-4.50304615359929,-3.47653428073288));
#77265=CARTESIAN_POINT('Ctrl Pts',(1.38135393564004,0.487637132638168,-5.66797364967663));
#77266=CARTESIAN_POINT('Ctrl Pts',(1.5006199080572,5.03067803581005,-2.65631206121851));
#77267=CARTESIAN_POINT('Ctrl Pts',(1.61988588047436,4.95564424027588,2.79379767169646));
#77268=CARTESIAN_POINT('Ctrl Pts',(1.73915185289153,0.331415461699871,5.67924986757076));
#77269=CARTESIAN_POINT('Ctrl Pts',(1.85841782530869,-4.59704693062398,3.35124973468065));
#77270=CARTESIAN_POINT('Ctrl Pts',(1.97768379772587,-5.30550041600524,-2.0531392067574));
#77271=CARTESIAN_POINT('Ctrl Pts',(2.09694977014301,-1.14359705073535,-5.57278216442251));
#77272=CARTESIAN_POINT('Ctrl Pts',(2.21621574256019,4.06810846206265,-3.97670828795007));
#77273=CARTESIAN_POINT('Ctrl Pts',(2.33548171497736,5.54536135704005,1.26991444058375));
#77274=CARTESIAN_POINT('Ctrl Pts',(2.45474768739451,1.93206924082099,5.35077786076283));
#77275=CARTESIAN_POINT('Ctrl Pts',(2.57401365981169,-3.45482874197723,4.5197205256702));
#77276=CARTESIAN_POINT('Ctrl Pts',(2.69327963222884,-5.67025419401183,-0.460361425238242));
#77277=CARTESIAN_POINT('Ctrl Pts',(2.81254560464602,-2.68048518871897,-5.0178396167688));
#77278=CARTESIAN_POINT('Ctrl Pts',(2.93181157706317,2.76992247048173,-4.9690285543632));
#77279=CARTESIAN_POINT('Ctrl Pts',(3.05107754948034,5.67758961095845,-0.358735942014323));
#77280=CARTESIAN_POINT('Ctrl Pts',(3.17034352189751,3.37332850928496,4.58087000852475));
#77281=CARTESIAN_POINT('Ctrl Pts',(3.28960949431467,-2.0275893309556,5.31531718447277));
#77282=CARTESIAN_POINT('Ctrl Pts',(3.40887546673183,-5.56721552780348,1.17039588752695));
#77283=CARTESIAN_POINT('Ctrl Pts',(3.52814143914899,-3.99623496584445,-4.04892842173314));
#77284=CARTESIAN_POINT('Ctrl Pts',(3.64740741156616,1.24321959792553,-5.55140705568331));
#77285=CARTESIAN_POINT('Ctrl Pts',(3.76667338398331,5.34142025332629,-1.95779083252319));
#77286=CARTESIAN_POINT('Ctrl Pts',(3.8859393564005,4.53629027387955,3.43304322979801));
#77287=CARTESIAN_POINT('Ctrl Pts',(4.00520532881765,-0.433075061252413,
5.67240348158324));
#77288=CARTESIAN_POINT('Ctrl Pts',(4.12447130123483,-5.00488504325426,2.70459626753531));
#77289=CARTESIAN_POINT('Ctrl Pts',(4.24373727365198,-4.98229784387044,-2.74598315026152));
#77290=CARTESIAN_POINT('Ctrl Pts',(4.36300324606915,-0.386048118200402,
-5.67579792777988));
#77291=CARTESIAN_POINT('Ctrl Pts',(4.48226921848632,4.56458704705725,-3.39532919705783));
#77292=CARTESIAN_POINT('Ctrl Pts',(4.60153519090347,5.32501091236597,2.001992519901));
#77293=CARTESIAN_POINT('Ctrl Pts',(4.72080116332065,1.1971676316396,5.56152001959095));
#77294=CARTESIAN_POINT('Ctrl Pts',(4.8400671357378,-4.02965465558056,4.01566913767982));
#77295=CARTESIAN_POINT('Ctrl Pts',(4.95933310815498,-5.55732424867229,-1.21649597684299));
#77296=CARTESIAN_POINT('Ctrl Pts',(5.07859908057214,-1.98346710468945,-5.33193900107375));
#77297=CARTESIAN_POINT('Ctrl Pts',(5.1978650529893,3.41117824849293,-4.55275501466583));
#77298=CARTESIAN_POINT('Ctrl Pts',(5.31713102540647,5.67442146263842,0.405778672313702));
#77299=CARTESIAN_POINT('Ctrl Pts',(5.43639699782363,2.72864473953703,4.99181461514278));
#77300=CARTESIAN_POINT('Ctrl Pts',(5.55566297024079,-2.7219802651905,4.99545180163613));
#77301=CARTESIAN_POINT('Ctrl Pts',(5.67492894265797,-5.67387485950943,0.413351358027617));
#77302=CARTESIAN_POINT('Ctrl Pts',(5.79419491507511,-3.41725128872073,-4.54819842314435));
#77303=CARTESIAN_POINT('Ctrl Pts',(5.91346088749229,1.97634936611633,-5.33458137529157));
#77304=CARTESIAN_POINT('Ctrl Pts',(6.03272685990945,5.55569577162621,-1.22391166335287));
#77305=CARTESIAN_POINT('Ctrl Pts',(6.15199283232661,4.03501035358811,4.01028760975979));
#77306=CARTESIAN_POINT('Ctrl Pts',(6.27125880474378,-1.18974419594258,5.56311279903411));
#77307=CARTESIAN_POINT('Ctrl Pts',(6.39052477716094,-5.32233432348004,2.00909746295764));
#77308=CARTESIAN_POINT('Ctrl Pts',(6.5097907495781,-4.56911436689826,-3.38923430419911));
#77309=CARTESIAN_POINT('Ctrl Pts',(6.62905672199528,0.378472890287174,-5.6763080904646));
#77310=CARTESIAN_POINT('Ctrl Pts',(6.74832269441244,4.97862863499266,-2.75263004804271));
#77311=CARTESIAN_POINT('Ctrl Pts',(6.86758866682961,5.00849012316842,2.69791437089479));
#77312=CARTESIAN_POINT('Ctrl Pts',(6.98685463924676,0.440645029472168,5.67182045066288));
#77313=CARTESIAN_POINT('Ctrl Pts',(7.10612061166394,-4.53170451615497,3.43909427681434));
#77314=CARTESIAN_POINT('Ctrl Pts',(7.2253865840811,-5.34402835170955,-1.95066046319719));
#77315=CARTESIAN_POINT('Ctrl Pts',(7.34465255649826,-1.25062736358769,-5.54974291873073));
#77316=CARTESIAN_POINT('Ctrl Pts',(7.46391852891543,3.99082773258522,-4.05425816585295));
#77317=CARTESIAN_POINT('Ctrl Pts',(7.58318450133259,5.5687725727736,1.16296487448275));
#77318=CARTESIAN_POINT('Ctrl Pts',(7.70245047374976,2.03468131402836,5.31260644287717));
#77319=CARTESIAN_POINT('Ctrl Pts',(7.82171644616693,-3.36721190488176,4.58536795188556));
#77320=CARTESIAN_POINT('Ctrl Pts',(7.94098241858407,-5.67806332138952,-0.351158347255461));
#77321=CARTESIAN_POINT('Ctrl Pts',(8.06024839100126,-2.77655163783317,-4.96532740803687));
#77322=CARTESIAN_POINT('Ctrl Pts',(8.17951436341841,2.67378602445897,-5.02141250665233));
#77323=CARTESIAN_POINT('Ctrl Pts',(8.29878033583558,5.66963474879634,-0.467928500731923));
#77324=CARTESIAN_POINT('Ctrl Pts',(8.41804630825273,3.46085765571055,4.51510570789498));
#77325=CARTESIAN_POINT('Ctrl Pts',(8.53731228066991,-1.924926405798,5.35335162293848));
#77326=CARTESIAN_POINT('Ctrl Pts',(8.65657825308706,-5.54366159870302,1.27731411392098));
#77327=CARTESIAN_POINT('Ctrl Pts',(8.77584422550424,-4.07341212892009,-3.97127547451985));
#77328=CARTESIAN_POINT('Ctrl Pts',(8.89511019792139,1.13615863235927,-5.57430343887665));
#77329=CARTESIAN_POINT('Ctrl Pts',(9.01437617033858,5.30275558444914,-2.0602180656789));
#77330=CARTESIAN_POINT('Ctrl Pts',(9.13364214275572,4.60151539338473,3.34511156032194));
#77331=CARTESIAN_POINT('Ctrl Pts',(9.25290811517291,-0.323835675503795,
5.6796871147826));
#77332=CARTESIAN_POINT('Ctrl Pts',(9.37217408759004,-4.95191124217634,2.8004089551642));
#77333=CARTESIAN_POINT('Ctrl Pts',(9.49144006000724,-5.03421865295653,-2.64959578441329));
#77334=CARTESIAN_POINT('Ctrl Pts',(9.61070603242439,-0.495201140240849,
-5.66731780450512));
#77335=CARTESIAN_POINT('Ctrl Pts',(9.72997200484155,4.4984023825987,-3.48254092162411));
#77336=CARTESIAN_POINT('Ctrl Pts',(9.84923797725872,5.36255097316036,1.89914778961855));
#77337=CARTESIAN_POINT('Ctrl Pts',(9.96850394967589,1.3039712965998,5.53745195231529));
#77338=CARTESIAN_POINT('Ctrl Pts',(10.087769922093,-3.95163128816538,4.09247179940786));
#77339=CARTESIAN_POINT('Ctrl Pts',(10.2070358945102,-5.579705269313,-1.10932609009118));
#77340=CARTESIAN_POINT('Ctrl Pts',(10.3263018669274,-2.08570712677686,-5.29278197622656));
#77341=CARTESIAN_POINT('Ctrl Pts',(10.4455678393445,3.32293378210522,-4.61755631761001));
#77342=CARTESIAN_POINT('Ctrl Pts',(10.5648338117617,5.68117943305569,0.296505507505705));
#77343=CARTESIAN_POINT('Ctrl Pts',(10.6840997841789,2.82420144777943,4.9383804479725));
#77344=CARTESIAN_POINT('Ctrl Pts',(10.803365756596,-2.62534421072083,5.04690826564054));
#77345=CARTESIAN_POINT('Ctrl Pts',(10.9226317290132,-5.66486967142244,0.522462316683581));
#77346=CARTESIAN_POINT('Ctrl Pts',(11.0418977014304,-3.50414357262422,-4.48159492691976));
#77347=CARTESIAN_POINT('Ctrl Pts',(11.1611636738475,1.87332521139011,-5.37162618942592));
#77348=CARTESIAN_POINT('Ctrl Pts',(11.2804296462647,5.53111412331024,-1.33059829455554));
#77349=CARTESIAN_POINT('Ctrl Pts',(11.3996956186819,4.11143673611723,3.93189562825137));
#77350=CARTESIAN_POINT('Ctrl Pts',(11.518961591099,-1.08246786880633,5.58497793903952));
#77351=CARTESIAN_POINT('Ctrl Pts',(11.6382275635162,-5.2826858490815,2.11114790729363));
#77352=CARTESIAN_POINT('Ctrl Pts',(11.7574935359334,-4.63349035324122,-3.30067908360948));
#77353=CARTESIAN_POINT('Ctrl Pts',(11.8767595083505,0.26916847590822,-5.68254024166424));
#77354=CARTESIAN_POINT('Ctrl Pts',(11.9960254807677,4.92473533864029,-2.84792856492294));
#77355=CARTESIAN_POINT('Ctrl Pts',(12.1152914531848,5.05948105096134,2.60103186476439));
#77356=CARTESIAN_POINT('Ctrl Pts',(12.234557425602,0.549711399010078,5.66229040621851));
#77357=CARTESIAN_POINT('Ctrl Pts',(12.3538233980192,-4.46468372992222,3.52566510864608));
#77358=CARTESIAN_POINT('Ctrl Pts',(12.4730893704364,-5.38057706165928,-1.84745926886156));
#77359=CARTESIAN_POINT('Ctrl Pts',(12.5923553428535,-1.35719449141834,-5.52464825839795));
#77360=CARTESIAN_POINT('Ctrl Pts',(12.7116213152707,3.91206895162486,-4.13030650004202));
#77361=CARTESIAN_POINT('Ctrl Pts',(12.8308872876878,5.59012132600284,1.05558459022699));
#77362=CARTESIAN_POINT('Ctrl Pts',(12.950153260105,2.13653981831823,5.27246743672232));
#77363=CARTESIAN_POINT('Ctrl Pts',(13.0694192325222,-3.27834797999339,4.64931713143229));
#77364=CARTESIAN_POINT('Ctrl Pts',(13.1886852049393,-5.68376950910777,-0.241825213517352));
#77365=CARTESIAN_POINT('Ctrl Pts',(13.3079511773565,-2.87158975735222,-4.91097623004087));
#77366=CARTESIAN_POINT('Ctrl Pts',(13.4272171497737,2.5766593093335,-5.07193671788022));
#77367=CARTESIAN_POINT('Ctrl Pts',(13.5464831221908,5.65958006859897,-0.576947756450346));
#77368=CARTESIAN_POINT('Ctrl Pts',(13.665749094608,3.54710503150264,4.44766918307164));
#77369=CARTESIAN_POINT('Ctrl Pts',(13.7850150670252,-1.82155056078556,5.3894033826629));
#77370=CARTESIAN_POINT('Ctrl Pts',(13.9042810394423,-5.51805450725224,1.38375927153138));
#77371=CARTESIAN_POINT('Ctrl Pts',(14.0235470118595,-4.14908065437921,-3.89215171723979));
#77372=CARTESIAN_POINT('Ctrl Pts',(14.1428129842766,1.02867687665546,-5.59513531114225));
#77373=CARTESIAN_POINT('Ctrl Pts',(14.2620789566938,5.26212697568769,-2.16188227207122));
#77374=CARTESIAN_POINT('Ctrl Pts',(14.3813449291109,4.66503628582042,3.25594098818379));
#77375=CARTESIAN_POINT('Ctrl Pts',(14.5006109015282,-0.214476353282968,
5.68486720693096));
#77376=CARTESIAN_POINT('Ctrl Pts',(14.6198768739453,-4.89710344067411,2.89518447735091));
#77377=CARTESIAN_POINT('Ctrl Pts',(14.7391428463625,-5.08427497806974,-2.55222710861131));
#77378=CARTESIAN_POINT('Ctrl Pts',(14.8584088187796,-0.60417075852906,-5.65673872130355));
#77379=CARTESIAN_POINT('Ctrl Pts',(14.9776747911968,4.43055168022577,-3.56846284489617));
#77380=CARTESIAN_POINT('Ctrl Pts',(15.0969407636139,5.3981049481225,1.79559968690459));
#77381=CARTESIAN_POINT('Ctrl Pts',(15.2162067360311,1.41029201996522,5.51133302250725));
#77382=CARTESIAN_POINT('Ctrl Pts',(15.3354727084483,-3.87214438614622,4.16775876453906));
#77383=CARTESIAN_POINT('Ctrl Pts',(15.4547386808655,-5.60001977839254,-1.00174535095946));
#77384=CARTESIAN_POINT('Ctrl Pts',(15.5740046532826,-2.18717468191774,-5.25166470534197));
#77385=CARTESIAN_POINT('Ctrl Pts',(15.6932706256998,3.23345862686471,-4.68064745253368));
#77386=CARTESIAN_POINT('Ctrl Pts',(15.8125365981169,5.68583330972381,0.187122528284859));
#77387=CARTESIAN_POINT('Ctrl Pts',(15.9318025705342,2.91871217874129,4.88311729167176));
#77388=CARTESIAN_POINT('Ctrl Pts',(16.0510685429512,-2.52773582816196,5.09649554591999));
#77389=CARTESIAN_POINT('Ctrl Pts',(16.1703345153685,-5.6537664301045,0.631379775079858));
#77390=CARTESIAN_POINT('Ctrl Pts',(16.2896004877856,-3.58973805442955,-4.41333161762595));
#77391=CARTESIAN_POINT('Ctrl Pts',(16.4088664602028,1.76960724793751,-5.4066815566115));
#77392=CARTESIAN_POINT('Ctrl Pts',(16.5281324326199,5.50448395975385,-1.43679212253169));
#77393=CARTESIAN_POINT('Ctrl Pts',(16.6473984050371,4.18634039815506,3.85204742148009));
#77394=CARTESIAN_POINT('Ctrl Pts',(16.7666643774543,-0.974790636558288,
5.6047746146865));
#77395=CARTESIAN_POINT('Ctrl Pts',(16.8859303498714,-5.24108086786879,2.21241646238138));
#77396=CARTESIAN_POINT('Ctrl Pts',(17.0051963222886,-4.69615027020021,-3.21090141646471));
#77397=CARTESIAN_POINT('Ctrl Pts',(17.1244622947058,0.159764371717757,-5.68666779512269));
#77398=CARTESIAN_POINT('Ctrl Pts',(17.2437282671229,4.86901810678927,-2.94217231689695));
#77399=CARTESIAN_POINT('Ctrl Pts',(17.3629942395401,5.1085981385457,2.50318603491707));
#77400=CARTESIAN_POINT('Ctrl Pts',(17.4822602119573,0.658574176260086,5.65066326380534));
#77401=CARTESIAN_POINT('Ctrl Pts',(17.6015261843744,-4.39600939388725,3.61093016761771));
#77402=CARTESIAN_POINT('Ctrl Pts',(17.7207921567916,-5.41513300959612,-1.74357384556518));
#77403=CARTESIAN_POINT('Ctrl Pts',(17.8400581292087,-1.46325896579829,-5.49750747753623));
#77404=CARTESIAN_POINT('Ctrl Pts',(17.9593241016259,3.83186128845189,-4.20482512509383));
#77405=CARTESIAN_POINT('Ctrl Pts',(18.0785900740431,5.6093997099579,0.947813357407833));
#77406=CARTESIAN_POINT('Ctrl Pts',(18.1978560464602,2.23760702915769,5.23037570826609));
#77407=CARTESIAN_POINT('Ctrl Pts',(18.3171220188774,-3.18826987914481,4.71154437995594));
#77408=CARTESIAN_POINT('Ctrl Pts',(18.4363879912946,-5.68737064381084,-0.132402516876524));
#77409=CARTESIAN_POINT('Ctrl Pts',(18.5556539637117,-2.96556434875542,-4.85480621239888));
#77410=CARTESIAN_POINT('Ctrl Pts',(18.6749199361289,2.47857829716258,-5.12058247579229));
#77411=CARTESIAN_POINT('Ctrl Pts',(18.7941859085461,5.64742929423926,-0.685753332565547));
#77412=CARTESIAN_POINT('Ctrl Pts',(18.9134518809632,3.63203869389911,4.3785854099898));
#77413=CARTESIAN_POINT('Ctrl Pts',(19.0327178533804,-1.7175000824166,5.42345911143944));
#77414=CARTESIAN_POINT('Ctrl Pts',(19.1519838257975,-5.49040373734829,1.48969193710258));
#77415=CARTESIAN_POINT('Ctrl Pts',(19.2712497982147,-4.22321251746525,-3.8115864543364));
#77416=CARTESIAN_POINT('Ctrl Pts',(19.3905157706319,0.920814137986261,-5.61389495714349));
#77417=CARTESIAN_POINT('Ctrl Pts',(19.5097817430491,5.21954947434026,-2.26274579912789));
#77418=CARTESIAN_POINT('Ctrl Pts',(19.6290477154662,4.72682942545333,3.16556453878679));
#77419=CARTESIAN_POINT('Ctrl Pts',(19.7483136878834,-0.105037597141629,
5.68794183951833));
#77420=CARTESIAN_POINT('Ctrl Pts',(19.8675796603006,-4.84048193748196,2.98888773283097));
#77421=CARTESIAN_POINT('Ctrl Pts',(19.9868456327177,-5.13244828024263,-2.45391318452596));
#77422=CARTESIAN_POINT('Ctrl Pts',(20.1061116051349,-0.712916614844916,
-5.644064596267));
#77423=CARTESIAN_POINT('Ctrl Pts',(20.225377577552,4.36106006926938,-3.65306314464733));
#77424=CARTESIAN_POINT('Ctrl Pts',(20.3446435499692,5.43165966940629,1.69138656205524));
#77425=CARTESIAN_POINT('Ctrl Pts',(20.4639095223863,1.51609042456612,5.48317290362938));
#77426=CARTESIAN_POINT('Ctrl Pts',(20.5831754948035,-3.79122338846171,4.24150214963253));
#77427=CARTESIAN_POINT('Ctrl Pts',(20.7024414672207,-5.6182602521859,-0.893793603279791));
#77428=CARTESIAN_POINT('Ctrl Pts',(20.8217074396379,-2.28783219037207,-5.20860241670007));
#77429=CARTESIAN_POINT('Ctrl Pts',(20.940973412055,3.14278592098079,-4.74200505286967));
#77430=CARTESIAN_POINT('Ctrl Pts',(21.0602393844722,5.68838136902297,0.0776702459646251));
#77431=CARTESIAN_POINT('Ctrl Pts',(21.1795053568894,3.01214192922678,4.826045613621));
#77432=CARTESIAN_POINT('Ctrl Pts',(21.2987713293065,-2.42919126796274,5.14419527722365));
#77433=CARTESIAN_POINT('Ctrl Pts',(21.4180373017237,-5.64056924777562,0.740063394314221));
#77434=CARTESIAN_POINT('Ctrl Pts',(21.5373032741408,-3.67400303318194,-4.34343377740774));
#77435=CARTESIAN_POINT('Ctrl Pts',(21.656569246558,1.66523388896478,-5.43973449366784));
#77436=CARTESIAN_POINT('Ctrl Pts',(21.7758352189752,5.47581514376105,-1.54245381710865));
#77437=CARTESIAN_POINT('Ctrl Pts',(21.8951011913923,4.25969359822163,3.77077256219813));
#77438=CARTESIAN_POINT('Ctrl Pts',(22.0143671638095,-0.866752378767923,
5.62249549403613));
#77439=CARTESIAN_POINT('Ctrl Pts',(22.1336331362266,-5.1975347887514,2.31286562218276));
#77440=CARTESIAN_POINT('Ctrl Pts',(22.2528991086438,-4.7570709109148,-3.11993455301305));
#77441=CARTESIAN_POINT('Ctrl Pts',(22.372165081061,0.0503010968532085,-5.68868922215055));
#77442=CARTESIAN_POINT('Ctrl Pts',(22.4914310534782,4.81149757499245,-3.03532639964759));
#77443=CARTESIAN_POINT('Ctrl Pts',(22.6106970258953,5.15582319481218,2.40441311974323));
#77444=CARTESIAN_POINT('Ctrl Pts',(22.7299629983125,0.767193042571622,5.63694332967666));
#77445=CARTESIAN_POINT('Ctrl Pts',(22.8492289707296,-4.32570694242367,3.69485787477996));
#77446=CARTESIAN_POINT('Ctrl Pts',(22.9684949431469,-5.44768339730547,-1.63904266853516));
#77447=CARTESIAN_POINT('Ctrl Pts',(23.0877609155639,-1.56878150446242,-5.46833062806312));
#77448=CARTESIAN_POINT('Ctrl Pts',(23.2070268879812,3.75023444894761,-4.27778644213131));
#77449=CARTESIAN_POINT('Ctrl Pts',(23.3262928603983,5.62660058465537,0.839691090409063));
#77450=CARTESIAN_POINT('Ctrl Pts',(23.4455588328155,2.3378455150786,5.18634684669117));
#77451=CARTESIAN_POINT('Ctrl Pts',(23.5648248052326,-3.09701096385403,4.77202665083964));
#77452=CARTESIAN_POINT('Ctrl Pts',(23.6840907776498,-5.68886539177463,-0.0229307833566997));
#77453=CARTESIAN_POINT('Ctrl Pts',(23.8033567500669,-3.05844060741237,-4.79683815835885));
#77454=CARTESIAN_POINT('Ctrl Pts',(23.9226227224842,2.37957931343959,-5.16733176384159));
#77455=CARTESIAN_POINT('Ctrl Pts',(24.0418886949013,5.63318692590381,-0.794304931611839));
#77456=CARTESIAN_POINT('Ctrl Pts',(24.1611546673185,3.71562718668736,4.30787997466344));
#77457=CARTESIAN_POINT('Ctrl Pts',(24.2804206397356,-1.61281350704876,5.45550619631551));
#77458=CARTESIAN_POINT('Ctrl Pts',(24.3996866121528,-5.46071952978924,1.59507287718616));
#77459=CARTESIAN_POINT('Ctrl Pts',(24.51895258457,-4.2957802625431,-3.72960952413273));
#77460=CARTESIAN_POINT('Ctrl Pts',(24.6382185569871,0.812610364626208,-5.63057542901771));
#77461=CARTESIAN_POINT('Ctrl Pts',(24.7574845294043,5.17503884950108,-2.36277129081743));
#77462=CARTESIAN_POINT('Ctrl Pts',(24.8767505018215,4.78687192644435,3.07401568414598));
#77463=CARTESIAN_POINT('Ctrl Pts',(24.9960164742386,0.00444006094848726,
5.68890987381718));
#77464=CARTESIAN_POINT('Ctrl Pts',(25.1152824466558,-4.78206770306065,3.08148401746638));
#77465=CARTESIAN_POINT('Ctrl Pts',(25.2345484190729,-5.17872071790823,-2.35469042391236));
#77466=CARTESIAN_POINT('Ctrl Pts',(25.3538143914901,-0.821398433840538,
-5.62930012341145));
#77467=CARTESIAN_POINT('Ctrl Pts',(25.4730803639073,4.28995328679094,-3.73631048812972));
#77468=CARTESIAN_POINT('Ctrl Pts',(25.5923463363244,5.46320270961362,1.58654701166618));
#77469=CARTESIAN_POINT('Ctrl Pts',(25.7116123087416,1.62132732667911,5.45298202512345));
#77470=CARTESIAN_POINT('Ctrl Pts',(25.8308782811588,-3.70889826518536,4.31367464293049));
#77471=CARTESIAN_POINT('Ctrl Pts',(25.950144253576,-5.63441993511243,-0.785510828292191));
#77472=CARTESIAN_POINT('Ctrl Pts',(26.0694102259931,-2.38764237240975,-5.16361105894212));
#77473=CARTESIAN_POINT('Ctrl Pts',(26.1886761984103,3.05094924619048,-4.80160639408587));
#77474=CARTESIAN_POINT('Ctrl Pts',(26.3079421708274,5.68882266724869,-0.031810802473794));
#77475=CARTESIAN_POINT('Ctrl Pts',(26.4272081432446,3.1044560963937,4.76718655100886));
#77476=CARTESIAN_POINT('Ctrl Pts',(26.5464741156617,-2.32974702729697,5.18998979337701));
#77477=CARTESIAN_POINT('Ctrl Pts',(26.6657400880789,-5.62528301217263,0.848472922089174));
#77478=CARTESIAN_POINT('Ctrl Pts',(26.7850060604961,-3.75690730032363,-4.27192729377863));
#77479=CARTESIAN_POINT('Ctrl Pts',(26.9042720329132,1.56024379041213,-5.47077275903843));
#77480=CARTESIAN_POINT('Ctrl Pts',(27.0235380053304,5.44511829317601,-1.6475442451954));
#77481=CARTESIAN_POINT('Ctrl Pts',(27.1428039777475,4.33146916906887,3.68810115153607));
#77482=CARTESIAN_POINT('Ctrl Pts',(27.2620699501648,-0.75839310871523,5.63813401394555));
#77483=CARTESIAN_POINT('Ctrl Pts',(27.3813359225819,-5.1520637395484,2.41245818413233));
#77484=CARTESIAN_POINT('Ctrl Pts',(27.5006018949991,-4.81622971268621,-3.02781218393652));
#77485=CARTESIAN_POINT('Ctrl Pts',(27.6198678674162,-0.0591808076330519,
-5.68860377408766));
#77486=CARTESIAN_POINT('Ctrl Pts',(27.7391338398334,4.75219504667706,-3.12735631242981));
#77487=CARTESIAN_POINT('Ctrl Pts',(27.8583998122506,5.20113872938789,2.30474970099082));
#77488=CARTESIAN_POINT('Ctrl Pts',(27.9776657846677,0.875527769629323,5.62113568517647));
#77489=CARTESIAN_POINT('Ctrl Pts',(28.0969317570849,-4.25380241289778,3.77741714648801));
#77490=CARTESIAN_POINT('Ctrl Pts',(28.2161977295021,-5.4782161693561,-1.53390445216165));
#77491=CARTESIAN_POINT('Ctrl Pts',(28.3354637019192,-1.67372302585793,-5.4371285159787));
#77492=CARTESIAN_POINT('Ctrl Pts',(28.4547296743364,3.66721866460272,-4.34916342904541));
#77493=CARTESIAN_POINT('Ctrl Pts',(28.5739956467536,5.64171757954254,0.731257833624528));
#77494=CARTESIAN_POINT('Ctrl Pts',(28.6932616191707,2.43721815154126,5.14039715862049));
#77495=CARTESIAN_POINT('Ctrl Pts',(28.8125275915879,-3.00460503296775,4.83074154374061));
#77496=CARTESIAN_POINT('Ctrl Pts',(28.9317935640051,-5.68825319940117,0.0865494428570666));
#77497=CARTESIAN_POINT('Ctrl Pts',(29.0510595364222,-3.15018413547354,-4.73709353709283));
#77498=CARTESIAN_POINT('Ctrl Pts',(29.1703255088394,2.27969902363949,-5.21216726786216));
#77499=CARTESIAN_POINT('Ctrl Pts',(29.2895914812565,5.61685823842664,-0.902562350187162));
#77500=CARTESIAN_POINT('Ctrl Pts',(29.4088574536737,3.79783955185462,4.23557906370835));
#77501=CARTESIAN_POINT('Ctrl Pts',(29.5281234260908,-1.50752960662557,5.48553276826453));
#77502=CARTESIAN_POINT('Ctrl Pts',(29.6473893985081,-5.42901287848164,1.69986306267211));
#77503=CARTESIAN_POINT('Ctrl Pts',(29.7666553709251,-4.36675701326764,-3.64625128777951));
#77504=CARTESIAN_POINT('Ctrl Pts',(29.8859213433424,0.704105631155751,-5.6451705489499));
#77505=CARTESIAN_POINT('Ctrl Pts',(30.0051873157595,5.12861158622029,-2.46192170148515));
#77506=CARTESIAN_POINT('Ctrl Pts',(30.1244532881767,4.84514155132446,2.98132833049047));
#77507=CARTESIAN_POINT('Ctrl Pts',(30.2437192605939,0.113916074608287,5.68777095130442));
#77508=CARTESIAN_POINT('Ctrl Pts',(30.362985233011,-4.72188237183086,3.17293903709944));
#77509=CARTESIAN_POINT('Ctrl Pts',(30.4822512054282,-5.22307515350755,-2.25459557512384));
#77510=CARTESIAN_POINT('Ctrl Pts',(30.6015171778453,-0.929576037957939,
-5.61245077093875));
#77511=CARTESIAN_POINT('Ctrl Pts',(30.7207831502625,4.21725766805032,-3.81817404367943));
#77512=CARTESIAN_POINT('Ctrl Pts',(30.8400491226797,5.49272238639658,1.48111986433704));
#77513=CARTESIAN_POINT('Ctrl Pts',(30.9593150950968,1.7259637505406,5.42077156854781));
#77514=CARTESIAN_POINT('Ctrl Pts',(31.078581067514,-3.62519950642571,4.38424951447422));
#77515=CARTESIAN_POINT('Ctrl Pts',(31.1978470399311,-5.64849284223719,-0.676937129836315));
#77516=CARTESIAN_POINT('Ctrl Pts',(31.3171130123484,-2.48656826211884,-5.11670729516354));
#77517=CARTESIAN_POINT('Ctrl Pts',(31.4363789847655,2.95798261532084,-4.85942940210229));
#77518=CARTESIAN_POINT('Ctrl Pts',(31.5556449571827,5.68715704096057,-0.141280069395615));
#77519=CARTESIAN_POINT('Ctrl Pts',(31.6749109295998,3.19562049057018,4.70656190300357));
#77520=CARTESIAN_POINT('Ctrl Pts',(31.7941769020171,-2.22943993654606,5.23386213382527));
#77521=CARTESIAN_POINT('Ctrl Pts',(31.9134428744341,-5.60791338473815,0.956568207620598));
#77522=CARTESIAN_POINT('Ctrl Pts',(32.0327088468514,-3.83842015125344,-4.19883865003266));
#77523=CARTESIAN_POINT('Ctrl Pts',(32.1519748192685,1.45467583663671,-5.49978485732504));
#77524=CARTESIAN_POINT('Ctrl Pts',(32.2712407916857,5.41240477694961,-1.75202448527666));
#77525=CARTESIAN_POINT('Ctrl Pts',(32.3905067641028,4.40164052774331,3.60406380785415));
#77526=CARTESIAN_POINT('Ctrl Pts',(32.50977273652,-0.649752958570897,5.65168438249916));
#77527=CARTESIAN_POINT('Ctrl Pts',(32.6290387089371,-5.10468456101445,2.51115726291617));
#77528=CARTESIAN_POINT('Ctrl Pts',(32.7483046813543,-4.87360476533446,-2.93456842787243));
#77529=CARTESIAN_POINT('Ctrl Pts',(32.8675706537715,-0.168640793789048,
-5.6864114825808));
#77530=CARTESIAN_POINT('Ctrl Pts',(32.9868366261887,4.69113248525386,-3.21822797084853));
#77531=CARTESIAN_POINT('Ctrl Pts',(33.1061025986057,5.24452795911491,2.20423269021639));
#77532=CARTESIAN_POINT('Ctrl Pts',(33.2253685710231,0.983538234352283,5.60324618485782));
#77533=CARTESIAN_POINT('Ctrl Pts',(33.3446345434401,-4.18032243602443,3.85857740591355));
#77534=CARTESIAN_POINT('Ctrl Pts',(33.4639005158574,-5.50672001756556,-1.42819813565887));
#77535=CARTESIAN_POINT('Ctrl Pts',(33.5831664882745,-1.77804466361857,-5.4039126973642));
#77536=CARTESIAN_POINT('Ctrl Pts',(33.7024324606916,3.58284468132043,-4.41892965050241));
#77537=CARTESIAN_POINT('Ctrl Pts',(33.8216984331088,5.65474509585696,0.622553746626874));
#77538=CARTESIAN_POINT('Ctrl Pts',(33.940964405526,2.53568813468345,5.09254366207905));
#77539=CARTESIAN_POINT('Ctrl Pts',(34.0602303779431,-2.91108631014372,4.88766731288531));
#77540=CARTESIAN_POINT('Ctrl Pts',(34.1794963503603,-5.68553429342391,0.195997614434357));
#77541=CARTESIAN_POINT('Ctrl Pts',(34.2987623227774,-3.24076095460869,-4.67559447574684));
#77542=CARTESIAN_POINT('Ctrl Pts',(34.4180282951946,2.17897441963776,-5.25507238248037));
#77543=CARTESIAN_POINT('Ctrl Pts',(34.5372942676118,5.59844927933938,-1.01048549384319));
#77544=CARTESIAN_POINT('Ctrl Pts',(34.656560240029,3.87864534104596,4.1617094546457));
#77545=CARTESIAN_POINT('Ctrl Pts',(34.7758262124461,-1.40168737430279,5.51352770657897));
#77546=CARTESIAN_POINT('Ctrl Pts',(34.8950921848633,-5.39529552639648,1.80402368324702));
#77547=CARTESIAN_POINT('Ctrl Pts',(35.0143581572804,-4.43611648248496,-3.56154261801842));
#77548=CARTESIAN_POINT('Ctrl Pts',(35.1336241296976,0.595340123519527,-5.657674911447));
#77549=CARTESIAN_POINT('Ctrl Pts',(35.2528901021148,5.08028487958908,-2.5601603095978));
#77550=CARTESIAN_POINT('Ctrl Pts',(35.3721560745319,4.90161671886864,2.88753680575381));
#77551=CARTESIAN_POINT('Ctrl Pts',(35.4914220469491,0.223349898755441,5.68452549370444));
#77552=CARTESIAN_POINT('Ctrl Pts',(35.6106880193663,-4.65994823546759,3.26321892042295));
#77553=CARTESIAN_POINT('Ctrl Pts',(35.7299539917834,-5.26549515735449,-2.15366570982432));
#77554=CARTESIAN_POINT('Ctrl Pts',(35.8492199642006,-1.03740936702376,-5.59352277860006));
#77555=CARTESIAN_POINT('Ctrl Pts',(35.9684859366177,4.14300014570849,-3.89862349329523));
#77556=CARTESIAN_POINT('Ctrl Pts',(36.087751909035,5.5202077497737,1.3751441684951));
#77557=CARTESIAN_POINT('Ctrl Pts',(36.2070178814521,1.82996097509064,5.38655345925063));
#77558=CARTESIAN_POINT('Ctrl Pts',(36.3262838538692,-3.54015817240135,4.45320063395262));
#77559=CARTESIAN_POINT('Ctrl Pts',(36.4455498262865,-5.66047364493052,-0.568112734597499));
#77560=CARTESIAN_POINT('Ctrl Pts',(36.5648157987035,-2.58457344247884,-5.06790846806574));
#77561=CARTESIAN_POINT('Ctrl Pts',(36.6840817711207,2.86392088017567,-4.91545271593295));
#77562=CARTESIAN_POINT('Ctrl Pts',(36.8033477435379,5.68338430840045,-0.250696908077834));
#77563=CARTESIAN_POINT('Ctrl Pts',(36.9226137159551,3.28560286481452,4.64419392618976));
#77564=CARTESIAN_POINT('Ctrl Pts',(37.0418796883722,-2.12831002677038,5.27579642311569));
#77565=CARTESIAN_POINT('Ctrl Pts',(37.1611456607894,-5.58846132630211,1.06430850767035));
#77566=CARTESIAN_POINT('Ctrl Pts',(37.2804116332066,-3.9185217903309,-4.12419356911063));
#77567=CARTESIAN_POINT('Ctrl Pts',(37.3996776056237,1.34858886709791,-5.5267626006799));
#77568=CARTESIAN_POINT('Ctrl Pts',(37.5189435780409,5.37764921580746,-1.85585098494954));
#77569=CARTESIAN_POINT('Ctrl Pts',(37.6382095504581,4.47025290163574,3.51868243053033));
#77570=CARTESIAN_POINT('Ctrl Pts',(37.7574755228752,-0.541007429195424,
5.66315910227798));
#77571=CARTESIAN_POINT('Ctrl Pts',(37.8767414952924,-5.0551578814661,2.60889302618054));
#77572=CARTESIAN_POINT('Ctrl Pts',(37.9960074677095,-4.92966283975873,-2.84017461837445));
#77573=CARTESIAN_POINT('Ctrl Pts',(38.1152734401267,-0.277111040578141,
-5.68223314890805));
#77574=CARTESIAN_POINT('Ctrl Pts',(38.2345394125439,4.62656819708096,-3.30768024346582));
#77575=CARTESIAN_POINT('Ctrl Pts',(38.3538053849611,5.28935206274146,2.1024708769518));
#77576=CARTESIAN_POINT('Ctrl Pts',(38.4730713573782,1.08454695527874,5.58406416185194));
#77577=CARTESIAN_POINT('Ctrl Pts',(38.5724596677259,-3.22824135538267,4.21160970579805));
#77578=CARTESIAN_POINT('Ctrl Pts',(38.6519703160039,-4.83334745226005,1.30553258485445));
#77579=CARTESIAN_POINT('Ctrl Pts',(38.691725640143,-4.86505302969868,-0.338699302841263));
#77580=CARTESIAN_POINT('Ctrl Pts',(38.7116033022125,-4.67889930883017,-1.11786102211901));
#77581=CARTESIAN_POINT('Ctrl Pts',(-17.6184,-2.11639460593172,4.47917290043409));
#77582=CARTESIAN_POINT('Ctrl Pts',(-17.5985223379305,-2.8622965430514,4.1267366646904));
#77583=CARTESIAN_POINT('Ctrl Pts',(-17.5587670137914,-4.16282509234333,
3.04193699287371));
#77584=CARTESIAN_POINT('Ctrl Pts',(-17.4792563655133,-5.46341108425688,
-0.119881008423284));
#77585=CARTESIAN_POINT('Ctrl Pts',(-17.3798680551657,-3.78742768517455,
-4.46895156442932));
#77586=CARTESIAN_POINT('Ctrl Pts',(-17.2606020827485,1.71866712847336,-5.60395676842087));
#77587=CARTESIAN_POINT('Ctrl Pts',(-17.1413361103314,5.63810416435217,-1.58589123022531));
#77588=CARTESIAN_POINT('Ctrl Pts',(-17.0220701379142,4.38650144303843,3.88351482617148));
#77589=CARTESIAN_POINT('Ctrl Pts',(-16.902804165497,-0.894268453325975,
5.79026664325592));
#77590=CARTESIAN_POINT('Ctrl Pts',(-16.7835381930799,-5.35283428647187,
2.38042187278717));
#77591=CARTESIAN_POINT('Ctrl Pts',(-16.6642722206627,-4.89826604426309,
-3.21395979162865));
#77592=CARTESIAN_POINT('Ctrl Pts',(-16.5450062482455,0.0531800766195173,
-5.8583240260201));
#77593=CARTESIAN_POINT('Ctrl Pts',(-16.4257402758284,4.95562086810942,-3.12466912572249));
#77594=CARTESIAN_POINT('Ctrl Pts',(-16.3064743034112,5.30898655851339,2.47728284467523));
#77595=CARTESIAN_POINT('Ctrl Pts',(-16.187208330994,0.78874335884052,5.80518222363476));
#77596=CARTESIAN_POINT('Ctrl Pts',(-16.0679423585769,-4.45552520423068,
3.80399931897383));
#77597=CARTESIAN_POINT('Ctrl Pts',(-15.9486763861597,-5.60971370183634,
-1.68917479670012));
#77598=CARTESIAN_POINT('Ctrl Pts',(-15.8294104137426,-1.61427529499575,
-5.63172318529513));
#77599=CARTESIAN_POINT('Ctrl Pts',(-15.7101444413254,3.8630356967424,-4.40444407974865));
#77600=CARTESIAN_POINT('Ctrl Pts',(-15.5908784689082,5.79414938910801,0.866035857838147));
#77601=CARTESIAN_POINT('Ctrl Pts',(-15.471612496491,2.40633389206521,5.34151104403555));
#77602=CARTESIAN_POINT('Ctrl Pts',(-15.3523465240739,-3.19045356878321,
4.9135716920102));
#77603=CARTESIAN_POINT('Ctrl Pts',(-15.2330805516567,-5.85846060296283,
-0.0249404831624147));
#77604=CARTESIAN_POINT('Ctrl Pts',(-15.1138145792395,-3.14850281774238,
-4.94055788474845));
#77605=CARTESIAN_POINT('Ctrl Pts',(-14.9945486068224,2.45172555749452,-5.32082923295528));
#77606=CARTESIAN_POINT('Ctrl Pts',(-14.8752826344052,5.80131267523169,-0.816672186855044));
#77607=CARTESIAN_POINT('Ctrl Pts',(-14.7560166619881,3.82539591211262,4.43717570612341));
#77608=CARTESIAN_POINT('Ctrl Pts',(-14.6367506895709,-1.66216756865306,
5.61777367608827));
#77609=CARTESIAN_POINT('Ctrl Pts',(-14.5174847171538,-5.62389021715314,
1.64135339515628));
#77610=CARTESIAN_POINT('Ctrl Pts',(-14.3982187447366,-4.42297972703404,
-3.84180067960166));
#77611=CARTESIAN_POINT('Ctrl Pts',(-14.2789527723194,0.838149011166279,
-5.79824873215111));
#77612=CARTESIAN_POINT('Ctrl Pts',(-14.1596867999022,5.32987157590943,-2.43200557458098));
#77613=CARTESIAN_POINT('Ctrl Pts',(-14.0404208274851,4.92886498975685,3.16677628523976));
#77614=CARTESIAN_POINT('Ctrl Pts',(-13.9211548550679,0.00324630575561585,
5.85851274551346));
#77615=CARTESIAN_POINT('Ctrl Pts',(-13.8018888826508,-4.92535243045046,
3.17223668166147));
#77616=CARTESIAN_POINT('Ctrl Pts',(-13.6826229102336,-5.33256353665323,
-2.42609733023661));
#77617=CARTESIAN_POINT('Ctrl Pts',(-13.5633569378164,-0.844574319486159,
-5.7973163055935));
#77618=CARTESIAN_POINT('Ctrl Pts',(-13.4440909653992,4.41871939308572,-3.84670002125304));
#77619=CARTESIAN_POINT('Ctrl Pts',(-13.3248249929821,5.62570576802085,1.63511979375657));
#77620=CARTESIAN_POINT('Ctrl Pts',(-13.2055590205649,1.66839236374145,5.61592815560291));
#77621=CARTESIAN_POINT('Ctrl Pts',(-13.0862930481478,-3.82047613265049,
4.44141241590395));
#77622=CARTESIAN_POINT('Ctrl Pts',(-12.9670270757306,-5.80221417075813,
-0.810242460589229));
#77623=CARTESIAN_POINT('Ctrl Pts',(-12.8477611033134,-2.45762079435045,
-5.31810888939538));
#77624=CARTESIAN_POINT('Ctrl Pts',(-12.7284951308963,3.14302560882944,-4.94404410887827));
#77625=CARTESIAN_POINT('Ctrl Pts',(-12.6092291584791,5.85842931943376,-0.0314330636285068));
#77626=CARTESIAN_POINT('Ctrl Pts',(-12.4899631860619,3.19589708946511,4.91003298581984));
#77627=CARTESIAN_POINT('Ctrl Pts',(-12.3706972136448,-2.40041293019083,
5.34417438832823));
#77628=CARTESIAN_POINT('Ctrl Pts',(-12.2514312412276,-5.79318574463262,
0.872456908091129));
#77629=CARTESIAN_POINT('Ctrl Pts',(-12.1321652688104,-3.86791508228008,
-4.4001607975801));
#77630=CARTESIAN_POINT('Ctrl Pts',(-12.0128992963933,1.60803416675023,-5.63350763262592));
#77631=CARTESIAN_POINT('Ctrl Pts',(-11.8936333239761,5.60783609582425,-1.69539271281352));
#77632=CARTESIAN_POINT('Ctrl Pts',(-11.7743673515589,4.45974229309636,3.79906314865365));
#77633=CARTESIAN_POINT('Ctrl Pts',(-11.6551013791418,-0.78231715400237,
5.80604529769138));
#77634=CARTESIAN_POINT('Ctrl Pts',(-11.5358354067246,-5.3062230978268,2.48317912450548));
#77635=CARTESIAN_POINT('Ctrl Pts',(-11.4165694343075,-4.95910878169189,
-3.11920217678126));
#77636=CARTESIAN_POINT('Ctrl Pts',(-11.2973034618903,-0.0596190939189362,
-5.85821028061735));
#77637=CARTESIAN_POINT('Ctrl Pts',(-11.1780374894731,4.89459988227734,-3.21948351769366));
#77638=CARTESIAN_POINT('Ctrl Pts',(-11.0587715170559,5.35566153142266,2.37467296466905));
#77639=CARTESIAN_POINT('Ctrl Pts',(-10.9395055446388,0.900319300804774,
5.78892108124553));
#77640=CARTESIAN_POINT('Ctrl Pts',(-10.8202395722216,-4.38150034582086,
3.88904060763863));
#77641=CARTESIAN_POINT('Ctrl Pts',(-10.7009735998045,-5.64117909108611,
-1.58091131648284));
#77642=CARTESIAN_POINT('Ctrl Pts',(-10.5817076273873,-1.72235381642172,
-5.59961422415402));
#77643=CARTESIAN_POINT('Ctrl Pts',(-10.4624416549701,3.77756222279128,-4.47796893482199));
#77644=CARTESIAN_POINT('Ctrl Pts',(-10.343175682553,5.80974202452692,0.754373738101006));
#77645=CARTESIAN_POINT('Ctrl Pts',(-10.2239097101358,2.50867997327711,5.29421447619652));
#77646=CARTESIAN_POINT('Ctrl Pts',(-10.1046437377186,-3.09530654049515,
4.97405865955143));
#77647=CARTESIAN_POINT('Ctrl Pts',(-9.98537776530148,-5.8578556341726,0.0878037441284453));
#77648=CARTESIAN_POINT('Ctrl Pts',(-9.86611179288431,-3.24299542034126,
-4.87905347705231));
#77649=CARTESIAN_POINT('Ctrl Pts',(-9.74684582046715,2.34887802949731,-5.36702470003963));
#77650=CARTESIAN_POINT('Ctrl Pts',(-9.62757984805,5.78452241415752,-0.928160852654129));
#77651=CARTESIAN_POINT('Ctrl Pts',(-9.50831387563281,3.91007610830566,4.36273846976275));
#77652=CARTESIAN_POINT('Ctrl Pts',(-9.38904790321567,-1.55375187080085,
5.64871996582177));
#77653=CARTESIAN_POINT('Ctrl Pts',(-9.26978193079848,-5.59126273091542,
1.74927505046137));
#77654=CARTESIAN_POINT('Ctrl Pts',(-9.15051595838133,-4.49609191916458,
-3.75597385277289));
#77655=CARTESIAN_POINT('Ctrl Pts',(-9.03124998596417,0.726412859727577,
-5.81330426569202));
#77656=CARTESIAN_POINT('Ctrl Pts',(-8.911984013547,5.28208330248386,-2.53412275036385));
#77657=CARTESIAN_POINT('Ctrl Pts',(-8.79271804112984,4.98889339639251,3.07133925311447));
#77658=CARTESIAN_POINT('Ctrl Pts',(-8.67345206871268,0.115986361830236,
5.85736538830899));
#77659=CARTESIAN_POINT('Ctrl Pts',(-8.5541860962955,-4.86339413001757,3.26643225314731));
#77660=CARTESIAN_POINT('Ctrl Pts',(-8.43492012387835,-5.37826363114107,
-2.32302872178451));
#77661=CARTESIAN_POINT('Ctrl Pts',(-8.31565415146118,-0.955980919154609,
-5.7799898451903));
#77662=CARTESIAN_POINT('Ctrl Pts',(-8.19638817904402,4.34387560371134,-3.93102109734504));
#77663=CARTESIAN_POINT('Ctrl Pts',(-8.07712220662684,5.65613008227446,1.52655645839927));
#77664=CARTESIAN_POINT('Ctrl Pts',(-7.95785623420969,1.77615579175165,5.58278180943137));
#77665=CARTESIAN_POINT('Ctrl Pts',(-7.83859026179252,-3.73429853833258,
4.51411082660778));
#77666=CARTESIAN_POINT('Ctrl Pts',(-7.71932428937535,-5.81673193872685,
-0.698435166128912));
#77667=CARTESIAN_POINT('Ctrl Pts',(-7.6000583169582,-2.55950686680862,-5.26982985750491));
#77668=CARTESIAN_POINT('Ctrl Pts',(-7.48079234454101,3.04730086944123,-5.00361264881616));
#77669=CARTESIAN_POINT('Ctrl Pts',(-7.36152637212387,5.85673955437486,-0.144166294644587));
#77670=CARTESIAN_POINT('Ctrl Pts',(-7.24226039970669,3.28979347358892,4.84762220366051));
#77671=CARTESIAN_POINT('Ctrl Pts',(-7.12299442728954,-2.29712563989832,
5.3893780645648));
#77672=CARTESIAN_POINT('Ctrl Pts',(-7.00372845487236,-5.77532347926509,
0.983778856318835));
#77673=CARTESIAN_POINT('Ctrl Pts',(-6.88446248245522,-3.95187508991586,
-4.32491218431002));
#77674=CARTESIAN_POINT('Ctrl Pts',(-6.76519651003803,1.49932570880582,-5.66340926891253));
#77675=CARTESIAN_POINT('Ctrl Pts',(-6.64593053762087,5.57417165602073,-1.80299541804897));
#77676=CARTESIAN_POINT('Ctrl Pts',(-6.52666456520372,4.53202524004452,3.71253678121714));
#77677=CARTESIAN_POINT('Ctrl Pts',(-6.40739859278654,-0.670441304941221,
5.82002496428659));
#77678=CARTESIAN_POINT('Ctrl Pts',(-6.28813262036937,-5.25745442490609,
2.58483173501215));
#77679=CARTESIAN_POINT('Ctrl Pts',(-6.16886664795223,-5.01821607609671,
-3.02319194592326));
#77680=CARTESIAN_POINT('Ctrl Pts',(-6.04960067553504,-0.172342890253803,
-5.85597814685722));
#77681=CARTESIAN_POINT('Ctrl Pts',(-5.93033470311789,4.83173806307439,-3.31307854089344));
#77682=CARTESIAN_POINT('Ctrl Pts',(-5.81106873070073,5.40036774303056,2.27116938345109));
#77683=CARTESIAN_POINT('Ctrl Pts',(-5.69180275828355,1.01155402067174,5.77052342440038));
#77684=CARTESIAN_POINT('Ctrl Pts',(-5.5725367858664,-4.3058486505297,3.9726376032835));
#77685=CARTESIAN_POINT('Ctrl Pts',(-5.45327081344922,-5.67055735723522,
-1.47206025236609));
#77686=CARTESIAN_POINT('Ctrl Pts',(-5.33400484103207,-1.82979330806154,
-5.56543246999403));
#77687=CARTESIAN_POINT('Ctrl Pts',(-5.21473886861489,3.69068908517426,-4.54983474478646));
#77688=CARTESIAN_POINT('Ctrl Pts',(-5.09547289619774,5.82318326614332,0.642431924174813));
#77689=CARTESIAN_POINT('Ctrl Pts',(-4.97620692378057,2.61009676874675,5.24495729115771));
#77690=CARTESIAN_POINT('Ctrl Pts',(-4.85694095136341,-2.99901304064116,
5.03270334018952));
#77691=CARTESIAN_POINT('Ctrl Pts',(-4.73767497894624,-5.85508118338141,
0.200515496417569));
#77692=CARTESIAN_POINT('Ctrl Pts',(-4.61840900652908,-3.33628691605105,
-4.8157420759502));
#77693=CARTESIAN_POINT('Ctrl Pts',(-4.49914303411192,2.24516055328616,-5.41123241214589));
#77694=CARTESIAN_POINT('Ctrl Pts',(-4.37987706169475,5.76558979170929,-1.03930576926535));
#77695=CARTESIAN_POINT('Ctrl Pts',(-4.26061108927759,3.99330815683104,4.28668544365891));
#77696=CARTESIAN_POINT('Ctrl Pts',(-4.14134511686042,-1.4447607202292,5.67757418177634));
#77697=CARTESIAN_POINT('Ctrl Pts',(-4.02207914444326,-5.55656445364856,
1.85654884146363));
#77698=CARTESIAN_POINT('Ctrl Pts',(-3.90281317202609,-4.56753892857381,
-3.66875595594112));
#77699=CARTESIAN_POINT('Ctrl Pts',(-3.78354719960893,0.614407672199417,
-5.82620677118766));
#77700=CARTESIAN_POINT('Ctrl Pts',(-3.66428122719176,5.2323387455472,-2.63530138316969));
#77701=CARTESIAN_POINT('Ctrl Pts',(-3.5450152547746,5.04707410573905,2.97476471329566));
#77702=CARTESIAN_POINT('Ctrl Pts',(-3.42574928235743,0.228683460987768,
5.85404868471053));
#77703=CARTESIAN_POINT('Ctrl Pts',(-3.30648330994027,-4.79963461256785,
3.35941806182726));
#77704=CARTESIAN_POINT('Ctrl Pts',(-3.1872173375231,-5.42197182041219,-2.21909975146378));
#77705=CARTESIAN_POINT('Ctrl Pts',(-3.06795136510594,-1.06703345969384,
-5.76052269539703));
#77706=CARTESIAN_POINT('Ctrl Pts',(-2.94868539268877,4.26742300729336,-4.01388627207025));
#77707=CARTESIAN_POINT('Ctrl Pts',(-2.82941942027161,5.68445958010836,1.41742774433296));
#77708=CARTESIAN_POINT('Ctrl Pts',(-2.71015344785444,1.88326139891008,5.54756781226383));
#77709=CARTESIAN_POINT('Ctrl Pts',(-2.59088747543728,-3.64673790123239,
4.58513738158476));
#77710=CARTESIAN_POINT('Ctrl Pts',(-2.47162150302012,-5.82909540943063,
-0.586369197728859));
#77711=CARTESIAN_POINT('Ctrl Pts',(-2.35235553060295,-2.66044499483698,
-5.21959908017247));
#77712=CARTESIAN_POINT('Ctrl Pts',(-2.23308955818579,2.95044752519428,-5.06132804008646));
#77713=CARTESIAN_POINT('Ctrl Pts',(-2.11382358576862,5.85288067474523,-0.256846131923952));
#77714=CARTESIAN_POINT('Ctrl Pts',(-1.99455761335146,3.38247144277536,4.78341604578777));
#77715=CARTESIAN_POINT('Ctrl Pts',(-1.8752916409343,-2.1929875812473,5.43258571923035));
#77716=CARTESIAN_POINT('Ctrl Pts',(-1.75602566851713,-5.7553222527583,1.0947364501082));
#77717=CARTESIAN_POINT('Ctrl Pts',(-1.63675969609996,-4.03437147265267,
-4.24806178732573));
#77718=CARTESIAN_POINT('Ctrl Pts',(-1.5174937236828,1.39006195738937,-5.69121339284596));
#77719=CARTESIAN_POINT('Ctrl Pts',(-1.39822775126564,5.53844275409686,-1.90993036205053));
#77720=CARTESIAN_POINT('Ctrl Pts',(-1.27896177884847,4.60262969644498,3.62463543072867));
#77721=CARTESIAN_POINT('Ctrl Pts',(-1.15969580643131,-0.558317149806238,
5.83184911400515));
#77722=CARTESIAN_POINT('Ctrl Pts',(-1.04042983401414,-5.20673858993517,
2.68552702171667));
#77723=CARTESIAN_POINT('Ctrl Pts',(-0.921163861596979,-5.07546481327733,
-2.92606203923883));
#77724=CARTESIAN_POINT('Ctrl Pts',(-0.801897889179813,-0.285002857307873,
-5.85157718052293));
#77725=CARTESIAN_POINT('Ctrl Pts',(-0.68263191676265,4.7670867510423,-3.40544652524855));
#77726=CARTESIAN_POINT('Ctrl Pts',(-0.563365944345483,5.44307386290664,
2.16682464708923));
#77727=CARTESIAN_POINT('Ctrl Pts',(-0.44409997192832,1.12241409923112,5.74998858417455));
#77728=CARTESIAN_POINT('Ctrl Pts',(-0.324833999511155,-4.22860223193546,
4.05476328438059));
#77729=CARTESIAN_POINT('Ctrl Pts',(-0.205568027093992,-5.69783546364988,
-1.36266399287005));
#77730=CARTESIAN_POINT('Ctrl Pts',(-0.0863020546768254,-1.93655511354362,
-5.52918949037728));
#77731=CARTESIAN_POINT('Ctrl Pts',(0.0329639177403375,3.60244905606469,
-4.62001546823699));
#77732=CARTESIAN_POINT('Ctrl Pts',(0.152229890157503,5.83446782116765,0.530252177788952));
#77733=CARTESIAN_POINT('Ctrl Pts',(0.271495862574667,2.71054688320229,5.19375757253385));
#77734=CARTESIAN_POINT('Ctrl Pts',(0.390761834991831,-2.90160881991181,
5.08948409806933));
#77735=CARTESIAN_POINT('Ctrl Pts',(0.510027807408999,-5.85013823221736,
0.313152985359231));
#77736=CARTESIAN_POINT('Ctrl Pts',(0.629293779826159,-3.42834277741273,
-4.75064710632693));
#77737=CARTESIAN_POINT('Ctrl Pts',(0.748559752243327,2.14061155461703,-5.45343600865826));
#77738=CARTESIAN_POINT('Ctrl Pts',(0.867825724660488,5.74452181311114,-1.15006576637208));
#77739=CARTESIAN_POINT('Ctrl Pts',(0.987091697077656,4.07506123521824,4.20904479157825));
#77740=CARTESIAN_POINT('Ctrl Pts',(1.10635766949482,-1.33523448499132,5.70432563923033));
#77741=CARTESIAN_POINT('Ctrl Pts',(1.22562364191199,-5.51980823530243,1.96313503707162));
#77742=CARTESIAN_POINT('Ctrl Pts',(1.34488961432914,-4.63729429450974,-3.5801792908174));
#77743=CARTESIAN_POINT('Ctrl Pts',(1.46415558674632,0.502174931333422,-5.83695147029944));
#77744=CARTESIAN_POINT('Ctrl Pts',(1.58342155916348,5.18065632845705,-2.7355040001266));
#77745=CARTESIAN_POINT('Ctrl Pts',(1.70268753158064,5.10338556993982,2.87708843326382));
#77746=CARTESIAN_POINT('Ctrl Pts',(1.82195350399781,0.341295864450316,5.84856386313765));
#77747=CARTESIAN_POINT('Ctrl Pts',(1.94121947641497,-4.73409749219153,3.45115966925853));
#77748=CARTESIAN_POINT('Ctrl Pts',(2.06048544883214,-5.46367191661918,-2.11434891061935));
#77749=CARTESIAN_POINT('Ctrl Pts',(2.17975142124929,-1.17769081144187,-5.7389220661145));
#77750=CARTESIAN_POINT('Ctrl Pts',(2.29901739366647,4.18938991897566,-4.09526485530251));
#77751=CARTESIAN_POINT('Ctrl Pts',(2.41828336608364,5.71068376935081,1.30777406869979));
#77752=CARTESIAN_POINT('Ctrl Pts',(2.53754933850079,1.98966951735438,5.5102992060324));
#77753=CARTESIAN_POINT('Ctrl Pts',(2.65681531091796,-3.55782665049407,4.65446577528774));
#77754=CARTESIAN_POINT('Ctrl Pts',(2.77608128333512,-5.8393000039083,-0.474086060380299));
#77755=CARTESIAN_POINT('Ctrl Pts',(2.89534725575229,-2.76039779477465,-5.16743516097626));
#77756=CARTESIAN_POINT('Ctrl Pts',(3.01461322816945,2.85250144690018,-5.11716890709337));
#77757=CARTESIAN_POINT('Ctrl Pts',(3.13387920058662,5.84685410972783,-0.369430843121191));
#77758=CARTESIAN_POINT('Ctrl Pts',(3.25314517300378,3.47389667261357,4.71743829173152));
#77759=CARTESIAN_POINT('Ctrl Pts',(3.37241114542095,-2.08803732303183,5.47378134984554));
#77760=CARTESIAN_POINT('Ctrl Pts',(3.4916771178381,-5.73318947280932,1.20528859496755));
#77761=CARTESIAN_POINT('Ctrl Pts',(3.61094309025528,-4.11537367695382,-4.16963806910456));
#77762=CARTESIAN_POINT('Ctrl Pts',(3.73020906267244,1.28028337965748,-5.71690970683145));
#77763=CARTESIAN_POINT('Ctrl Pts',(3.8494750350896,5.50066262268514,-2.01615794016368));
#77764=CARTESIAN_POINT('Ctrl Pts',(3.96874100750677,4.67152951308028,3.53539165252032));
#77765=CARTESIAN_POINT('Ctrl Pts',(4.08800697992393,-0.445986215139254,
5.84151336762971));
#77766=CARTESIAN_POINT('Ctrl Pts',(4.20727295234111,-5.15409437613914,2.78522769089733));
#77767=CARTESIAN_POINT('Ctrl Pts',(4.32653892475825,-5.13083379046902,-2.82784842996788));
#77768=CARTESIAN_POINT('Ctrl Pts',(4.44580489717543,-0.39755727009488,-5.84500901156581));
#77769=CARTESIAN_POINT('Ctrl Pts',(4.56507086959259,4.7006698905792,-3.49655326115484));
#77770=CARTESIAN_POINT('Ctrl Pts',(4.68433684200975,5.483764074321,2.06167740092304));
#77771=CARTESIAN_POINT('Ctrl Pts',(4.80360281442692,1.23285847810731,5.72732416589543));
#77772=CARTESIAN_POINT('Ctrl Pts',(4.92286878684409,-4.14978969918686,4.1353872346871));
#77773=CARTESIAN_POINT('Ctrl Pts',(5.04213475926125,-5.72300330755224,-1.25276305422717));
#77774=CARTESIAN_POINT('Ctrl Pts',(5.16140073167841,-2.04259969233753,-5.49089870833121));
#77775=CARTESIAN_POINT('Ctrl Pts',(5.28066670409558,3.51287481622839,-4.68848511289082));
#77776=CARTESIAN_POINT('Ctrl Pts',(5.39993267651275,5.84359151022793,0.417876046074028));
#77777=CARTESIAN_POINT('Ctrl Pts',(5.51919864892991,2.80999311372474,5.14063428276219));
#77778=CARTESIAN_POINT('Ctrl Pts',(5.63846462134707,-2.80312995314244,5.14437990374799));
#77779=CARTESIAN_POINT('Ctrl Pts',(5.75773059376424,-5.84302861136241,0.425674494292362));
#77780=CARTESIAN_POINT('Ctrl Pts',(5.8769965661814,-3.51912891042079,-4.68379267689455));
#77781=CARTESIAN_POINT('Ctrl Pts',(5.99626253859856,2.03526975448046,-5.49361985896253));
#77782=CARTESIAN_POINT('Ctrl Pts',(6.11552851101573,5.72132628114465,-1.26039982266515));
#77783=CARTESIAN_POINT('Ctrl Pts',(6.23479448343289,4.15530506522249,4.12984526867857));
#77784=CARTESIAN_POINT('Ctrl Pts',(6.35406045585006,-1.2252137294577,5.72896443045676));
#77785=CARTESIAN_POINT('Ctrl Pts',(6.47332642826722,-5.4810076889886,2.06899416179424));
#77786=CARTESIAN_POINT('Ctrl Pts',(6.59259240068438,-4.70533218222602,-3.49027666284472));
#77787=CARTESIAN_POINT('Ctrl Pts',(6.71185837310156,0.389756203887297,-5.8455343835976));
#77788=CARTESIAN_POINT('Ctrl Pts',(6.83112434551871,5.1270551924238,-2.83469348997928));
#77789=CARTESIAN_POINT('Ctrl Pts',(6.95039031793589,5.15780693336066,2.77834658861474));
#77790=CARTESIAN_POINT('Ctrl Pts',(7.06965629035304,0.453781864847495,5.84091295496054));
#77791=CARTESIAN_POINT('Ctrl Pts',(7.18892226277022,-4.66680704135651,3.54162309782339));
#77792=CARTESIAN_POINT('Ctrl Pts',(7.30818823518737,-5.50334847562537,-2.00881499499638));
#77793=CARTESIAN_POINT('Ctrl Pts',(7.42745420760454,-1.28791199110556,-5.71519595739787));
#77794=CARTESIAN_POINT('Ctrl Pts',(7.54672018002171,4.1098052392595,-4.17512670749595));
#77795=CARTESIAN_POINT('Ctrl Pts',(7.66598615243887,5.7347929375551,1.19763604306929));
#77796=CARTESIAN_POINT('Ctrl Pts',(7.78525212485604,2.09534073754652,5.47098979361764));
#77797=CARTESIAN_POINT('Ctrl Pts',(7.9045180972732,-3.46759771547835,4.72207033110479));
#77798=CARTESIAN_POINT('Ctrl Pts',(8.02378406969036,-5.84734194276446,-0.361627339505832));
#77799=CARTESIAN_POINT('Ctrl Pts',(8.14305004210753,-2.85932824788915,-5.11335741945677));
#77800=CARTESIAN_POINT('Ctrl Pts',(8.26231601452469,2.75349891007753,-5.17111456849417));
#77801=CARTESIAN_POINT('Ctrl Pts',(8.38158198694186,5.83866209133414,-0.481878731122364));
#77802=CARTESIAN_POINT('Ctrl Pts',(8.50084795935901,3.56403530266033,4.64971337715362));
#77803=CARTESIAN_POINT('Ctrl Pts',(8.62011393177619,-1.98231373485353,5.51294969910862));
#77804=CARTESIAN_POINT('Ctrl Pts',(8.73937990419334,-5.70893333656173,1.31539434656858));
#77805=CARTESIAN_POINT('Ctrl Pts',(8.85864587661052,-4.19485170267006,-4.08967007482224));
#77806=CARTESIAN_POINT('Ctrl Pts',(8.97791184902767,1.1700306334385,-5.74048869392723));
#77807=CARTESIAN_POINT('Ctrl Pts',(9.09717782144485,5.46084525411568,-2.1216388097159));
#77808=CARTESIAN_POINT('Ctrl Pts',(9.21644379386201,4.73869917206731,3.44483849910834));
#77809=CARTESIAN_POINT('Ctrl Pts',(9.33570976627917,-0.333490104064998,
5.8490141458866));
#77810=CARTESIAN_POINT('Ctrl Pts',(9.45497573869634,-5.0995412809414,2.88389681720152));
#77811=CARTESIAN_POINT('Ctrl Pts',(9.5742417111135,-5.18430250109922,-2.72858749271244));
#77812=CARTESIAN_POINT('Ctrl Pts',(9.69350768353068,-0.509964442722255,
-5.83627607258685));
#77813=CARTESIAN_POINT('Ctrl Pts',(9.81277365594782,4.6325120799753,-3.58636500612715));
#77814=CARTESIAN_POINT('Ctrl Pts',(9.93203962836501,5.52242330716014,1.95576658751111));
#77815=CARTESIAN_POINT('Ctrl Pts',(10.0513056007822,1.34284625288435,5.70253856360527));
#77816=CARTESIAN_POINT('Ctrl Pts',(10.1705715731993,-4.06944024146176,4.2144795941447));
#77817=CARTESIAN_POINT('Ctrl Pts',(10.2898375456165,-5.74605156772597,-1.14239813958374));
#77818=CARTESIAN_POINT('Ctrl Pts',(10.4091035180337,-2.14788776954667,-5.45057430531156));
#77819=CARTESIAN_POINT('Ctrl Pts',(10.5283694904508,3.42199954057199,-4.75521832018421));
#77820=CARTESIAN_POINT('Ctrl Pts',(10.647635462868,5.85055095425527,0.305345148894098));
#77821=CARTESIAN_POINT('Ctrl Pts',(10.7669014352851,2.90839862919574,5.08560709669781));
#77822=CARTESIAN_POINT('Ctrl Pts',(10.8861674077023,-2.70361291317653,5.19737042589766));
#77823=CARTESIAN_POINT('Ctrl Pts',(11.0054333801195,-5.83375495395087,0.538038349510541));
#77824=CARTESIAN_POINT('Ctrl Pts',(11.1246993525366,-3.60861169132913,-4.61520354800236));
#77825=CARTESIAN_POINT('Ctrl Pts',(11.2439653249538,1.92917416749059,-5.53176908048207));
#77826=CARTESIAN_POINT('Ctrl Pts',(11.363231297371,5.69601178655655,-1.37026707458776));
#77827=CARTESIAN_POINT('Ctrl Pts',(11.4824972697881,4.23400992756751,4.04911620746435));
#77828=CARTESIAN_POINT('Ctrl Pts',(11.6017632422053,-1.11473920115039,5.75148143018032));
#77829=CARTESIAN_POINT('Ctrl Pts',(11.7210292146225,-5.44017718496026,2.17408700941989));
#77830=CARTESIAN_POINT('Ctrl Pts',(11.8402951870396,-4.77162739306525,-3.39908136855241));
#77831=CARTESIAN_POINT('Ctrl Pts',(11.9595611594568,0.277193125501102,-5.85195233229607));
#77832=CARTESIAN_POINT('Ctrl Pts',(12.078827131874,5.07155518927873,-2.93283311669634));
#77833=CARTESIAN_POINT('Ctrl Pts',(12.1980931042911,5.21031804038915,2.67857574958897));
#77834=CARTESIAN_POINT('Ctrl Pts',(12.3173590767083,0.566099801623865,5.83109879378591));
#77835=CARTESIAN_POINT('Ctrl Pts',(12.4366250491254,-4.59778818189795,3.63077484329315));
#77836=CARTESIAN_POINT('Ctrl Pts',(12.5558910215426,-5.54098680273559,-1.90253709036138));
#77837=CARTESIAN_POINT('Ctrl Pts',(12.6751569939598,-1.39765617693328,-5.68935315649946));
#77838=CARTESIAN_POINT('Ctrl Pts',(12.794422966377,4.02869844329693,-4.25344225084433));
#77839=CARTESIAN_POINT('Ctrl Pts',(12.9136889387941,5.75677815559816,1.08705445839597));
#77840=CARTESIAN_POINT('Ctrl Pts',(13.0329549112113,2.20023592286751,5.42965413373763));
#77841=CARTESIAN_POINT('Ctrl Pts',(13.1522208836285,-3.37608451356654,4.78792601086807));
#77842=CARTESIAN_POINT('Ctrl Pts',(13.2714868560456,-5.85321824756939,-0.249034685557716));
#77843=CARTESIAN_POINT('Ctrl Pts',(13.3907528284628,-2.95719971408639,-5.057385883962));
#77844=CARTESIAN_POINT('Ctrl Pts',(13.5100188008799,2.65347658151761,-5.22314504485836));
#77845=CARTESIAN_POINT('Ctrl Pts',(13.6292847732971,5.82830765357758,-0.594148149487238));
#77846=CARTESIAN_POINT('Ctrl Pts',(13.7485507457143,3.65285394897987,4.58026638479827));
#77847=CARTESIAN_POINT('Ctrl Pts',(13.8678167181314,-1.87585597272662,5.55007626054603));
#77848=CARTESIAN_POINT('Ctrl Pts',(13.9870826905486,-5.68256282757001,1.42501292590967));
#77849=CARTESIAN_POINT('Ctrl Pts',(14.1063486629658,-4.27277611414985,-4.00818742159612));
#77850=CARTESIAN_POINT('Ctrl Pts',(14.2256146353829,1.05934455217531,-5.76194162136924));
#77851=CARTESIAN_POINT('Ctrl Pts',(14.3448806078001,5.41900539523421,-2.22633390458677));
#77852=CARTESIAN_POINT('Ctrl Pts',(14.4641465802173,4.80411379630757,3.35300950795224));
#77853=CARTESIAN_POINT('Ctrl Pts',(14.5834125526344,-0.220870480883753,
5.85434867077158));
#77854=CARTESIAN_POINT('Ctrl Pts',(14.7026785250516,-5.04309950874287,2.98149785732063));
#77855=CARTESIAN_POINT('Ctrl Pts',(14.8219444974687,-5.23585114238199,-2.62831598996543));
#77856=CARTESIAN_POINT('Ctrl Pts',(14.9412104698859,-0.622182743829148,
-5.82538159793605));
#77857=CARTESIAN_POINT('Ctrl Pts',(15.0604764423031,4.56263856230305,-3.67484849729553));
#77858=CARTESIAN_POINT('Ctrl Pts',(15.1797424147202,5.55903724350795,1.84913143220874));
#77859=CARTESIAN_POINT('Ctrl Pts',(15.2990083871374,1.45233668825476,5.67564095695279));
#77860=CARTESIAN_POINT('Ctrl Pts',(15.4182743595546,-3.98758361715711,4.29201106993799));
#77861=CARTESIAN_POINT('Ctrl Pts',(15.5375403319718,-5.76697170796816,-1.03161012392551));
#77862=CARTESIAN_POINT('Ctrl Pts',(15.6568063043889,-2.25238035045361,-5.40823121595048));
#77863=CARTESIAN_POINT('Ctrl Pts',(15.7760722768061,3.32985688585691,-4.82019037466379));
#77864=CARTESIAN_POINT('Ctrl Pts',(15.8953382492232,5.85534357573511,0.192701163432864));
#77865=CARTESIAN_POINT('Ctrl Pts',(16.0146042216404,3.00572698393825,5.02869639432689));
#77866=CARTESIAN_POINT('Ctrl Pts',(16.1338701940575,-2.60309455735759,5.24843603883532));
#77867=CARTESIAN_POINT('Ctrl Pts',(16.2531361664747,-5.82232069459445,0.650202935696243));
#77868=CARTESIAN_POINT('Ctrl Pts',(16.3724021388919,-3.69675797910371,-4.54490512246668));
#77869=CARTESIAN_POINT('Ctrl Pts',(16.491668111309,1.82236408743567,-5.56786954418967));
#77870=CARTESIAN_POINT('Ctrl Pts',(16.6109340837262,5.66858770487726,-1.47962683146975));
#77871=CARTESIAN_POINT('Ctrl Pts',(16.7302000561434,4.31114667295226,3.96688750692321));
#77872=CARTESIAN_POINT('Ctrl Pts',(16.8494660285605,-1.00385181565173,5.77186829895683));
#77873=CARTESIAN_POINT('Ctrl Pts',(16.9687320009777,-5.39733184529022,2.27837465753701));
#77874=CARTESIAN_POINT('Ctrl Pts',(17.0879979733949,-4.83615537379139,-3.30662718322454));
#77875=CARTESIAN_POINT('Ctrl Pts',(17.207263945812,0.164527385277041,-5.85620293942961));
#77876=CARTESIAN_POINT('Ctrl Pts',(17.3265299182292,5.01417687412153,-3.02988653307605));
#77877=CARTESIAN_POINT('Ctrl Pts',(17.4457958906464,5.26089944289952,2.57781286752749));
#77878=CARTESIAN_POINT('Ctrl Pts',(17.5650618630635,0.678208076468528,5.81912501440749));
#77879=CARTESIAN_POINT('Ctrl Pts',(17.6843278354807,-4.52706647578802,3.71858188723699));
#77880=CARTESIAN_POINT('Ctrl Pts',(17.8035938078979,-5.57657295813861,-1.79555455802603));
#77881=CARTESIAN_POINT('Ctrl Pts',(17.922859780315,-1.50688272383402,-5.66140323461425));
#77882=CARTESIAN_POINT('Ctrl Pts',(18.0421257527322,3.94609956997411,-4.33018248023578));
#77883=CARTESIAN_POINT('Ctrl Pts',(18.1613917251494,5.77663128098768,0.976070269911672));
#77884=CARTESIAN_POINT('Ctrl Pts',(18.2806576975665,2.30431622411275,5.3863075355554));
#77885=CARTESIAN_POINT('Ctrl Pts',(18.3999236699837,-3.28332093778318,4.85200842412762));
#77886=CARTESIAN_POINT('Ctrl Pts',(18.5191896424009,-5.85692674196245,-0.136349798591407));
#77887=CARTESIAN_POINT('Ctrl Pts',(18.638455614818,-3.05397594548137,-4.99954128422911));
#77888=CARTESIAN_POINT('Ctrl Pts',(18.7577215872352,2.55247150570324,-5.2732410660678));
#77889=CARTESIAN_POINT('Ctrl Pts',(18.8769875596523,5.81579463134992,-0.706197517874579));
#77890=CARTESIAN_POINT('Ctrl Pts',(18.9962535320695,3.74031971650885,4.50912303520155));
#77891=CARTESIAN_POINT('Ctrl Pts',(19.1155195044867,-1.76870346457484,5.58514728388534));
#77892=CARTESIAN_POINT('Ctrl Pts',(19.2347854769038,-5.65408771247222,1.53410373442001));
#77893=CARTESIAN_POINT('Ctrl Pts',(19.354051449321,-4.34911805114188,-3.92522028751534));
#77894=CARTESIAN_POINT('Ctrl Pts',(19.4733174217381,0.948266129800921,-5.78126054380557));
#77895=CARTESIAN_POINT('Ctrl Pts',(19.5925833941553,5.37515854194023,-2.33020444967771));
#77896=CARTESIAN_POINT('Ctrl Pts',(19.7118493665725,4.86774915870119,3.25993868903297));
#77897=CARTESIAN_POINT('Ctrl Pts',(19.8311153389897,-0.108169055639234,
5.85751496657865));
#77898=CARTESIAN_POINT('Ctrl Pts',(19.9503813114068,-4.98478996343882,3.07799466352533));
#77899=CARTESIAN_POINT('Ctrl Pts',(20.069647283824,-5.28546062265248,-2.52707105849445));
#77900=CARTESIAN_POINT('Ctrl Pts',(20.1889132562411,-0.734170612006343,
-5.81232962251428));
#77901=CARTESIAN_POINT('Ctrl Pts',(20.3081792286583,4.49107521606757,-3.76197096372558));
#77902=CARTESIAN_POINT('Ctrl Pts',(20.4274452010755,5.59359232294874,1.74181142863946));
#77903=CARTESIAN_POINT('Ctrl Pts',(20.5467111734926,1.5612892331075,5.64664130779292));
#77904=CARTESIAN_POINT('Ctrl Pts',(20.6659771459098,-3.90425014286694,4.36795294734436));
#77905=CARTESIAN_POINT('Ctrl Pts',(20.785243118327,-5.78575598025094,-0.920440038938236));
#77906=CARTESIAN_POINT('Ctrl Pts',(20.9045090907441,-2.35603873496334,-5.36388512252482));
#77907=CARTESIAN_POINT('Ctrl Pts',(21.0237750631613,3.23648097823332,-4.88337721314099));
#77908=CARTESIAN_POINT('Ctrl Pts',(21.1430410355785,5.85796759966182,0.0799858087570004));
#77909=CARTESIAN_POINT('Ctrl Pts',(21.2623070079956,3.10194213121528,4.96992325321854));
#77910=CARTESIAN_POINT('Ctrl Pts',(21.3815729804128,-2.5016121138784,5.29755782979173));
#77911=CARTESIAN_POINT('Ctrl Pts',(21.50083895283,-5.80873006810966,0.762126711334059));
#77912=CARTESIAN_POINT('Ctrl Pts',(21.6201049252471,-3.78353512769747,-4.47292343616231));
#77913=CARTESIAN_POINT('Ctrl Pts',(21.7393708976643,1.71487907272487,-5.60190787984068));
#77914=CARTESIAN_POINT('Ctrl Pts',(21.8586368700815,5.63906419294801,-1.58843859059823));
#77915=CARTESIAN_POINT('Ctrl Pts',(21.9779028424986,4.38668673284723,3.88318962145203));
#77916=CARTESIAN_POINT('Ctrl Pts',(22.0971688149158,-0.892592641450376,
5.79011748626221));
#77917=CARTESIAN_POINT('Ctrl Pts',(22.2164347873329,-5.35248753826974,2.38181848194971));
#77918=CARTESIAN_POINT('Ctrl Pts',(22.3357007597501,-4.89889222568395,-3.21294834839033));
#77919=CARTESIAN_POINT('Ctrl Pts',(22.4549667321672,0.0518007103390068,
-5.85828463073442));
#77920=CARTESIAN_POINT('Ctrl Pts',(22.5742327045845,4.95494149770743,-3.12581779420793));
#77921=CARTESIAN_POINT('Ctrl Pts',(22.6934986770016,5.3095324074556,2.47609526118635));
#77922=CARTESIAN_POINT('Ctrl Pts',(22.8127646494188,0.79006516872153,5.80499605145979));
#77923=CARTESIAN_POINT('Ctrl Pts',(22.9320306218359,-4.45466811566874,3.80501170925063));
#77924=CARTESIAN_POINT('Ctrl Pts',(23.0512965942531,-5.61009376206996,-1.68790702026934));
#77925=CARTESIAN_POINT('Ctrl Pts',(23.1705625666702,-1.61555117843076,-5.63135654333499));
#77926=CARTESIAN_POINT('Ctrl Pts',(23.2898285390874,3.86203921078604,-4.4053189739951));
#77927=CARTESIAN_POINT('Ctrl Pts',(23.4090945115046,5.79434496087777,0.864724581957292));
#77928=CARTESIAN_POINT('Ctrl Pts',(23.5283604839218,2.40754309387953,5.34096605300986));
#77929=CARTESIAN_POINT('Ctrl Pts',(23.6476264563389,-3.18934134424452,4.9142938371838));
#77930=CARTESIAN_POINT('Ctrl Pts',(23.7668924287561,-5.85846605245757,-0.0236144128224182));
#77931=CARTESIAN_POINT('Ctrl Pts',(23.8861584011732,-3.1496210998223,-4.93984504370784));
#77932=CARTESIAN_POINT('Ctrl Pts',(24.0054243735904,2.45052109109024,-5.3213840784529));
#77933=CARTESIAN_POINT('Ctrl Pts',(24.1246903460076,5.80112765900066,-0.817985337440891));
#77934=CARTESIAN_POINT('Ctrl Pts',(24.2439563184247,3.8264002112388,4.43630967716665));
#77935=CARTESIAN_POINT('Ctrl Pts',(24.3632222908419,-1.6608958956302,5.61814978014727));
#77936=CARTESIAN_POINT('Ctrl Pts',(24.482488263259,-5.62351853737269,1.64262636899463));
#77937=CARTESIAN_POINT('Ctrl Pts',(24.6017542356763,-4.42384923948336,-3.84079940046513));
#77938=CARTESIAN_POINT('Ctrl Pts',(24.7210202080934,0.836836505557353,-5.79843830623873));
#77939=CARTESIAN_POINT('Ctrl Pts',(24.8402861805106,5.32932093344786,-2.43321197527163));
#77940=CARTESIAN_POINT('Ctrl Pts',(24.9595521529278,4.92958169111955,3.16566051225803));
#77941=CARTESIAN_POINT('Ctrl Pts',(25.0788181253449,0.00457243132771929,
5.85851186063166));
#77942=CARTESIAN_POINT('Ctrl Pts',(25.1980840977621,-4.92463424067689,3.17335149705221));
#77943=CARTESIAN_POINT('Ctrl Pts',(25.3173500701792,-5.33311256843772,-2.42489019558874));
#77944=CARTESIAN_POINT('Ctrl Pts',(25.4366160425964,-0.845886571187518,
-5.797124980279));
#77945=CARTESIAN_POINT('Ctrl Pts',(25.5558820150136,4.41784854562258,-3.84770013855436));
#77946=CARTESIAN_POINT('Ctrl Pts',(25.6751479874307,5.62607574758965,1.63384632406917));
#77947=CARTESIAN_POINT('Ctrl Pts',(25.7944139598479,1.66966353554507,5.61555035649768));
#77948=CARTESIAN_POINT('Ctrl Pts',(25.9136799322651,-3.81947068215475,4.44227710036768));
#77949=CARTESIAN_POINT('Ctrl Pts',(26.0329459046822,-5.80239742759128,-0.808929057812192));
#77950=CARTESIAN_POINT('Ctrl Pts',(26.1522118770994,-2.45882453193489,-5.31755244914851));
#77951=CARTESIAN_POINT('Ctrl Pts',(26.2714778495165,3.14190640060181,-4.94475543360317));
#77952=CARTESIAN_POINT('Ctrl Pts',(26.3907438219337,5.85842205419648,-0.032759169633832));
#77953=CARTESIAN_POINT('Ctrl Pts',(26.5100097943509,3.19700843657914,4.90930944071892));
#77954=CARTESIAN_POINT('Ctrl Pts',(26.629275766768,-2.39920316799348,5.34471760591528));
#77955=CARTESIAN_POINT('Ctrl Pts',(26.7485417391852,-5.79298810795018,0.873768224095266));
#77956=CARTESIAN_POINT('Ctrl Pts',(26.8678077116024,-3.86891099814006,-4.39928514838047));
#77957=CARTESIAN_POINT('Ctrl Pts',(26.9870736840195,1.60675893173784,-5.63387148092423));
#77958=CARTESIAN_POINT('Ctrl Pts',(27.1063396564367,5.60745218515998,-1.69666205221763));
#77959=CARTESIAN_POINT('Ctrl Pts',(27.2256056288539,4.46060213007431,3.79805354957861));
#77960=CARTESIAN_POINT('Ctrl Pts',(27.344871601271,-0.781002884731814,5.8062222332883));
#77961=CARTESIAN_POINT('Ctrl Pts',(27.4641375736882,-5.3056608725324,2.4843801709822));
#77962=CARTESIAN_POINT('Ctrl Pts',(27.5834035461053,-4.95981471338826,-3.11807955914333));
#77963=CARTESIAN_POINT('Ctrl Pts',(27.7026695185225,-0.0609451496207866,
-5.85819663523071));
#77964=CARTESIAN_POINT('Ctrl Pts',(27.8219354909397,4.89387099857715,-3.22059137078522));
#77965=CARTESIAN_POINT('Ctrl Pts',(27.9412014633569,5.35619892224863,2.37346060291565));
#77966=CARTESIAN_POINT('Ctrl Pts',(28.060467435774,0.901629650751189,5.78871713777561));
#77967=CARTESIAN_POINT('Ctrl Pts',(28.1797334081912,-4.38061991515157,3.89003229900066));
#77968=CARTESIAN_POINT('Ctrl Pts',(28.2989993806083,-5.64153679969301,-1.57963434566348));
#77969=CARTESIAN_POINT('Ctrl Pts',(28.4182653530255,-1.72362129404252,-5.59922421081825));
#77970=CARTESIAN_POINT('Ctrl Pts',(28.5375313254427,3.77654849850695,-4.47882390441015));
#77971=CARTESIAN_POINT('Ctrl Pts',(28.6567972978598,5.8099126347921,0.753058632759737));
#77972=CARTESIAN_POINT('Ctrl Pts',(28.776063270277,2.50987830084389,5.29364647886908));
#77973=CARTESIAN_POINT('Ctrl Pts',(28.8953292426942,-3.09418053943347,4.97475918187826));
#77974=CARTESIAN_POINT('Ctrl Pts',(29.0145952151113,-5.8578356089525,0.0891297188309879));
#77975=CARTESIAN_POINT('Ctrl Pts',(29.1338611875285,-3.24409975376552,-4.87831927162507));
#77976=CARTESIAN_POINT('Ctrl Pts',(29.2531271599456,2.34766309625184,-5.367556251665));
#77977=CARTESIAN_POINT('Ctrl Pts',(29.3723931323628,5.78431216862107,-0.929470206210548));
#77978=CARTESIAN_POINT('Ctrl Pts',(29.49165910478,3.91106355221379,4.36185327800407));
#77979=CARTESIAN_POINT('Ctrl Pts',(29.6109250771972,-1.55247319373407,5.64907152645706));
#77980=CARTESIAN_POINT('Ctrl Pts',(29.7301910496143,-5.59086662393646,1.75054063695882));
#77981=CARTESIAN_POINT('Ctrl Pts',(29.8494570220315,-4.49694200157167,-3.75495602674528));
#77982=CARTESIAN_POINT('Ctrl Pts',(29.9687229944486,0.725096948758073,-5.81346854667612));
#77983=CARTESIAN_POINT('Ctrl Pts',(30.0879889668658,5.28150954627173,-2.53531833128137));
#77984=CARTESIAN_POINT('Ctrl Pts',(30.207254939283,4.98958849313373,3.07020989469409));
#77985=CARTESIAN_POINT('Ctrl Pts',(30.3265209117001,0.117312224839382,5.85733898371898));
#77986=CARTESIAN_POINT('Ctrl Pts',(30.4457868841173,-4.86265461985911,3.26753304134077));
#77987=CARTESIAN_POINT('Ctrl Pts',(30.5650528565344,-5.37878933126115,-2.32181124517074));
#77988=CARTESIAN_POINT('Ctrl Pts',(30.6843188289516,-0.957289246011629,
-5.77977330245411));
#77989=CARTESIAN_POINT('Ctrl Pts',(30.8035848013688,4.34298567135418,-3.93200427094161));
#77990=CARTESIAN_POINT('Ctrl Pts',(30.9228507737859,5.65647548679995,1.52527610468443));
#77991=CARTESIAN_POINT('Ctrl Pts',(31.0421167462031,1.77741945782958,5.58237961797831));
#77992=CARTESIAN_POINT('Ctrl Pts',(31.1613827186203,-3.73327663412274,4.51495600215594));
#77993=CARTESIAN_POINT('Ctrl Pts',(31.2806486910374,-5.81688988662698,-0.697118479992365));
#77994=CARTESIAN_POINT('Ctrl Pts',(31.3999146634546,-2.5606996734012,-5.26925035568949));
#77995=CARTESIAN_POINT('Ctrl Pts',(31.5191806358718,3.04616817980498,-5.00430230388157));
#77996=CARTESIAN_POINT('Ctrl Pts',(31.6384466082889,5.85670677102611,-0.145492015268766));
#77997=CARTESIAN_POINT('Ctrl Pts',(31.7577125807061,3.29089069107016,4.84687740588913));
#77998=CARTESIAN_POINT('Ctrl Pts',(31.8769785531233,-2.2959056480988,5.38989790101063));
#77999=CARTESIAN_POINT('Ctrl Pts',(31.9962445255404,-5.77510064434174,0.985086126190849));
#78000=CARTESIAN_POINT('Ctrl Pts',(32.1155104979576,-3.95285397044202,-4.3240175319547));
#78001=CARTESIAN_POINT('Ctrl Pts',(32.2347764703747,1.49804370808096,-5.66374850933283));
#78002=CARTESIAN_POINT('Ctrl Pts',(32.3540424427919,5.57376338940363,-1.80425713445558));
#78003=CARTESIAN_POINT('Ctrl Pts',(32.4733084152091,4.53286548916933,3.71151082248032));
#78004=CARTESIAN_POINT('Ctrl Pts',(32.5925743876263,-0.669123874116674,
5.82017657544665));
#78005=CARTESIAN_POINT('Ctrl Pts',(32.7118403600434,-5.25686919090186,2.58602173966828));
#78006=CARTESIAN_POINT('Ctrl Pts',(32.8311063324606,-5.01890027352189,-3.02205595129089));
#78007=CARTESIAN_POINT('Ctrl Pts',(32.9503723048778,-0.173668437804856,
-5.85593898550875));
#78008=CARTESIAN_POINT('Ctrl Pts',(33.0696382772949,4.83098799493092,-3.31417216226366));
#78009=CARTESIAN_POINT('Ctrl Pts',(33.1889042497121,5.40088170376875,2.26994690470652));
#78010=CARTESIAN_POINT('Ctrl Pts',(33.3081702221293,1.01286020329767,5.77029430244824));
#78011=CARTESIAN_POINT('Ctrl Pts',(33.4274361945464,-4.30494929888592,3.97361216807977));
#78012=CARTESIAN_POINT('Ctrl Pts',(33.5467021669636,-5.67089042569741,-1.47077663430731));
#78013=CARTESIAN_POINT('Ctrl Pts',(33.6659681393807,-1.83105304559022,-5.56501813766366));
#78014=CARTESIAN_POINT('Ctrl Pts',(33.7852341117979,3.68965909565966,-4.5506700480375));
#78015=CARTESIAN_POINT('Ctrl Pts',(33.904500084215,5.82332853705378,0.641113779158535));
#78016=CARTESIAN_POINT('Ctrl Pts',(34.0237660566323,2.6112839439197,5.24436633851196));
#78017=CARTESIAN_POINT('Ctrl Pts',(34.1430320290494,-2.99787376730876,5.03338206413637));
#78018=CARTESIAN_POINT('Ctrl Pts',(34.2622980014666,-5.85503564494024,0.201840840211394));
#78019=CARTESIAN_POINT('Ctrl Pts',(34.3815639738837,-3.3373769159937,-4.81498675479765));
#78020=CARTESIAN_POINT('Ctrl Pts',(34.5008299463009,2.24393561589265,-5.41174048527879));
#78021=CARTESIAN_POINT('Ctrl Pts',(34.6200959187181,5.76535438803626,-1.04061083440989));
#78022=CARTESIAN_POINT('Ctrl Pts',(34.7393618911352,3.99427838333004,4.28578141354626));
#78023=CARTESIAN_POINT('Ctrl Pts',(34.8586278635524,-1.44347551453501,5.67790107056843));
#78024=CARTESIAN_POINT('Ctrl Pts',(34.9778938359695,-5.55614406522461,1.85780657095742));
#78025=CARTESIAN_POINT('Ctrl Pts',(35.0971598083867,-4.56836926656086,-3.66772195949845));
#78026=CARTESIAN_POINT('Ctrl Pts',(35.2164257808039,0.613088843400821,-5.82634569847212));
#78027=CARTESIAN_POINT('Ctrl Pts',(35.335691753221,5.23174208813583,-2.6364857014042));
#78028=CARTESIAN_POINT('Ctrl Pts',(35.4549577256382,5.0477473401233,2.97362218768447));
#78029=CARTESIAN_POINT('Ctrl Pts',(35.5742236980554,0.230008571053462,5.85399677013775));
#78030=CARTESIAN_POINT('Ctrl Pts',(35.6934896704726,-4.79887405723636,3.36050441528738));
#78031=CARTESIAN_POINT('Ctrl Pts',(35.8127556428897,-5.42247399162274,-2.21787238411221));
#78032=CARTESIAN_POINT('Ctrl Pts',(35.9320216153069,-1.0683373820018,-5.76028101481488));
#78033=CARTESIAN_POINT('Ctrl Pts',(36.051287587724,4.26651432885973,-4.01485213902346));
#78034=CARTESIAN_POINT('Ctrl Pts',(36.1705535601412,5.68478026414927,1.41614098305311));
#78035=CARTESIAN_POINT('Ctrl Pts',(36.2898195325583,1.88451712452022,5.54714137311024));
#78036=CARTESIAN_POINT('Ctrl Pts',(36.4090855049756,-3.64569998497971,4.58596274338194));
#78037=CARTESIAN_POINT('Ctrl Pts',(36.5283514773927,-5.82922786986728,-0.585049731431784));
#78038=CARTESIAN_POINT('Ctrl Pts',(36.6476174498099,-2.66162665665066,-5.2189967018826));
#78039=CARTESIAN_POINT('Ctrl Pts',(36.766883422227,2.94930220667439,-5.06199582616066));
#78040=CARTESIAN_POINT('Ctrl Pts',(36.8861493946442,5.85282156297383,-0.258170869634671));
#78041=CARTESIAN_POINT('Ctrl Pts',(37.0054153670614,3.383555686377,4.7826500688436));
#78042=CARTESIAN_POINT('Ctrl Pts',(37.1246813394785,-2.19176077869031,5.43308236633426));
#78043=CARTESIAN_POINT('Ctrl Pts',(37.2439473118957,-5.75506866675922,1.09603845971515));
#78044=CARTESIAN_POINT('Ctrl Pts',(37.3632132843128,-4.03534365880062,-4.24714707669714));
#78045=CARTESIAN_POINT('Ctrl Pts',(37.48247925673,1.38879399537905,-5.69153053311651));
#78046=CARTESIAN_POINT('Ctrl Pts',(37.6017452291472,5.53797166977889,-1.91117898649279));
#78047=CARTESIAN_POINT('Ctrl Pts',(37.7210112015643,4.60352338587549,3.62358399241559));
#78048=CARTESIAN_POINT('Ctrl Pts',(37.8402771739815,-0.557136342626843,
5.83199338805448));
#78049=CARTESIAN_POINT('Ctrl Pts',(37.9595431463987,-5.20586598536909,2.68667127376048));
#78050=CARTESIAN_POINT('Ctrl Pts',(38.0788091188158,-5.0766295927031,-2.92484800376138));
#78051=CARTESIAN_POINT('Ctrl Pts',(38.198075091233,-0.285372479780323,-5.85163608426362));
#78052=CARTESIAN_POINT('Ctrl Pts',(38.3173410636502,4.76449886846839,-3.40629125216186));
#78053=CARTESIAN_POINT('Ctrl Pts',(38.4366070360673,5.44704213670987,2.16515129303516));
#78054=CARTESIAN_POINT('Ctrl Pts',(38.5558730084845,1.11688027088538,5.75054041079176));
#78055=CARTESIAN_POINT('Ctrl Pts',(38.6552613188321,-3.32448407322045,4.33716932787563));
#78056=CARTESIAN_POINT('Ctrl Pts',(38.7347719671102,-4.97744277966909,1.34445408741869));
#78057=CARTESIAN_POINT('Ctrl Pts',(38.7745272912493,-5.01009358722135,-0.348796856848898));
#78058=CARTESIAN_POINT('Ctrl Pts',(38.7944049533188,-4.8183901140079,-1.1511875213148));
#78059=CARTESIAN_POINT('Ctrl Pts',(38.0164112878558,-4.94597286168509,0.000644103793583921));
#78060=CARTESIAN_POINT('Ctrl Pts',(38.0372105648425,-4.94504990619645,-0.865885476849175));
#78061=CARTESIAN_POINT('Ctrl Pts',(38.0580098418292,-4.72867855578625,-1.73287776724594));
#78062=CARTESIAN_POINT('Ctrl Pts',(38.0788091188158,-4.29962613932685,-2.47739280425836));
#78063=CARTESIAN_POINT('Ctrl Pts',(38.1185644429549,-3.47954388839537,-3.90044403059553));
#78064=CARTESIAN_POINT('Ctrl Pts',(38.1583197670939,-1.88245818408785,-4.87604005742951));
#78065=CARTESIAN_POINT('Ctrl Pts',(38.198075091233,-0.242270107226094,-4.95628059882961));
#78066=CARTESIAN_POINT('Ctrl Pts',(38.237830415372,1.39791796963594,-5.03652114022972));
#78067=CARTESIAN_POINT('Ctrl Pts',(38.2775857395111,3.08120841905215,-4.22140619619581));
#78068=CARTESIAN_POINT('Ctrl Pts',(38.3173410636502,4.0366108551339,-2.8852749666459));
#78069=CARTESIAN_POINT('Ctrl Pts',(38.3570963877892,4.99201329121554,-1.54914373709615));
#78070=CARTESIAN_POINT('Ctrl Pts',(38.3968517119283,5.21952771396271,0.308003777969546));
#78071=CARTESIAN_POINT('Ctrl Pts',(38.4366070360673,4.61159128103222,1.83414238846176));
#78072=CARTESIAN_POINT('Ctrl Pts',(38.4730713573782,4.05398069912805,3.23394505296223));
#78073=CARTESIAN_POINT('Ctrl Pts',(38.5095356786891,2.79351375556776,4.3552732712842));
#78074=CARTESIAN_POINT('Ctrl Pts',(38.546,1.34632304271355,4.77431539461067));
#78075=CARTESIAN_POINT('',(-17.6184,-2.62535040627153,-3.68399909158375));
#78076=CARTESIAN_POINT('Ctrl Pts',(-17.6184,-2.63197694108733,-3.68657593761835));
#78077=CARTESIAN_POINT('Ctrl Pts',(-17.6184,-2.73716117210554,-3.61958470141671));
#78078=CARTESIAN_POINT('Ctrl Pts',(-17.6184,-2.83916784935626,-3.54816356962529));
#78079=CARTESIAN_POINT('Ctrl Pts',(-17.6184,-2.93765889762381,-3.47237117351613));
#78080=CARTESIAN_POINT('Ctrl Pts',(-17.6184,-3.0439083914269,-3.39060837514641));
#78081=CARTESIAN_POINT('Ctrl Pts',(-17.6184,-3.14606771222116,-3.30375913852623));
#78082=CARTESIAN_POINT('Ctrl Pts',(-17.6184,-3.24404505736733,-3.21224748954631));
#78083=CARTESIAN_POINT('Ctrl Pts',(-17.6184,-3.30825262600525,-3.15227709052925));
#78084=CARTESIAN_POINT('Ctrl Pts',(-17.6184,-3.37066364900808,-3.09030339612478));
#78085=CARTESIAN_POINT('Ctrl Pts',(-17.6184,-3.43124502544207,-3.02643626197717));
#78086=CARTESIAN_POINT('Ctrl Pts',(-17.6184,-3.45627312892573,-3.00005070693135));
#78087=CARTESIAN_POINT('Ctrl Pts',(-17.6184,-3.4809888798162,-2.97334190334144));
#78088=CARTESIAN_POINT('Ctrl Pts',(-17.6184,-3.50538962958215,-2.94631727874148));
#78089=CARTESIAN_POINT('Ctrl Pts',(-17.6184,-3.52549305907404,-2.92405207622101));
#78090=CARTESIAN_POINT('Ctrl Pts',(-17.6184,-3.54538564420158,-2.90156890295012));
#78091=CARTESIAN_POINT('Ctrl Pts',(-17.6184,-3.56504672982455,-2.87889429908813));
#78092=CARTESIAN_POINT('Ctrl Pts',(-17.6184,-3.65439596746517,-2.77585021455875));
#78093=CARTESIAN_POINT('Ctrl Pts',(-17.6184,-3.7390390925291,-2.66877877171196));
#78094=CARTESIAN_POINT('Ctrl Pts',(-17.6184,-3.81888410590975,-2.55811744250654));
#78095=CARTESIAN_POINT('Ctrl Pts',(-17.6184,-3.90082700708385,-2.44454854222162));
#78096=CARTESIAN_POINT('Ctrl Pts',(-17.6184,-3.97771685155179,-2.32719808251997));
#78097=CARTESIAN_POINT('Ctrl Pts',(-17.6184,-4.04941690653803,-2.20649857516439));
#78098=CARTESIAN_POINT('Ctrl Pts',(-17.6184,-4.08078568059451,-2.15369254069632));
#78099=CARTESIAN_POINT('Ctrl Pts',(-17.6184,-4.11116057774341,-2.10024501648371));
#78100=CARTESIAN_POINT('Ctrl Pts',(-17.6184,-4.14052760413295,-2.04619031750335));
#78101=CARTESIAN_POINT('Ctrl Pts',(-17.6184,-4.16412477109697,-2.00275596565207));
#78102=CARTESIAN_POINT('Ctrl Pts',(-17.6184,-4.18707117346303,-1.95892956580614));
#78103=CARTESIAN_POINT('Ctrl Pts',(-17.6184,-4.20935877075171,-1.91472849022619));
#78104=CARTESIAN_POINT('Ctrl Pts',(-17.6184,-4.21851295458813,-1.8965737844324));
#78105=CARTESIAN_POINT('Ctrl Pts',(-17.6184,-4.22755205088212,-1.87836365074964));
#78106=CARTESIAN_POINT('Ctrl Pts',(-17.6184,-4.23647441528938,-1.86010226714326));
#78107=CARTESIAN_POINT('Ctrl Pts',(-17.6184,-4.29849811267229,-1.73315850213925));
#78108=CARTESIAN_POINT('Ctrl Pts',(-17.6184,-4.35490596821788,-1.60369781509999));
#78109=CARTESIAN_POINT('Ctrl Pts',(-17.6184,-4.4055941948389,-1.47217017248125));
#78110=CARTESIAN_POINT('Ctrl Pts',(-17.6184,-4.45675075636739,-1.33942727751611));
#78111=CARTESIAN_POINT('Ctrl Pts',(-17.6184,-4.50208192177669,-1.204578337258));
#78112=CARTESIAN_POINT('Ctrl Pts',(-17.6184,-4.54143888287325,-1.06805365986625));
#78113=CARTESIAN_POINT('Ctrl Pts',(-17.6184,-4.58077531682645,-0.931600188724784));
#78114=CARTESIAN_POINT('Ctrl Pts',(-17.6184,-4.61414414231629,-0.793471953457049));
#78115=CARTESIAN_POINT('Ctrl Pts',(-17.6184,-4.64134914051464,-0.654077827943033));
#78116=CARTESIAN_POINT('Ctrl Pts',(-17.6184,-4.66175288916341,-0.54953223380752));
#78117=CARTESIAN_POINT('Ctrl Pts',(-17.6184,-4.6786885469106,-0.444274077934729));
#78118=CARTESIAN_POINT('Ctrl Pts',(-17.6184,-4.69205381237269,-0.338472159449352));
#78119=CARTESIAN_POINT('Ctrl Pts',(-17.6184,-4.69780146049362,-0.292972711668202));
#78120=CARTESIAN_POINT('Ctrl Pts',(-17.6184,-4.70288858877598,-0.247372681820807));
#78121=CARTESIAN_POINT('Ctrl Pts',(-17.6184,-4.70730603495934,-0.201685461789799));
#78122=CARTESIAN_POINT('Ctrl Pts',(-17.6184,-4.70953517448911,-0.178630695766913));
#78123=CARTESIAN_POINT('Ctrl Pts',(-17.6184,-4.71159393181158,-0.155550821171334));
#78124=CARTESIAN_POINT('Ctrl Pts',(-17.6184,-4.71347929372106,-0.132472198343172));
#78125=CARTESIAN_POINT('Ctrl Pts',(-17.6184,-4.72517039895951,0.0106380484937822));
#78126=CARTESIAN_POINT('Ctrl Pts',(-17.6184,-4.73021838483544,0.153891258577337));
#78127=CARTESIAN_POINT('Ctrl Pts',(-17.6184,-4.72847670664429,0.29686064475732));
#78128=CARTESIAN_POINT('Ctrl Pts',(-17.6184,-4.7271730108818,0.403877304824889));
#78129=CARTESIAN_POINT('Ctrl Pts',(-17.6184,-4.72206419852149,0.510735518131823));
#78130=CARTESIAN_POINT('Ctrl Pts',(-17.6184,-4.71307035555621,0.617261392298407));
#78131=CARTESIAN_POINT('Ctrl Pts',(-17.6184,-4.70132235933636,0.756408314460109));
#78132=CARTESIAN_POINT('Ctrl Pts',(-17.6184,-4.68294770909115,0.894988563534377));
#78133=CARTESIAN_POINT('Ctrl Pts',(-17.6184,-4.65822406848993,1.03262123260427));
#78134=CARTESIAN_POINT('Ctrl Pts',(-17.6184,-4.63316934564393,1.17209698513291));
#78135=CARTESIAN_POINT('Ctrl Pts',(-17.6184,-4.60159422545019,1.31060035998519));
#78136=CARTESIAN_POINT('Ctrl Pts',(-17.6184,-4.56373468707362,1.44772796830018));
#78137=CARTESIAN_POINT('Ctrl Pts',(-17.6184,-4.55297010560545,1.48671738482605));
#78138=CARTESIAN_POINT('Ctrl Pts',(-17.6184,-4.54169715893265,1.52559549794463));
#78139=CARTESIAN_POINT('Ctrl Pts',(-17.6184,-4.52992054380946,1.56435280087288));
#78140=CARTESIAN_POINT('Ctrl Pts',(-17.6184,-4.52310938075615,1.58676860600784));
#78141=CARTESIAN_POINT('Ctrl Pts',(-17.6184,-4.51612973269326,1.60914399728935));
#78142=CARTESIAN_POINT('Ctrl Pts',(-17.6184,-4.50898246146665,1.63147711431087));
#78143=CARTESIAN_POINT('Ctrl Pts',(-17.6184,-4.50302481877714,1.6500929926144));
#78144=CARTESIAN_POINT('Ctrl Pts',(-17.6184,-4.49695039804118,1.66868024935221));
#78145=CARTESIAN_POINT('Ctrl Pts',(-17.6184,-4.49076502234239,1.68722232347077));
#78146=CARTESIAN_POINT('Ctrl Pts',(-17.6184,-4.44573327332057,1.82221525982782));
#78147=CARTESIAN_POINT('Ctrl Pts',(-17.6184,-4.39476378955444,1.95500777029891));
#78148=CARTESIAN_POINT('Ctrl Pts',(-17.6184,-4.3381737036556,2.08521764827832));
#78149=CARTESIAN_POINT('Ctrl Pts',(-17.6184,-4.2796106428686,2.21996720516727));
#78150=CARTESIAN_POINT('Ctrl Pts',(-17.6184,-4.2150281457401,2.35195174008015));
#78151=CARTESIAN_POINT('Ctrl Pts',(-17.6184,-4.14472053045541,2.48074070343891));
#78152=CARTESIAN_POINT('Ctrl Pts',(-17.6184,-4.07441291517072,2.60952966679768));
#78153=CARTESIAN_POINT('Ctrl Pts',(-17.6184,-3.9983797687207,2.73512390207661));
#78154=CARTESIAN_POINT('Ctrl Pts',(-17.6184,-3.91686351059182,2.85707332817252));
#78155=CARTESIAN_POINT('Ctrl Pts',(-17.6184,-3.8601159990715,2.94196837391093));
#78156=CARTESIAN_POINT('Ctrl Pts',(-17.6184,-3.80071014382092,3.02509662626796));
#78157=CARTESIAN_POINT('Ctrl Pts',(-17.6184,-3.73873295306836,3.10635975427808));
#78158=CARTESIAN_POINT('Ctrl Pts',(-17.6184,-3.71153664712141,3.14201895187533));
#78159=CARTESIAN_POINT('Ctrl Pts',(-17.6184,-3.68384508470585,3.17731890463176));
#78160=CARTESIAN_POINT('Ctrl Pts',(-17.6184,-3.65566502692804,3.21225077861425));
#78161=CARTESIAN_POINT('Ctrl Pts',(-17.6184,-3.63992931102603,3.23175670188976));
#78162=CARTESIAN_POINT('Ctrl Pts',(-17.6184,-3.62404127145717,3.25114784869207));
#78163=CARTESIAN_POINT('Ctrl Pts',(-17.6184,-3.60800203978635,3.2704226332339));
#78164=CARTESIAN_POINT('Ctrl Pts',(-17.6184,-3.59510956928472,3.28591586858525));
#78165=CARTESIAN_POINT('Ctrl Pts',(-17.6184,-3.58211862855319,3.30133475112244));
#78166=CARTESIAN_POINT('Ctrl Pts',(-17.6184,-3.56904120736592,3.31666531967021));
#78167=CARTESIAN_POINT('Ctrl Pts',(-17.6184,-3.47465808930856,3.4273099827433));
#78168=CARTESIAN_POINT('Ctrl Pts',(-17.6184,-3.37564227864469,3.53351659865466));
#78169=CARTESIAN_POINT('Ctrl Pts',(-17.6184,-3.27231843400203,3.63505679843972));
#78170=CARTESIAN_POINT('Ctrl Pts',(-17.6184,-3.16806457753583,3.73751095556628));
#78171=CARTESIAN_POINT('Ctrl Pts',(-17.6184,-3.05942437423569,3.83521489577629));
#78172=CARTESIAN_POINT('Ctrl Pts',(-17.6184,-2.94668631586489,3.92790671043383));
#78173=CARTESIAN_POINT('Ctrl Pts',(-17.6184,-2.83436660052935,4.02025456870566));
#78174=CARTESIAN_POINT('Ctrl Pts',(-17.6184,-2.717978894366,4.10762796058369));
#78175=CARTESIAN_POINT('Ctrl Pts',(-17.6184,-2.59777092570975,4.18973263300831));
#78176=CARTESIAN_POINT('Ctrl Pts',(-17.6184,-2.47949248010661,4.2705193989748));
#78177=CARTESIAN_POINT('Ctrl Pts',(-17.6184,-2.35751491506182,4.34620565556445));
#78178=CARTESIAN_POINT('Ctrl Pts',(-17.6184,-2.23204533204169,4.41646995878763));
#78179=CARTESIAN_POINT('Ctrl Pts',(-17.6184,-2.19381761648338,4.43787788677195));
#78180=CARTESIAN_POINT('Ctrl Pts',(-17.6184,-2.15526556691906,4.45878218778325));
#78181=CARTESIAN_POINT('Ctrl Pts',(-17.6184,-2.11639460593215,4.47917290043388));
#78182=CARTESIAN_POINT('Ctrl Pts',(-17.6184,-2.63197694108751,-3.68657593761822));
#78183=CARTESIAN_POINT('Ctrl Pts',(-17.5819356786891,-1.50670517901651,
-4.47812843616949));
#78184=CARTESIAN_POINT('Ctrl Pts',(-17.5057160332392,1.66816188487742,-5.01601419576036));
#78185=CARTESIAN_POINT('Ctrl Pts',(-17.3897410636502,5.14844039432527,-1.44815814548532));
#78186=CARTESIAN_POINT('Ctrl Pts',(-17.270475091233,4.00553813139823,3.54623540470151));
#78187=CARTESIAN_POINT('Ctrl Pts',(-17.1512091188158,-0.816602122674766,
5.28738771244033));
#78188=CARTESIAN_POINT('Ctrl Pts',(-17.0550486435592,-4.09920106397465,
2.77690491316815));
#78189=CARTESIAN_POINT('Ctrl Pts',(-16.9986434924416,-4.51947609461455,
0.635058848558144));
#78190=CARTESIAN_POINT('Ctrl Pts',(-16.9819936654631,-4.51703452062264,
0.00191132365274384));
#78191=CARTESIAN_POINT('Origin',(-17.6184,-1.12989188470299E-15,0.));
#78192=CARTESIAN_POINT('',(-17.6184,-4.954,-6.06690024297599E-16));
#78193=CARTESIAN_POINT('Origin',(-17.6184,0.,0.));
#78194=CARTESIAN_POINT('Origin',(-17.6184,0.,0.));
#78195=CARTESIAN_POINT('',(-17.6184,2.62535040627109,-3.68399909158407));
#78196=CARTESIAN_POINT('Ctrl Pts',(-17.6184,2.12303769703984,4.48323345254434));
#78197=CARTESIAN_POINT('Ctrl Pts',(-17.6184,2.24381940709171,4.4207770582956));
#78198=CARTESIAN_POINT('Ctrl Pts',(-17.6184,2.36160609121881,4.35319682073143));
#78199=CARTESIAN_POINT('Ctrl Pts',(-17.6184,2.4760271263133,4.28047879555117));
#78200=CARTESIAN_POINT('Ctrl Pts',(-17.6184,2.59817096823974,4.20285269327472));
#78201=CARTESIAN_POINT('Ctrl Pts',(-17.6184,2.71648030536387,4.11937188811111));
#78202=CARTESIAN_POINT('Ctrl Pts',(-17.6184,2.83077226006603,4.0304564910319));
#78203=CARTESIAN_POINT('Ctrl Pts',(-17.6184,2.90276609647662,3.97444764449161));
#78204=CARTESIAN_POINT('Ctrl Pts',(-17.6184,2.9731652237438,3.91628154560514));
#78205=CARTESIAN_POINT('Ctrl Pts',(-17.6184,3.04191642491439,3.85605590927701));
#78206=CARTESIAN_POINT('Ctrl Pts',(-17.6184,3.0824756587865,3.8205262657604));
#78207=CARTESIAN_POINT('Ctrl Pts',(-17.6184,3.12246124783005,3.78427974006281));
#78208=CARTESIAN_POINT('Ctrl Pts',(-17.6184,3.16186122468888,3.74733565762945));
#78209=CARTESIAN_POINT('Ctrl Pts',(-17.6184,3.17680182420591,3.73332634127531));
#78210=CARTESIAN_POINT('Ctrl Pts',(-17.6184,3.19165673930132,3.71921803818185));
#78211=CARTESIAN_POINT('Ctrl Pts',(-17.6184,3.20641884358392,3.70501824795818));
#78212=CARTESIAN_POINT('Ctrl Pts',(-17.6184,3.31072331864878,3.60468691057177));
#78213=CARTESIAN_POINT('Ctrl Pts',(-17.6184,3.41049168111438,3.49970317250891));
#78214=CARTESIAN_POINT('Ctrl Pts',(-17.6184,3.50554675464997,3.39048828312545));
#78215=CARTESIAN_POINT('Ctrl Pts',(-17.6184,3.60030478700596,3.28161468346346));
#78216=CARTESIAN_POINT('Ctrl Pts',(-17.6184,3.69037927330835,3.16853559672437));
#78217=CARTESIAN_POINT('Ctrl Pts',(-17.6184,3.77555511792418,3.05163746945272));
#78218=CARTESIAN_POINT('Ctrl Pts',(-17.6184,3.81405934856761,2.99879299841104));
#78219=CARTESIAN_POINT('Ctrl Pts',(-17.6184,3.85156195266768,2.94516773799131));
#78220=CARTESIAN_POINT('Ctrl Pts',(-17.6184,3.88804011199047,2.89079592116327));
#78221=CARTESIAN_POINT('Ctrl Pts',(-17.6184,3.90826393821039,2.86065168704605));
#78222=CARTESIAN_POINT('Ctrl Pts',(-17.6184,3.92817284751982,2.83027797047312));
#78223=CARTESIAN_POINT('Ctrl Pts',(-17.6184,3.94776269178357,2.79968051659357));
#78224=CARTESIAN_POINT('Ctrl Pts',(-17.6184,3.95882030543706,2.78240958685949));
#78225=CARTESIAN_POINT('Ctrl Pts',(-17.6184,3.96977625803069,2.76506737090552));
#78226=CARTESIAN_POINT('Ctrl Pts',(-17.6184,3.98062977664469,2.74765489470299));
#78227=CARTESIAN_POINT('Ctrl Pts',(-17.6184,3.99133694893152,2.73047720429022));
#78228=CARTESIAN_POINT('Ctrl Pts',(-17.6184,4.00193956608098,2.71323892588693));
#78229=CARTESIAN_POINT('Ctrl Pts',(-17.6184,4.0124361625168,2.69594287926482));
#78230=CARTESIAN_POINT('Ctrl Pts',(-17.6184,4.08795407340856,2.57150622824435));
#78231=CARTESIAN_POINT('Ctrl Pts',(-17.6184,4.15800542572808,2.44405359890784));
#78232=CARTESIAN_POINT('Ctrl Pts',(-17.6184,4.22240808518171,2.31399496854479));
#78233=CARTESIAN_POINT('Ctrl Pts',(-17.6184,4.28677631677449,2.18400586388871));
#78234=CARTESIAN_POINT('Ctrl Pts',(-17.6184,4.34550224287882,2.05141278203371));
#78235=CARTESIAN_POINT('Ctrl Pts',(-17.6184,4.39835791748156,1.91660140410854));
#78236=CARTESIAN_POINT('Ctrl Pts',(-17.6184,4.45114294408316,1.78197021789321));
#78237=CARTESIAN_POINT('Ctrl Pts',(-17.6184,4.49807375121929,1.64512592017646));
#78238=CARTESIAN_POINT('Ctrl Pts',(-17.6184,4.53887208607825,1.50644031813667));
#78239=CARTESIAN_POINT('Ctrl Pts',(-17.6184,4.56947083722247,1.40242611660682));
#78240=CARTESIAN_POINT('Ctrl Pts',(-17.6184,4.59661905930676,1.29737586205953));
#78241=CARTESIAN_POINT('Ctrl Pts',(-17.6184,4.62017859187827,1.191445622251));
#78242=CARTESIAN_POINT('Ctrl Pts',(-17.6184,4.62970711520508,1.148602719576));
#78243=CARTESIAN_POINT('Ctrl Pts',(-17.6184,4.63864840540407,1.10561588280141));
#78244=CARTESIAN_POINT('Ctrl Pts',(-17.6184,4.64699243736825,1.06249551694592));
#78245=CARTESIAN_POINT('Ctrl Pts',(-17.6184,4.65040106524143,1.04488037817516));
#78246=CARTESIAN_POINT('Ctrl Pts',(-17.6184,4.65371013823636,1.02724228268309));
#78247=CARTESIAN_POINT('Ctrl Pts',(-17.6184,4.65691857348069,1.00958400498525));
#78248=CARTESIAN_POINT('Ctrl Pts',(-17.6184,4.68219783989241,0.87045440681626));
#78249=CARTESIAN_POINT('Ctrl Pts',(-17.6184,4.70113960444395,0.730593445780796));
#78250=CARTESIAN_POINT('Ctrl Pts',(-17.6184,4.71353612598034,0.59035734446077));
#78251=CARTESIAN_POINT('Ctrl Pts',(-17.6184,4.72428327942915,0.468779779695929));
#78252=CARTESIAN_POINT('Ctrl Pts',(-17.6184,4.73011040694146,0.346919744006319));
#78253=CARTESIAN_POINT('Ctrl Pts',(-17.6184,4.73085060001627,0.225005660692869));
#78254=CARTESIAN_POINT('Ctrl Pts',(-17.6184,4.73170563360439,0.0841766801921896));
#78255=CARTESIAN_POINT('Ctrl Pts',(-17.6184,4.72577375269981,-0.0567251366648641));
#78256=CARTESIAN_POINT('Ctrl Pts',(-17.6184,4.71325836366559,-0.197256136884384));
#78257=CARTESIAN_POINT('Ctrl Pts',(-17.6184,4.70068788818754,-0.338405683840902));
#78258=CARTESIAN_POINT('Ctrl Pts',(-17.6184,4.68147549611962,-0.479181965102924));
#78259=CARTESIAN_POINT('Ctrl Pts',(-17.6184,4.65577743932771,-0.619119634047808));
#78260=CARTESIAN_POINT('Ctrl Pts',(-17.6184,4.64747570444936,-0.664326376194986));
#78261=CARTESIAN_POINT('Ctrl Pts',(-17.6184,4.6384967543993,-0.709445425498875));
#78262=CARTESIAN_POINT('Ctrl Pts',(-17.6184,4.62884483854091,-0.754460522413662));
#78263=CARTESIAN_POINT('Ctrl Pts',(-17.6184,4.62503524587868,-0.772227894758371));
#78264=CARTESIAN_POINT('Ctrl Pts',(-17.6184,4.62112080895723,-0.789979069125397));
#78265=CARTESIAN_POINT('Ctrl Pts',(-17.6184,4.61710176889132,-0.807713031086456));
#78266=CARTESIAN_POINT('Ctrl Pts',(-17.6184,4.61286384600412,-0.826412810646483));
#78267=CARTESIAN_POINT('Ctrl Pts',(-17.6184,4.60851138104239,-0.845085572518443));
#78268=CARTESIAN_POINT('Ctrl Pts',(-17.6184,4.60404615614281,-0.863725337721086));
#78269=CARTESIAN_POINT('Ctrl Pts',(-17.6184,4.57140957603825,-0.99996443067781));
#78270=CARTESIAN_POINT('Ctrl Pts',(-17.6184,4.5327344910388,-1.1345251091489));
#78271=CARTESIAN_POINT('Ctrl Pts',(-17.6184,4.48825308683246,-1.26698550606458));
#78272=CARTESIAN_POINT('Ctrl Pts',(-17.6184,4.4435856042334,-1.40000002257693));
#78273=CARTESIAN_POINT('Ctrl Pts',(-17.6184,4.39306276857063,-1.53089744915004));
#78274=CARTESIAN_POINT('Ctrl Pts',(-17.6184,4.33686983674132,-1.65923491503709));
#78275=CARTESIAN_POINT('Ctrl Pts',(-17.6184,4.2828641903748,-1.78257690081076));
#78276=CARTESIAN_POINT('Ctrl Pts',(-17.6184,4.22362068596107,-1.90355486374681));
#78277=CARTESIAN_POINT('Ctrl Pts',(-17.6184,4.15926519043502,-2.02175178363005));
#78278=CARTESIAN_POINT('Ctrl Pts',(-17.6184,4.11365597924993,-2.10551880673066));
#78279=CARTESIAN_POINT('Ctrl Pts',(-17.6184,4.06547835815844,-2.18788846192158));
#78280=CARTESIAN_POINT('Ctrl Pts',(-17.6184,4.01479316151161,-2.26875477322379));
#78281=CARTESIAN_POINT('Ctrl Pts',(-17.6184,3.99105024278133,-2.30663570067969));
#78282=CARTESIAN_POINT('Ctrl Pts',(-17.6184,3.96675696552567,-2.34418662407999));
#78283=CARTESIAN_POINT('Ctrl Pts',(-17.6184,3.94191903989479,-2.38139598871097));
#78284=CARTESIAN_POINT('Ctrl Pts',(-17.6184,3.92720191601446,-2.40344351542156));
#78285=CARTESIAN_POINT('Ctrl Pts',(-17.6184,3.91229356663274,-2.42537111682055));
#78286=CARTESIAN_POINT('Ctrl Pts',(-17.6184,3.89719512685908,-2.4471763135535));
#78287=CARTESIAN_POINT('Ctrl Pts',(-17.6184,3.88793571226168,-2.46054877852041));
#78288=CARTESIAN_POINT('Ctrl Pts',(-17.6184,3.87860551837951,-2.47387411422051));
#78289=CARTESIAN_POINT('Ctrl Pts',(-17.6184,3.86921058723167,-2.48714381222199));
#78290=CARTESIAN_POINT('Ctrl Pts',(-17.6184,3.78526556952311,-2.60571041118819));
#78291=CARTESIAN_POINT('Ctrl Pts',(-17.6184,3.69603451419748,-2.72001500601706));
#78292=CARTESIAN_POINT('Ctrl Pts',(-17.6184,3.6018119705952,-2.82974803590307));
#78293=CARTESIAN_POINT('Ctrl Pts',(-17.6184,3.51211118207048,-2.93421495997094));
#78294=CARTESIAN_POINT('Ctrl Pts',(-17.6184,3.41788563088132,-3.03453885711949));
#78295=CARTESIAN_POINT('Ctrl Pts',(-17.6184,3.31934941853852,-3.13041809444619));
#78296=CARTESIAN_POINT('Ctrl Pts',(-17.6184,3.22168601847118,-3.22544805440257));
#78297=CARTESIAN_POINT('Ctrl Pts',(-17.6184,3.11978748274982,-3.31611220668362));
#78298=CARTESIAN_POINT('Ctrl Pts',(-17.6184,3.01383146888639,-3.40207631807092));
#78299=CARTESIAN_POINT('Ctrl Pts',(-17.6184,2.90999389424987,-3.48632169977948));
#78300=CARTESIAN_POINT('Ctrl Pts',(-17.6184,2.8022589807078,-3.56605343912507));
#78301=CARTESIAN_POINT('Ctrl Pts',(-17.6184,2.69077155688435,-3.6409121095589));
#78302=CARTESIAN_POINT('Ctrl Pts',(-17.6184,2.66910594838121,-3.65545956783772));
#78303=CARTESIAN_POINT('Ctrl Pts',(-17.6184,2.64729856962228,-3.66982284730888));
#78304=CARTESIAN_POINT('Ctrl Pts',(-17.6184,2.62535040627071,-3.68399909158434));
#78305=CARTESIAN_POINT('Origin',(-17.6184,0.,0.));
#78306=CARTESIAN_POINT('Origin',(-19.0048063345371,0.,0.));
#78307=CARTESIAN_POINT('Ctrl Pts',(-17.6184,2.62535040627071,-3.68399909158434));
#78308=CARTESIAN_POINT('Ctrl Pts',(-17.5985223379305,3.23883466326236,-3.24680811968291));
#78309=CARTESIAN_POINT('Ctrl Pts',(-17.5587670137914,4.23254591953354,-2.06184536971571));
#78310=CARTESIAN_POINT('Ctrl Pts',(-17.4792563655133,4.8909587174436,0.989874372427294));
#78311=CARTESIAN_POINT('Ctrl Pts',(-17.3798680551657,2.68243561037911,4.62805141939821));
#78312=CARTESIAN_POINT('Ctrl Pts',(-17.2606020827485,-2.44949610129593,
4.7591308229798));
#78313=CARTESIAN_POINT('Ctrl Pts',(-17.1772481758723,-4.45802737904165,
1.79294945179082));
#78314=CARTESIAN_POINT('Ctrl Pts',(-17.1336495931351,-4.53003253390568,
0.147368644500374));
#78315=CARTESIAN_POINT('Ctrl Pts',(-17.129806334537,-4.52905226269683,0.0022285783852446));
#78316=CARTESIAN_POINT('Ctrl Pts',(-17.8668049533188,2.87504524181639,-4.03438109968666));
#78317=CARTESIAN_POINT('Ctrl Pts',(-17.8469272912493,3.54687746268103,-3.55560926773309));
#78318=CARTESIAN_POINT('Ctrl Pts',(-17.8071719671102,4.63509974807851,-2.25794572236962));
#78319=CARTESIAN_POINT('Ctrl Pts',(-17.7276613188321,5.35613362502683,1.0840204788079));
#78320=CARTESIAN_POINT('Ctrl Pts',(-17.6282730084845,2.93755977094575,5.06822143834209));
#78321=CARTESIAN_POINT('Ctrl Pts',(-17.5090070360674,-2.68246558404474,
5.21176769207864));
#78322=CARTESIAN_POINT('Ctrl Pts',(-17.3897410636502,-5.82968193086184,
0.563986199967765));
#78323=CARTESIAN_POINT('Ctrl Pts',(-17.270475091233,-3.63071138506581,-4.59793593777515));
#78324=CARTESIAN_POINT('Ctrl Pts',(-17.1512091188158,1.90400000504956,-5.54091032617354));
#78325=CARTESIAN_POINT('Ctrl Pts',(-17.0319431463987,5.68939374674768,-1.39643871054889));
#78326=CARTESIAN_POINT('Ctrl Pts',(-16.9126771739815,4.25280175532545,4.02941979983046));
#78327=CARTESIAN_POINT('Ctrl Pts',(-16.7934112015644,-1.08819795636646,
5.75661471108102));
#78328=CARTESIAN_POINT('Ctrl Pts',(-16.6741452291472,-5.43003511364721,
2.19919371409573));
#78329=CARTESIAN_POINT('Ctrl Pts',(-16.55487925673,-4.78730836808999,-3.37697293683734));
#78330=CARTESIAN_POINT('Ctrl Pts',(-16.4356132843129,0.250143793580362,
-5.85317724934502));
#78331=CARTESIAN_POINT('Ctrl Pts',(-16.3163473118957,5.05793681468126,-2.95624591066989));
#78332=CARTESIAN_POINT('Ctrl Pts',(-16.1970813394786,5.2226486393331,2.65445654805712));
#78333=CARTESIAN_POINT('Ctrl Pts',(-16.0778153670614,0.593051366503517,
5.82842001816422));
#78334=CARTESIAN_POINT('Ctrl Pts',(-15.9585493946442,-4.58095211955662,
3.65199249477323));
#78335=CARTESIAN_POINT('Ctrl Pts',(-15.839283422227,-5.54972387549991,-1.87689883035945));
#78336=CARTESIAN_POINT('Ctrl Pts',(-15.7200174498099,-1.42394462969,-5.68283061407078));
#78337=CARTESIAN_POINT('Ctrl Pts',(-15.6007514773927,4.00899028053514,-4.27202255834164));
#78338=CARTESIAN_POINT('Ctrl Pts',(-15.4814855049755,5.76174238590305,1.06042746340526));
#78339=CARTESIAN_POINT('Ctrl Pts',(-15.3622195325584,2.22531528333639,5.41942369241641));
#78340=CARTESIAN_POINT('Ctrl Pts',(-15.2429535601412,-3.35391234047839,
4.80348342455471));
#78341=CARTESIAN_POINT('Ctrl Pts',(-15.1236875877241,-5.85430698164175,
-0.221970816878097));
#78342=CARTESIAN_POINT('Ctrl Pts',(-15.0044216153069,-2.98054988927022,
-5.04365973784862));
#78343=CARTESIAN_POINT('Ctrl Pts',(-14.8851556428897,2.62930000449966,-5.23535697450904));
#78344=CARTESIAN_POINT('Ctrl Pts',(-14.7658896704726,5.82549835830257,-0.621087821490262));
#78345=CARTESIAN_POINT('Ctrl Pts',(-14.6466236980554,3.67399081555006,4.56332912214217));
#78346=CARTESIAN_POINT('Ctrl Pts',(-14.5273577256382,-1.85017621709516,
5.55868951756596));
#78347=CARTESIAN_POINT('Ctrl Pts',(-14.4080917532211,-5.67591375177504,
1.45126988361524));
#78348=CARTESIAN_POINT('Ctrl Pts',(-14.2888257808039,-4.29126145322842,
-3.98839019282699));
#78349=CARTESIAN_POINT('Ctrl Pts',(-14.1695598083868,1.03269401679673,-5.76677763206729));
#78350=CARTESIAN_POINT('Ctrl Pts',(-14.0502938359695,5.40865439039165,-2.25136378138128));
#78351=CARTESIAN_POINT('Ctrl Pts',(-13.9310278635524,4.81956436383399,3.33076275547831));
#78352=CARTESIAN_POINT('Ctrl Pts',(-13.8117618911352,-0.193801692465541,
5.85530717336233));
#78353=CARTESIAN_POINT('Ctrl Pts',(-13.6924959187181,-5.02926117512766,
3.0047817263303));
#78354=CARTESIAN_POINT('Ctrl Pts',(-13.5732299463009,-5.24794661246699,
-2.60408094021077));
#78355=CARTESIAN_POINT('Ctrl Pts',(-13.4539639738837,-0.649108587035416,
-5.8224427204324));
#78356=CARTESIAN_POINT('Ctrl Pts',(-13.3346980014666,4.5455998004388,-3.69590363033771));
#78357=CARTESIAN_POINT('Ctrl Pts',(-13.2154320290494,5.5675268492086,1.82341053354003));
#78358=CARTESIAN_POINT('Ctrl Pts',(-13.0961660566323,1.47856135155213,5.6688656290462));
#78359=CARTESIAN_POINT('Ctrl Pts',(-12.9769000842151,-3.96769767979603,
4.31040094564622));
#78360=CARTESIAN_POINT('Ctrl Pts',(-12.8576341117979,-5.77167944021737,
-1.00493662977195));
#78361=CARTESIAN_POINT('Ctrl Pts',(-12.7383681393807,-2.27736013621432,
-5.39775990578199));
#78362=CARTESIAN_POINT('Ctrl Pts',(-12.6191021669636,3.30753605425009,-4.83553372858896));
#78363=CARTESIAN_POINT('Ctrl Pts',(-12.4998361945464,5.85617183240789,0.165628076719709));
#78364=CARTESIAN_POINT('Ctrl Pts',(-12.3805702221293,3.02894400371043,5.01474619625683));
#78365=CARTESIAN_POINT('Ctrl Pts',(-12.2613042497121,-2.57880159371761,
5.26041476793657));
#78366=CARTESIAN_POINT('Ctrl Pts',(-12.1420382772949,-5.81925230402365,
0.677114327570302));
#78367=CARTESIAN_POINT('Ctrl Pts',(-12.0227723048778,-3.71773089063149,
-4.52776525620864));
#78368=CARTESIAN_POINT('Ctrl Pts',(-11.9035063324606,1.79660264081118,-5.57623530184263));
#78369=CARTESIAN_POINT('Ctrl Pts',(-11.7842403600434,5.66168628186157,-1.50581859341225));
#78370=CARTESIAN_POINT('Ctrl Pts',(-11.6649743876263,4.32944065950869,3.94691332135362));
#78371=CARTESIAN_POINT('Ctrl Pts',(-11.5457084152091,-0.977155980123466,
5.77644764375084));
#78372=CARTESIAN_POINT('Ctrl Pts',(-11.426442442792,-5.38674047221298,2.30330377404027));
#78373=CARTESIAN_POINT('Ctrl Pts',(-11.3071764703748,-4.85139115892997,
-3.28423278918257));
#78374=CARTESIAN_POINT('Ctrl Pts',(-11.1879104979576,0.137450626958296,
-5.85690093100732));
#78375=CARTESIAN_POINT('Ctrl Pts',(-11.0686445255404,5.00011513452361,-3.05303616617843));
#78376=CARTESIAN_POINT('Ctrl Pts',(-10.9493785531233,5.27276115372783,2.55346255234429));
#78377=CARTESIAN_POINT('Ctrl Pts',(-10.8301125807061,0.705104394058296,
5.81592718179702));
#78378=CARTESIAN_POINT('Ctrl Pts',(-10.710846608289,-4.5098259018956,3.73947209176336));
#78379=CARTESIAN_POINT('Ctrl Pts',(-10.5915806358718,-5.58481467409041,
-1.7697531597797));
#78380=CARTESIAN_POINT('Ctrl Pts',(-10.4723146634546,-1.53304097812696,
-5.65437587624569));
#78381=CARTESIAN_POINT('Ctrl Pts',(-10.3530486910375,3.92603759856465,-4.34838015416571));
#78382=CARTESIAN_POINT('Ctrl Pts',(-10.2337827186203,5.78108213232227,0.949352710972031));
#78383=CARTESIAN_POINT('Ctrl Pts',(-10.1145167462031,2.32919409429188,5.37559634474182));
#78384=CARTESIAN_POINT('Ctrl Pts',(-9.99525077378599,-3.26085349969837,
4.867136287797));
#78385=CARTESIAN_POINT('Ctrl Pts',(-9.8759848013688,-5.85749445228765,-0.109269995448056));
#78386=CARTESIAN_POINT('Ctrl Pts',(-9.75671882895166,-3.07705765603928,
-4.98536832860881));
#78387=CARTESIAN_POINT('Ctrl Pts',(-9.63745285653448,2.52806440264535,-5.28498548404467));
#78388=CARTESIAN_POINT('Ctrl Pts',(-9.51818688411733,5.81246743072405,-0.733078138575955));
#78389=CARTESIAN_POINT('Ctrl Pts',(-9.39892091170016,3.76112673046111,4.49178215276483));
#78390=CARTESIAN_POINT('Ctrl Pts',(-9.27965493928299,-1.74286271196533,
5.59326476735425));
#78391=CARTESIAN_POINT('Ctrl Pts',(-9.16038896686583,-5.64693458142209,
1.56022787554418));
#78392=CARTESIAN_POINT('Ctrl Pts',(-9.04112299444866,-4.36721899120011,
-3.90507099466665));
#78393=CARTESIAN_POINT('Ctrl Pts',(-8.9218570220315,0.921527465916119,-5.78558279865112));
#78394=CARTESIAN_POINT('Ctrl Pts',(-8.80259104961434,5.36432778133606,-2.35503049765218));
#78395=CARTESIAN_POINT('Ctrl Pts',(-8.68332507719717,4.88276875071711,3.23739872698841));
#78396=CARTESIAN_POINT('Ctrl Pts',(-8.56405910477999,-0.0810868345228415,
5.85795238250983));
#78397=CARTESIAN_POINT('Ctrl Pts',(-8.44479313236285,-4.97050611987588,
3.10100791723629));
#78398=CARTESIAN_POINT('Ctrl Pts',(-8.32552715994566,-5.29708747591468,
-2.5026077325449));
#78399=CARTESIAN_POINT('Ctrl Pts',(-8.20626118752852,-0.761034913578503,
-5.80887313089209));
#78400=CARTESIAN_POINT('Ctrl Pts',(-8.08699521511134,4.47363442649844,-3.7826943054566));
#78401=CARTESIAN_POINT('Ctrl Pts',(-7.96772924269418,5.60158538602889,1.71593191983633));
#78402=CARTESIAN_POINT('Ctrl Pts',(-7.84846327027702,1.5873786563333,5.63936256964411));
#78403=CARTESIAN_POINT('Ctrl Pts',(-7.72919729785985,-3.88401399500086,
4.38595673452477));
#78404=CARTESIAN_POINT('Ctrl Pts',(-7.6099313254427,-5.78994953855466,-0.893680889062952));
#78405=CARTESIAN_POINT('Ctrl Pts',(-7.49066535302551,-2.38081238605224,
-5.35293504284386));
#78406=CARTESIAN_POINT('Ctrl Pts',(-7.37139938060837,3.21386901399082,-4.89828818582527));
#78407=CARTESIAN_POINT('Ctrl Pts',(-7.25213340819118,5.85827471107363,0.0529017965749914));
#78408=CARTESIAN_POINT('Ctrl Pts',(-7.13286743577404,3.1248863953615,4.95552885235978));
#78409=CARTESIAN_POINT('Ctrl Pts',(-7.01360146335686,-2.47709313132159,
5.30906684919723));
#78410=CARTESIAN_POINT('Ctrl Pts',(-6.8943354909397,-5.80514436550315,0.788974071914089));
#78411=CARTESIAN_POINT('Ctrl Pts',(-6.77506951852254,-3.80417431749705,
-4.45538314318551));
#78412=CARTESIAN_POINT('Ctrl Pts',(-6.65580354610538,1.68896140679477,-5.6097763375061));
#78413=CARTESIAN_POINT('Ctrl Pts',(-6.5365375736882,5.63166001619102,-1.6144926919999));
#78414=CARTESIAN_POINT('Ctrl Pts',(-6.41727160127105,4.40459295039272,3.86286708700112));
#78415=CARTESIAN_POINT('Ctrl Pts',(-6.29800562885387,-0.865813625013472,
5.79418225095022));
#78416=CARTESIAN_POINT('Ctrl Pts',(-6.17873965643672,-5.3414183929878,2.40653916268516));
#78417=CARTESIAN_POINT('Ctrl Pts',(-6.05947368401955,-4.9136942338729,-3.19026490537854));
#78418=CARTESIAN_POINT('Ctrl Pts',(-5.94020771160238,0.0247155340402711,
-5.85846143051762));
#78419=CARTESIAN_POINT('Ctrl Pts',(-5.82094173918523,4.94043687275883,-3.14869253766872));
#78420=CARTESIAN_POINT('Ctrl Pts',(-5.70167576676805,5.32092332659016,2.45152118959525));
#78421=CARTESIAN_POINT('Ctrl Pts',(-5.58240979435089,0.816894966838531,
5.80128122087176));
#78422=CARTESIAN_POINT('Ctrl Pts',(-5.46314382193373,-4.43702872531231,
3.82556626935662));
#78423=CARTESIAN_POINT('Ctrl Pts',(-5.34387784951656,-5.61783743217928,
-1.66195179716236));
#78424=CARTESIAN_POINT('Ctrl Pts',(-5.2246118770994,-1.64156935489994,-5.62382709936382));
#78425=CARTESIAN_POINT('Ctrl Pts',(-5.10534590468224,3.84163076018247,-4.42312720740718));
#78426=CARTESIAN_POINT('Ctrl Pts',(-4.98607993226507,5.79828083785774,0.837926318847652));
#78427=CARTESIAN_POINT('Ctrl Pts',(-4.8668139598479,2.4322102320196,5.32977809835875));
#78428=CARTESIAN_POINT('Ctrl Pts',(-4.74754798743074,-3.16658694754665,
4.92898653823612));
#78429=CARTESIAN_POINT('Ctrl Pts',(-4.62828201501358,-5.85851253651964,
0.00347130061708939));
#78430=CARTESIAN_POINT('Ctrl Pts',(-4.50901604259641,-3.17242579308605,
-4.92523053042676));
#78431=CARTESIAN_POINT('Ctrl Pts',(-4.38975007017924,2.42589249931285,-5.33265663363612));
#78432=CARTESIAN_POINT('Ctrl Pts',(-4.27048409776208,5.79728378642323,-0.844796952030536));
#78433=CARTESIAN_POINT('Ctrl Pts',(-4.15121812534491,3.84686966584789,4.41857159775248));
#78434=CARTESIAN_POINT('Ctrl Pts',(-4.03195215292775,-1.63490371616564,
5.62576848344769));
#78435=CARTESIAN_POINT('Ctrl Pts',(-3.91268618051059,-5.61586400048129,
1.66860801825474));
#78436=CARTESIAN_POINT('Ctrl Pts',(-3.79342020809342,-4.44155907653154,
-3.82030550612983));
#78437=CARTESIAN_POINT('Ctrl Pts',(-3.67415423567626,0.810019616109184,
-5.80224520440182));
#78438=CARTESIAN_POINT('Ctrl Pts',(-3.55488826325909,5.31801442840983,-2.457824999814));
#78439=CARTESIAN_POINT('Ctrl Pts',(-3.43562229084193,4.94416474492404,3.14283568859967));
#78440=CARTESIAN_POINT('Ctrl Pts',(-3.31635631842476,0.0316580549198027,
5.85842802789658));
#78441=CARTESIAN_POINT('Ctrl Pts',(-3.1970903460076,-4.90991017736459,3.19608561222904));
#78442=CARTESIAN_POINT('Ctrl Pts',(-3.07782437359043,-5.34426649872899,
-2.4002076537351));
#78443=CARTESIAN_POINT('Ctrl Pts',(-2.95855840117328,-0.872679381606534,
-5.79315215469129));
#78444=CARTESIAN_POINT('Ctrl Pts',(-2.8392924287561,4.40001218775717,-3.8680840138335));
#78445=CARTESIAN_POINT('Ctrl Pts',(-2.72002645633894,5.63356930772102,1.60781778992187));
#78446=CARTESIAN_POINT('Ctrl Pts',(-2.60076048392178,1.69560805616505,5.6077709038756));
#78447=CARTESIAN_POINT('Ctrl Pts',(-2.48149451150461,-3.79889181848672,
4.45988813109932));
#78448=CARTESIAN_POINT('Ctrl Pts',(-2.36222853908745,-5.80607525881414,
-0.782094162791051));
#78449=CARTESIAN_POINT('Ctrl Pts',(-2.24296256667028,-2.48338287312981,
-5.30612765544998));
#78450=CARTESIAN_POINT('Ctrl Pts',(-2.12369659425312,3.11901167833903,-4.95922850258693));
#78451=CARTESIAN_POINT('Ctrl Pts',(-2.00443062183595,5.85820790660474,-0.0598440763921811));
#78452=CARTESIAN_POINT('Ctrl Pts',(-1.88516464941879,3.21967144741286,4.89447616821248));
#78453=CARTESIAN_POINT('Ctrl Pts',(-1.76589867700162,-2.37446724742266,
5.35575265312009));
#78454=CARTESIAN_POINT('Ctrl Pts',(-1.64663270458446,-5.78888642131629,
0.900541610135457));
#78455=CARTESIAN_POINT('Ctrl Pts',(-1.5273667321673,-3.88920882223712,-4.38135092494524));
#78456=CARTESIAN_POINT('Ctrl Pts',(-1.40810075975013,1.58069464542428,-5.64123972442342));
#78457=CARTESIAN_POINT('Ctrl Pts',(-1.28883478733297,5.59954799688826,-1.72256884362577));
#78458=CARTESIAN_POINT('Ctrl Pts',(-1.1695688149158,4.47811394682395,3.77739019294359));
#78459=CARTESIAN_POINT('Ctrl Pts',(-1.05030284249864,-0.754150605320021,
5.80977091243547));
#78460=CARTESIAN_POINT('Ctrl Pts',(-0.931036870081473,-5.29411805463789,
2.50888326034566));
#78461=CARTESIAN_POINT('Ctrl Pts',(-0.81177089766431,-4.97417746252431,
-3.09511546825006));
#78462=CARTESIAN_POINT('Ctrl Pts',(-0.692504925247144,-0.0880287125757489,
-5.85785217773957));
#78463=CARTESIAN_POINT('Ctrl Pts',(-0.573238952829979,4.87892886024161,
-3.24318275266551));
#78464=CARTESIAN_POINT('Ctrl Pts',(-0.453972980412814,5.36711483092438,
2.3486718762222));
#78465=CARTESIAN_POINT('Ctrl Pts',(-0.334707007995651,0.92838299265408,
5.78448668504272));
#78466=CARTESIAN_POINT('Ctrl Pts',(-0.215441035578486,-4.36258824129331,
3.91024360205536));
#78467=CARTESIAN_POINT('Ctrl Pts',(-0.0961750631613217,-5.6487795559977,
-1.55353491052762));
#78468=CARTESIAN_POINT('Ctrl Pts',(0.0230909092558439,-1.74948975654047,
-5.59119546986562));
#78469=CARTESIAN_POINT('Ctrl Pts',(0.142356881673008,3.75580112722664,-4.49623610180878));
#78470=CARTESIAN_POINT('Ctrl Pts',(0.261622854090171,5.81333207971762,0.726189590542047));
#78471=CARTESIAN_POINT('Ctrl Pts',(0.380888826507337,2.53432557117091,5.28198590397543));
#78472=CARTESIAN_POINT('Ctrl Pts',(0.500154798924501,-3.07114761148953,
4.98901127869317));
#78473=CARTESIAN_POINT('Ctrl Pts',(0.619420771341668,-5.85736084953548,
0.116211311043978));
#78474=CARTESIAN_POINT('Ctrl Pts',(0.738686743758829,-3.2666189837402,-4.86326861334576));
#78475=CARTESIAN_POINT('Ctrl Pts',(0.857952716175997,2.32282213725285,-5.37835276912677));
#78476=CARTESIAN_POINT('Ctrl Pts',(0.977218688593157,5.77995304771692,-0.956202884681618));
#78477=CARTESIAN_POINT('Ctrl Pts',(1.09648466101033,3.93118786636879,4.34372457112565));
#78478=CARTESIAN_POINT('Ctrl Pts',(1.21575063342749,-1.52633921393369,5.65618862790959));
#78479=CARTESIAN_POINT('Ctrl Pts',(1.33501660584466,-5.58271351615443,1.77637017173568));
#78480=CARTESIAN_POINT('Ctrl Pts',(1.45428257826181,-4.51425417655669,-3.73412512108611));
#78481=CARTESIAN_POINT('Ctrl Pts',(1.57354855067899,0.698211765707205,-5.81675867822566));
#78482=CARTESIAN_POINT('Ctrl Pts',(1.69281452309614,5.26973148430123,-2.55970921665918));
#78483=CARTESIAN_POINT('Ctrl Pts',(1.81208049551331,5.00372960771586,3.04710866287265));
#78484=CARTESIAN_POINT('Ctrl Pts',(1.93134646793048,0.144391219417513,5.85673393336599));
#78485=CARTESIAN_POINT('Ctrl Pts',(2.05061244034764,-4.84749579003301,3.28997959812789));
#78486=CARTESIAN_POINT('Ctrl Pts',(2.16987841276481,-5.38946620758809,-2.29691862889217));
#78487=CARTESIAN_POINT('Ctrl Pts',(2.28914438518197,-0.98400064223475,-5.77528561428499));
#78488=CARTESIAN_POINT('Ctrl Pts',(2.40841035759913,4.32476035110414,-3.95204113035316));
#78489=CARTESIAN_POINT('Ctrl Pts',(2.5276763300163,5.6634667686517,1.49910818517671));
#78490=CARTESIAN_POINT('Ctrl Pts',(2.64694230243346,1.80320946697538,5.5741023320976));
#78491=CARTESIAN_POINT('Ctrl Pts',(2.76620827485063,-3.71236267628471,4.53216775397974));
#78492=CARTESIAN_POINT('Ctrl Pts',(2.88547424726779,-5.82005062863969,-0.670217778454638));
#78493=CARTESIAN_POINT('Ctrl Pts',(3.00474021968496,-2.58503360922216,-5.25735507928439));
#78494=CARTESIAN_POINT('Ctrl Pts',(3.12400619210212,3.02299917886025,-5.01833210888796));
#78495=CARTESIAN_POINT('Ctrl Pts',(3.24327216451929,5.85597144374314,-0.172567785379327));
#78496=CARTESIAN_POINT('Ctrl Pts',(3.36253813693645,3.31326405507003,4.83161075541754));
#78497=CARTESIAN_POINT('Ctrl Pts',(3.48180410935361,-2.27096195076241,5.40045488905101));
#78498=CARTESIAN_POINT('Ctrl Pts',(3.60107008177078,-5.77048449279005,1.01177562184265));
#78499=CARTESIAN_POINT('Ctrl Pts',(3.72033605418794,-3.97280291129088,-4.30569602021837));
#78500=CARTESIAN_POINT('Ctrl Pts',(3.83960202660511,1.47184245460874,-5.67061380974733));
#78501=CARTESIAN_POINT('Ctrl Pts',(3.95886799902227,5.56536211702939,-1.83000702097551));
#78502=CARTESIAN_POINT('Ctrl Pts',(4.07813397143944,4.54997641940911,3.69051429658614));
#78503=CARTESIAN_POINT('Ctrl Pts',(4.1973999438566,-0.642208276797606,5.82320785475656));
#78504=CARTESIAN_POINT('Ctrl Pts',(4.31666591627376,-5.24485697541764,2.61029816264319));
#78505=CARTESIAN_POINT('Ctrl Pts',(4.43593188869093,-5.03281844418643,-2.99881971754596));
#78506=CARTESIAN_POINT('Ctrl Pts',(4.55519786110809,-0.200740356689758,
-5.85507339831722));
#78507=CARTESIAN_POINT('Ctrl Pts',(4.67446383352526,4.81561387721088,-3.33647181557097));
#78508=CARTESIAN_POINT('Ctrl Pts',(4.79372980594242,5.41131855914629,2.24495270371661));
#78509=CARTESIAN_POINT('Ctrl Pts',(4.91299577835959,1.03952718056155,5.76554979436997));
#78510=CARTESIAN_POINT('Ctrl Pts',(5.03226175077675,-4.28653201977527,3.99347272858184));
#78511=CARTESIAN_POINT('Ctrl Pts',(5.15152772319392,-5.67762958575462,-1.44454265338526));
#78512=CARTESIAN_POINT('Ctrl Pts',(5.27079369561108,-1.85676221341805,-5.55649307327102));
#78513=CARTESIAN_POINT('Ctrl Pts',(5.39005966802825,3.66858048774337,-4.56767976060429));
#78514=CARTESIAN_POINT('Ctrl Pts',(5.50932564044541,5.82623028349186,0.614183909108646));
#78515=CARTESIAN_POINT('Ctrl Pts',(5.62859161286257,2.63550229209064,5.23223746201096));
#78516=CARTESIAN_POINT('Ctrl Pts',(5.74785758527974,-2.9745708386434,5.0471882782771));
#78517=CARTESIAN_POINT('Ctrl Pts',(5.8671235576969,-5.85403981787645,0.228908281201479));
#78518=CARTESIAN_POINT('Ctrl Pts',(5.98638953011408,-3.3596023424104,-4.79950552571371));
#78519=CARTESIAN_POINT('Ctrl Pts',(6.10565550253123,2.21889148982482,-5.42205696639832));
#78520=CARTESIAN_POINT('Ctrl Pts',(6.2249214749484,5.76048163325456,-1.06725467598998));
#78521=CARTESIAN_POINT('Ctrl Pts',(6.34418744736557,4.01405010375492,4.26726879338893));
#78522=CARTESIAN_POINT('Ctrl Pts',(6.46345341978272,-1.41720941345036,5.6845139342703));
#78523=CARTESIAN_POINT('Ctrl Pts',(6.5827193921999,-5.54749540612569,1.88347442496573));
#78524=CARTESIAN_POINT('Ctrl Pts',(6.70198536461705,-4.58527736776309,-3.64656175748683));
#78525=CARTESIAN_POINT('Ctrl Pts',(6.82125133703423,0.586145324104315,-5.82911784488152));
#78526=CARTESIAN_POINT('Ctrl Pts',(6.94051730945138,5.21949683118455,-2.66064541413169));
#78527=CARTESIAN_POINT('Ctrl Pts',(7.05978328186856,5.06144127852277,2.95025310347291));
#78528=CARTESIAN_POINT('Ctrl Pts',(7.17904925428571,0.257070906874864,5.85287072634652));
#78529=CARTESIAN_POINT('Ctrl Pts',(7.29831522670289,-4.78328607380694,3.38265510015582));
#78530=CARTESIAN_POINT('Ctrl Pts',(7.41758119912004,-5.43266986223127,-2.19277891235983));
#78531=CARTESIAN_POINT('Ctrl Pts',(7.53684717153722,-1.09495746628347,-5.75528012676322));
#78532=CARTESIAN_POINT('Ctrl Pts',(7.65611314395437,4.24790678697028,-4.03453456047874));
#78533=CARTESIAN_POINT('Ctrl Pts',(7.77537911637154,5.6912666959334,1.38984336752211));
#78534=CARTESIAN_POINT('Ctrl Pts',(7.8946450887887,1.91014303727615,5.53836932387422));
#78535=CARTESIAN_POINT('Ctrl Pts',(8.01391106120587,-3.62445861551272,4.60276883353065));
#78536=CARTESIAN_POINT('Ctrl Pts',(8.13317703362303,-5.83187047208342,-0.558093170830226));
#78537=CARTESIAN_POINT('Ctrl Pts',(8.25244300604019,-2.68572694674573,-5.20663537786251));
#78538=CARTESIAN_POINT('Ctrl Pts',(8.37170897845736,2.92586707494877,-5.0755771149906));
#78539=CARTESIAN_POINT('Ctrl Pts',(8.49097495087453,5.85156615078993,-0.285227581792945));
#78540=CARTESIAN_POINT('Ctrl Pts',(8.61024092329168,3.40562955517506,4.76695589694342));
#78541=CARTESIAN_POINT('Ctrl Pts',(8.72950689570887,-2.16661557578352,5.44315700097451));
#78542=CARTESIAN_POINT('Ctrl Pts',(8.84877286812601,-5.749945395302,1.12263491016946));
#78543=CARTESIAN_POINT('Ctrl Pts',(8.96803884054319,-4.05492562457292,-4.22844644871701));
#78544=CARTESIAN_POINT('Ctrl Pts',(9.08730481296034,1.36244514907805,-5.69788771442885));
#78545=CARTESIAN_POINT('Ctrl Pts',(9.20657078537752,5.52911503776992,-1.93676743301625));
#78546=CARTESIAN_POINT('Ctrl Pts',(9.32583675779466,4.6201537530093,3.60227157347134));
#78547=CARTESIAN_POINT('Ctrl Pts',(9.44510273021186,-0.530028098646155,
5.83448810137882));
#78548=CARTESIAN_POINT('Ctrl Pts',(9.564368702629,-5.19365339976557,2.71074630933791));
#78549=CARTESIAN_POINT('Ctrl Pts',(9.68363467504617,-5.08959546046003,-2.90141331756615));
#78550=CARTESIAN_POINT('Ctrl Pts',(9.80290064746334,-0.313377654176505,
-5.85012612140531));
#78551=CARTESIAN_POINT('Ctrl Pts',(9.92216661988049,4.75051537313899,-3.4285251756485));
#78552=CARTESIAN_POINT('Ctrl Pts',(10.0414325922977,5.45351813986867,2.14040208573271));
#78553=CARTESIAN_POINT('Ctrl Pts',(10.1606985647148,1.1502863669621,5.74447756236082));
#78554=CARTESIAN_POINT('Ctrl Pts',(10.279964537132,-4.20888822910284,4.07522282401896));
#78555=CARTESIAN_POINT('Ctrl Pts',(10.3992305095492,-5.70437683649141,-1.33501539234042));
#78556=CARTESIAN_POINT('Ctrl Pts',(10.5184964819663,-1.96334699587643,-5.51973276203376));
#78557=CARTESIAN_POINT('Ctrl Pts',(10.6377624543835,3.58000114495498,-4.63743172376764));
#78558=CARTESIAN_POINT('Ctrl Pts',(10.7570284268007,5.83697067217415,0.50195075721085));
#78559=CARTESIAN_POINT('Ctrl Pts',(10.8762943992178,2.73570292275234,5.18055119740459));
#78560=CARTESIAN_POINT('Ctrl Pts',(10.995560371635,-2.87689239738814,5.10349599043008));
#78561=CARTESIAN_POINT('Ctrl Pts',(11.1148263440521,-5.84855067152691,0.341520472399031));
#78562=CARTESIAN_POINT('Ctrl Pts',(11.2340923164693,-3.45134143158132,-4.73396488296396));
#78563=CARTESIAN_POINT('Ctrl Pts',(11.3533582888865,2.11413904900531,-5.4637530390709));
#78564=CARTESIAN_POINT('Ctrl Pts',(11.4726242613036,5.73887675451073,-1.17791119657705));
#78565=CARTESIAN_POINT('Ctrl Pts',(11.5918902337208,4.09542568897112,4.18923258086744));
#78566=CARTESIAN_POINT('Ctrl Pts',(11.711156206138,-1.30755473226162,5.71073391190888));
#78567=CARTESIAN_POINT('Ctrl Pts',(11.8304221785551,-5.51022271384947,1.98988111058489));
#78568=CARTESIAN_POINT('Ctrl Pts',(11.9496881509723,-4.65460234584999,-3.55764784548636));
#78569=CARTESIAN_POINT('Ctrl Pts',(12.0689541233895,0.473861796467209,-5.83931812700205));
#78570=CARTESIAN_POINT('Ctrl Pts',(12.1882200958066,5.16732907407318,-2.76059620928582));
#78571=CARTESIAN_POINT('Ctrl Pts',(12.3074860682238,5.11727838312716,2.85230488203232));
#78572=CARTESIAN_POINT('Ctrl Pts',(12.426752040641,0.369655385002119,5.84683983762381));
#78573=CARTESIAN_POINT('Ctrl Pts',(12.5460180130581,-4.71730480953397,3.47407779481591));
#78574=CARTESIAN_POINT('Ctrl Pts',(12.6652839854753,-5.47386146166072,-2.08782707354593));
#78575=CARTESIAN_POINT('Ctrl Pts',(12.7845499578925,-1.20550875954632,-5.7331431014011));
#78576=CARTESIAN_POINT('Ctrl Pts',(12.9038159303096,4.1694799590057,-4.1155337517672));
#78577=CARTESIAN_POINT('Ctrl Pts',(13.0230819027268,5.71695879352572,1.28006380450929));
#78578=CARTESIAN_POINT('Ctrl Pts',(13.1423478751439,2.01636916292184,5.50058511335874));
#78579=CARTESIAN_POINT('Ctrl Pts',(13.2616138475611,-3.5352121925064,4.6716652217854));
#78580=CARTESIAN_POINT('Ctrl Pts',(13.3808798199783,-5.84153041152292,-0.445761866626982));
#78581=CARTESIAN_POINT('Ctrl Pts',(13.5001457923954,-2.78542559270095,-5.15398733584129));
#78582=CARTESIAN_POINT('Ctrl Pts',(13.6194117648126,2.82765134065804,-5.13094231951208));
#78583=CARTESIAN_POINT('Ctrl Pts',(13.7386777372298,5.84499365929882,-0.397781740710223));
#78584=CARTESIAN_POINT('Ctrl Pts',(13.8579437096469,3.49673373904406,4.70053553850163));
#78585=CARTESIAN_POINT('Ctrl Pts',(13.9772096820641,-2.06146676843229,5.48384317364516));
#78586=CARTESIAN_POINT('Ctrl Pts',(14.0964756544813,-5.72727673575607,1.23307841703323));
#78587=CARTESIAN_POINT('Ctrl Pts',(14.2157416268984,-4.13554654693988,-4.14963082075738));
#78588=CARTESIAN_POINT('Ctrl Pts',(14.3350075993156,1.25254324545183,-5.72305133724644));
#78589=CARTESIAN_POINT('Ctrl Pts',(14.4542735717327,5.49082018365544,-2.04281053973388));
#78590=CARTESIAN_POINT('Ctrl Pts',(14.5735395441499,4.68861995659749,3.51269470536248));
#78591=CARTESIAN_POINT('Ctrl Pts',(14.6928055165671,-0.417651618155915,
5.84360747452608));
#78592=CARTESIAN_POINT('Ctrl Pts',(14.8120714889842,-5.14052629154732,2.81019049823969));
#78593=CARTESIAN_POINT('Ctrl Pts',(14.9313374614014,-5.14448748328812,-2.80293234395298));
#78594=CARTESIAN_POINT('Ctrl Pts',(15.0506034338186,-0.425898888445909,
-5.84301217928782));
#78595=CARTESIAN_POINT('Ctrl Pts',(15.1698694062357,4.68365745804696,-3.51930873981908));
#78596=CARTESIAN_POINT('Ctrl Pts',(15.2891353786529,5.4936979439647,2.03505874386071));
#78597=CARTESIAN_POINT('Ctrl Pts',(15.4084013510701,1.26061953084691,5.72127779337208));
#78598=CARTESIAN_POINT('Ctrl Pts',(15.5276673234872,-4.1296856255962,4.1554636112268));
#78599=CARTESIAN_POINT('Ctrl Pts',(15.6469332959044,-5.72901140203915,-1.22499369214346));
#78600=CARTESIAN_POINT('Ctrl Pts',(15.7661992683216,-2.06920462894793,-5.48092815078119));
#78601=CARTESIAN_POINT('Ctrl Pts',(15.8854652407387,3.49009590529609,-4.70546615781277));
#78602=CARTESIAN_POINT('Ctrl Pts',(16.0047312131559,5.8455492679312,0.389531701758518));
#78603=CARTESIAN_POINT('Ctrl Pts',(16.1239971855731,2.8348903526364,5.12694625279165));
#78604=CARTESIAN_POINT('Ctrl Pts',(16.2432631579902,-2.77814846411986,5.15791356090758));
#78605=CARTESIAN_POINT('Ctrl Pts',(16.3625291304074,-5.84089544345886,0.454006177344968));
#78606=CARTESIAN_POINT('Ctrl Pts',(16.4817951028245,-3.54180227456795,-4.66667095886892));
#78607=CARTESIAN_POINT('Ctrl Pts',(16.6010610752417,2.00860361113205,-5.50342554449801));
#78608=CARTESIAN_POINT('Ctrl Pts',(16.7203270476589,5.71514641311463,-1.28813146345738));
#78609=CARTESIAN_POINT('Ctrl Pts',(16.839593020076,4.17528448358166,4.10964483521964));
#78610=CARTESIAN_POINT('Ctrl Pts',(16.9588589924932,-1.19741578230951,5.73483884993833));
#78611=CARTESIAN_POINT('Ctrl Pts',(17.0781249649104,-5.47090924371988,2.09555081958569));
#78612=CARTESIAN_POINT('Ctrl Pts',(17.1973909373275,-4.72220343547024,-3.46741631543117));
#78613=CARTESIAN_POINT('Ctrl Pts',(17.3166569097447,0.361402768363106,-5.84735574678891));
#78614=CARTESIAN_POINT('Ctrl Pts',(17.4359228821619,5.11324753392925,-2.85952458413149));
#78615=CARTESIAN_POINT('Ctrl Pts',(17.555188854579,5.17122024157952,2.75330027486351));
#78616=CARTESIAN_POINT('Ctrl Pts',(17.6744548269962,0.482102956771366,5.83864350081062));
#78617=CARTESIAN_POINT('Ctrl Pts',(17.7937207994134,-4.64957643417624,3.56421382260364));
#78618=CARTESIAN_POINT('Ctrl Pts',(17.9129867718305,-5.5130257500676,-1.98210198263782));
#78619=CARTESIAN_POINT('Ctrl Pts',(18.0322527442477,-1.31561357801008,-5.70888273691459));
#78620=CARTESIAN_POINT('Ctrl Pts',(18.1515187166649,4.08950891353811,-4.19500870518504));
#78621=CARTESIAN_POINT('Ctrl Pts',(18.270784689082,5.74053354604842,1.1698101543319));
#78622=CARTESIAN_POINT('Ctrl Pts',(18.3900506614992,2.12184850177754,5.46076369439205));
#78623=CARTESIAN_POINT('Ctrl Pts',(18.5093166339163,-3.4446564607618,4.73883140213048));
#78624=CARTESIAN_POINT('Ctrl Pts',(18.6285826063335,-5.84902686928229,-0.333265469106851));
#78625=CARTESIAN_POINT('Ctrl Pts',(18.7478485787507,-2.88409262248423,-5.09943045206206));
#78626=CARTESIAN_POINT('Ctrl Pts',(18.8671145511678,2.72838835137739,-5.18440721727702));
#78627=CARTESIAN_POINT('Ctrl Pts',(18.986380523585,5.83625640347177,-0.510188576332255));
#78628=CARTESIAN_POINT('Ctrl Pts',(19.1056464960022,3.58654286513676,4.63237427967802));
#78629=CARTESIAN_POINT('Ctrl Pts',(19.2249124684194,-1.95555447184578,5.52249833844519));
#78630=CARTESIAN_POINT('Ctrl Pts',(19.3441784408365,-5.70248690976545,1.3430652383406));
#78631=CARTESIAN_POINT('Ctrl Pts',(19.4634444132536,-4.21463581945459,-4.06927832666386));
#78632=CARTESIAN_POINT('Ctrl Pts',(19.5827103856708,1.14217744723407,-5.74609535854703));
#78633=CARTESIAN_POINT('Ctrl Pts',(19.701976358088,5.45049173764998,-2.14809706677667));
#78634=CARTESIAN_POINT('Ctrl Pts',(19.8212423305052,4.75534967288414,3.42181686813988));
#78635=CARTESIAN_POINT('Ctrl Pts',(19.9405083029223,-0.305120455320437,
5.85056259672785));
#78636=CARTESIAN_POINT('Ctrl Pts',(20.0597742753395,-5.08549532703213,2.90859389898618));
#78637=CARTESIAN_POINT('Ctrl Pts',(20.1790402477566,-5.19747418274383,-2.70341327033015));
#78638=CARTESIAN_POINT('Ctrl Pts',(20.2983062201738,-0.538262385893262,
-5.83373420669972));
#78639=CARTESIAN_POINT('Ctrl Pts',(20.417572192591,4.615064893575,-3.60878888528781));
#78640=CARTESIAN_POINT('Ctrl Pts',(20.5368381650081,5.53184309035626,1.92896169328567));
#78641=CARTESIAN_POINT('Ctrl Pts',(20.6561041374253,1.37048580898969,5.69595907971992));
#78642=CARTESIAN_POINT('Ctrl Pts',(20.7753701098424,-4.04895354290072,4.23416537205587));
#78643=CARTESIAN_POINT('Ctrl Pts',(20.8946360822597,-5.7515241586875,-1.11451830066622));
#78644=CARTESIAN_POINT('Ctrl Pts',(21.0139020546768,-2.17429590697344,-5.44009361127219));
#78645=CARTESIAN_POINT('Ctrl Pts',(21.133168027094,3.39889806626329,-4.77175786536124));
#78646=CARTESIAN_POINT('Ctrl Pts',(21.2524339995111,5.85196289357594,0.276968378513138));
#78647=CARTESIAN_POINT('Ctrl Pts',(21.3716999719283,2.93302784647445,5.07144248141408));
#78648=CARTESIAN_POINT('Ctrl Pts',(21.4909659443455,-2.67837560985263,5.21042083550184));
#78649=CARTESIAN_POINT('Ctrl Pts',(21.6102319167626,-5.83107696887886,0.566323735593342));
#78650=CARTESIAN_POINT('Ctrl Pts',(21.7294978891798,-3.63095136809929,-4.5976486765502));
#78651=CARTESIAN_POINT('Ctrl Pts',(21.848763861597,1.90232426253526,-5.54105978948566));
#78652=CARTESIAN_POINT('Ctrl Pts',(21.9680298340141,5.68929939788601,-1.39787465521763));
#78653=CARTESIAN_POINT('Ctrl Pts',(22.0872958064313,4.253596910913,4.02853503273303));
#78654=CARTESIAN_POINT('Ctrl Pts',(22.2065617788484,-1.08683335489076,5.75681982080229));
#78655=CARTESIAN_POINT('Ctrl Pts',(22.3258277512656,-5.42956955595747,2.20044441590912));
#78656=CARTESIAN_POINT('Ctrl Pts',(22.4450937236828,-4.78805559974015,-3.37590058566347));
#78657=CARTESIAN_POINT('Ctrl Pts',(22.5643596961,0.248809890357853,-5.85322772741205));
#78658=CARTESIAN_POINT('Ctrl Pts',(22.6836256685171,5.05727224050727,-2.95739389934458));
#78659=CARTESIAN_POINT('Ctrl Pts',(22.8028916409343,5.22324687585818,2.65327594952422));
#78660=CARTESIAN_POINT('Ctrl Pts',(22.9221576133514,0.594371975859776,5.82828475151976));
#78661=CARTESIAN_POINT('Ctrl Pts',(23.0414235857686,-4.58012603175932,3.65302980054727));
#78662=CARTESIAN_POINT('Ctrl Pts',(23.1606895581858,-5.5501482224826,-1.87564279620591));
#78663=CARTESIAN_POINT('Ctrl Pts',(23.2799555306029,-1.42523114301903,-5.68250801842407));
#78664=CARTESIAN_POINT('Ctrl Pts',(23.3992215030202,4.00802326881451,-4.27292998621875));
#78665=CARTESIAN_POINT('Ctrl Pts',(23.5184874754372,5.76198222230599,1.0591232507672));
#78666=CARTESIAN_POINT('Ctrl Pts',(23.6377534478545,2.22654198829003,5.4189198153199));
#78667=CARTESIAN_POINT('Ctrl Pts',(23.7570194202715,-3.35282495869293,4.80424249875583));
#78668=CARTESIAN_POINT('Ctrl Pts',(23.8762853926888,-5.85435706895763,-0.220645642675769));
#78669=CARTESIAN_POINT('Ctrl Pts',(23.9955513651059,-2.9816914935637,-5.04298493232878));
#78670=CARTESIAN_POINT('Ctrl Pts',(24.1148173375231,2.62811487035934,-5.23595200691163));
#78671=CARTESIAN_POINT('Ctrl Pts',(24.2340833099403,5.82535761925768,-0.62240645742347));
#78672=CARTESIAN_POINT('Ctrl Pts',(24.3533492823574,3.67502367155342,4.56249736482195));
#78673=CARTESIAN_POINT('Ctrl Pts',(24.4726152547746,-1.84891791192818,5.55910817896513));
#78674=CARTESIAN_POINT('Ctrl Pts',(24.5918812271917,-5.67558509854319,1.4525546391377));
#78675=CARTESIAN_POINT('Ctrl Pts',(24.7111471996089,-4.29216415044515,-3.98741872595776));
#78676=CARTESIAN_POINT('Ctrl Pts',(24.8304131720261,1.03138862973723,-5.76701124369755));
#78677=CARTESIAN_POINT('Ctrl Pts',(24.9496791444432,5.40814463588299,-2.25258802000187));
#78678=CARTESIAN_POINT('Ctrl Pts',(25.0689451168604,4.82031818770908,3.32967171951333));
#78679=CARTESIAN_POINT('Ctrl Pts',(25.1882110892775,-0.192476287421281,
5.85535089207007));
#78680=CARTESIAN_POINT('Ctrl Pts',(25.3074770616947,-5.02858088760561,3.00592006668398));
#78681=CARTESIAN_POINT('Ctrl Pts',(25.4267430341119,-5.24853593456004,-2.6028929547943));
#78682=CARTESIAN_POINT('Ctrl Pts',(25.5460090065291,-0.650426531333829,
-5.82229563985052));
#78683=CARTESIAN_POINT('Ctrl Pts',(25.6652749789462,4.5447630838118,-3.6969324719972));
#78684=CARTESIAN_POINT('Ctrl Pts',(25.7845409513634,5.56793945152552,1.82215022833782));
#78685=CARTESIAN_POINT('Ctrl Pts',(25.9038069237805,1.47984451108115,5.66853079849693));
#78686=CARTESIAN_POINT('Ctrl Pts',(26.0230728961977,-3.96672188112297,4.31129895835422));
#78687=CARTESIAN_POINT('Ctrl Pts',(26.1423388686148,-5.77190676856384,-1.00363013381062));
#78688=CARTESIAN_POINT('Ctrl Pts',(26.2616048410321,-2.27858190812287,-5.39724426707374));
#78689=CARTESIAN_POINT('Ctrl Pts',(26.3808708134492,3.30644140408296,-4.83628229447494));
#78690=CARTESIAN_POINT('Ctrl Pts',(26.5001367858664,5.85620917374429,0.164302476667459));
#78691=CARTESIAN_POINT('Ctrl Pts',(26.6194027582835,3.03007905785472,5.01406043976691));
#78692=CARTESIAN_POINT('Ctrl Pts',(26.7386687307008,-2.57761078667377,5.26099836750677));
#78693=CARTESIAN_POINT('Ctrl Pts',(26.8579347031178,-5.81909888417815,0.678431548973455));
#78694=CARTESIAN_POINT('Ctrl Pts',(26.9772006755351,-3.71875569472669,-4.5269235992474));
#78695=CARTESIAN_POINT('Ctrl Pts',(27.0964666479522,1.79534036506138,-5.57664183573476));
#78696=CARTESIAN_POINT('Ctrl Pts',(27.2157326203694,5.66134528158068,-1.50710012713492));
#78697=CARTESIAN_POINT('Ctrl Pts',(27.3349985927865,4.33033396700724,3.94593321340702));
#78698=CARTESIAN_POINT('Ctrl Pts',(27.4542645652037,-0.975848405549228,
5.77666868358165));
#78699=CARTESIAN_POINT('Ctrl Pts',(27.5735305376208,-5.38621896121736,2.30452305093883));
#78700=CARTESIAN_POINT('Ctrl Pts',(27.6927965100381,-4.85213444951138,-3.28313455014414));
#78701=CARTESIAN_POINT('Ctrl Pts',(27.8120624824551,0.136124862590045,-5.85693189411237));
#78702=CARTESIAN_POINT('Ctrl Pts',(27.9313284548724,4.9994239249365,-3.05416790783649));
#78703=CARTESIAN_POINT('Ctrl Pts',(28.0505944272895,5.27333901726761,2.55226895123699));
#78704=CARTESIAN_POINT('Ctrl Pts',(28.1698603997067,0.706420862073846,5.81576742623987));
#78705=CARTESIAN_POINT('Ctrl Pts',(28.2891263721238,-4.50897932408263,3.74049283457156));
#78706=CARTESIAN_POINT('Ctrl Pts',(28.408392344541,-5.58521513014738,-1.76848894270167));
#78707=CARTESIAN_POINT('Ctrl Pts',(28.5276583169582,-1.53432085637788,-5.65402871412675));
#78708=CARTESIAN_POINT('Ctrl Pts',(28.6469242893753,3.92505320403234,-4.34926873577631));
#78709=CARTESIAN_POINT('Ctrl Pts',(28.7661902617925,5.78129687852069,0.948044088053002));
#78710=CARTESIAN_POINT('Ctrl Pts',(28.8854562342096,2.33041084795627,5.37506897353082));
#78711=CARTESIAN_POINT('Ctrl Pts',(29.0047222066268,-3.25975169721106,4.86787428586805));
#78712=CARTESIAN_POINT('Ctrl Pts',(29.123988179044,-5.85751903644455,-0.107944097453046));
#78713=CARTESIAN_POINT('Ctrl Pts',(29.2432541514612,-3.07818605901322,-4.98467168192475));
#78714=CARTESIAN_POINT('Ctrl Pts',(29.3625201238783,2.52686803510449,-5.28555759817761));
#78715=CARTESIAN_POINT('Ctrl Pts',(29.4817860962955,5.81230134315328,-0.734393822729839));
#78716=CARTESIAN_POINT('Ctrl Pts',(29.6010520687127,3.76214338835384,4.49093067369687));
#78717=CARTESIAN_POINT('Ctrl Pts',(29.7203180411298,-1.7415965828236,5.59365913630631));
#78718=CARTESIAN_POINT('Ctrl Pts',(29.839584013547,-5.64658126550127,1.56150606869626));
#78719=CARTESIAN_POINT('Ctrl Pts',(29.9588499859641,-4.36810282635358,-3.90408233633562));
#78720=CARTESIAN_POINT('Ctrl Pts',(30.0781159583813,0.920217824944716,-5.78579124624626));
#78721=CARTESIAN_POINT('Ctrl Pts',(30.1973819307985,5.36379456211742,-2.35624469991655));
#78722=CARTESIAN_POINT('Ctrl Pts',(30.3166479032156,4.88350143919435,3.23629338655699));
#78723=CARTESIAN_POINT('Ctrl Pts',(30.4359138756328,-0.079760833593354,
5.85797058714965));
#78724=CARTESIAN_POINT('Ctrl Pts',(30.55517984805,-4.96980405222106,3.10213295540542));
#78725=CARTESIAN_POINT('Ctrl Pts',(30.6744458204671,-5.29765382739722,-2.50140862626428));
#78726=CARTESIAN_POINT('Ctrl Pts',(30.7937117928843,-0.762349783414896,
-5.80870071515249));
#78727=CARTESIAN_POINT('Ctrl Pts',(30.9129777653015,4.47277806588579,-3.78370685489987));
#78728=CARTESIAN_POINT('Ctrl Pts',(31.0322437377186,5.601973658747,1.71466390793955));
#78729=CARTESIAN_POINT('Ctrl Pts',(31.1515097101358,1.5886551347986,5.63900310810021));
#78730=CARTESIAN_POINT('Ctrl Pts',(31.270775682553,-3.88302109575688,4.38683580276175));
#78731=CARTESIAN_POINT('Ctrl Pts',(31.3900416549701,-5.79015168272125,-0.89237026035508));
#78732=CARTESIAN_POINT('Ctrl Pts',(31.5093076273873,-2.38202400880994,-5.35239598796079));
#78733=CARTESIAN_POINT('Ctrl Pts',(31.6285735998044,3.21276016120207,-4.89901554774815));
#78734=CARTESIAN_POINT('Ctrl Pts',(31.7478395722217,5.85828653577487,0.0515757234056574));
#78735=CARTESIAN_POINT('Ctrl Pts',(31.8671055446387,3.12600804268317,4.95482137998596));
#78736=CARTESIAN_POINT('Ctrl Pts',(31.986371517056,-2.47589131405855,5.30962742491925));
#78737=CARTESIAN_POINT('Ctrl Pts',(32.1056374894731,-5.80496562558577,0.790288096995977));
#78738=CARTESIAN_POINT('Ctrl Pts',(32.2249034618903,-3.80518273505212,-4.45452192085157));
#78739=CARTESIAN_POINT('Ctrl Pts',(32.3441694343074,1.68769154149534,-5.61015850500237));
#78740=CARTESIAN_POINT('Ctrl Pts',(32.4634354067246,5.63129441734489,-1.61576742623007));
#78741=CARTESIAN_POINT('Ctrl Pts',(32.5827013791418,4.40546723136434,3.8618699698282));
#78742=CARTESIAN_POINT('Ctrl Pts',(32.7019673515589,-0.86450203890803,5.79437808700892));
#78743=CARTESIAN_POINT('Ctrl Pts',(32.8212333239761,-5.34087351491845,2.40774817788913));
#78744=CARTESIAN_POINT('Ctrl Pts',(32.9404992963932,-4.9144162524043,-3.1891525659006));
#78745=CARTESIAN_POINT('Ctrl Pts',(33.0597652688104,0.0233894193275074,
-5.85846687500652));
#78746=CARTESIAN_POINT('Ctrl Pts',(33.1790312412276,4.93972401204274,-3.14981076817866));
#78747=CARTESIAN_POINT('Ctrl Pts',(33.2982972136447,5.3214781135754,2.4503166891698));
#78748=CARTESIAN_POINT('Ctrl Pts',(33.4175631860619,0.818208116748437,5.80109616091408));
#78749=CARTESIAN_POINT('Ctrl Pts',(33.536829158479,-4.43616266119279,3.82657053168034));
#78750=CARTESIAN_POINT('Ctrl Pts',(33.6560951308962,-5.61821348560732,-1.6606801078555));
#78751=CARTESIAN_POINT('Ctrl Pts',(33.7753611033134,-1.6428423153869,-5.62345537167841));
#78752=CARTESIAN_POINT('Ctrl Pts',(33.8946270757306,3.8406294481618,-4.42399668087533));
#78753=CARTESIAN_POINT('Ctrl Pts',(34.0138930481477,5.79847036127596,0.836613805705633));
#78754=CARTESIAN_POINT('Ctrl Pts',(34.1331590205649,2.43341661168203,5.32922740971606));
#78755=CARTESIAN_POINT('Ctrl Pts',(34.2524249929821,-3.16547114712599,4.92970319666262));
#78756=CARTESIAN_POINT('Ctrl Pts',(34.3716909653992,-5.85851160067448,0.00479742617581129));
#78757=CARTESIAN_POINT('Ctrl Pts',(34.4909569378164,-3.17354058089109,-4.92451229786949));
#78758=CARTESIAN_POINT('Ctrl Pts',(34.6102229102335,2.4246853435919,-5.33320561904289));
#78759=CARTESIAN_POINT('Ctrl Pts',(34.7294888826507,5.79709241073807,-0.846109196369897));
#78760=CARTESIAN_POINT('Ctrl Pts',(34.8487548550679,3.84786974963835,4.41770071189267));
#78761=CARTESIAN_POINT('Ctrl Pts',(34.9680208274851,-1.63363023218451,5.62613841410746));
#78762=CARTESIAN_POINT('Ctrl Pts',(35.0872867999022,-5.61548615275964,1.66987917552219));
#78763=CARTESIAN_POINT('Ctrl Pts',(35.2065527723194,-4.4424237219931,-3.81930002242228));
#78764=CARTESIAN_POINT('Ctrl Pts',(35.3258187447365,0.808706205598543,-5.80242841082625));
#78765=CARTESIAN_POINT('Ctrl Pts',(35.4450847171537,5.31745794329846,-2.45902871594494));
#78766=CARTESIAN_POINT('Ctrl Pts',(35.5643506895709,4.94487602407868,3.14171645294316));
#78767=CARTESIAN_POINT('Ctrl Pts',(35.6836166619881,0.0329841655221652,
5.85842071197083));
#78768=CARTESIAN_POINT('Ctrl Pts',(35.8028826344052,-4.90918659888947,3.1971969310834));
#78769=CARTESIAN_POINT('Ctrl Pts',(35.9221486068224,-5.34480965219109,-2.39899786982601));
#78770=CARTESIAN_POINT('Ctrl Pts',(36.0414145792395,-0.873990723536196,
-5.79295446929697));
#78771=CARTESIAN_POINT('Ctrl Pts',(36.1606805516567,4.39913656401214,-3.86907989292384));
#78772=CARTESIAN_POINT('Ctrl Pts',(36.2799465240739,5.6339329860754,1.60654253501617));
#78773=CARTESIAN_POINT('Ctrl Pts',(36.399212496491,1.69687761054767,5.60738695574555));
#78774=CARTESIAN_POINT('Ctrl Pts',(36.5184784689082,-3.79788262273949,4.46074790787285));
#78775=CARTESIAN_POINT('Ctrl Pts',(36.6377444413253,-5.8062513152231,-0.78077984606419));
#78776=CARTESIAN_POINT('Ctrl Pts',(36.7570104137426,-2.48458547192956,-5.30556546129872));
#78777=CARTESIAN_POINT('Ctrl Pts',(36.8762763861596,3.11789202290122,-4.95993424442102));
#78778=CARTESIAN_POINT('Ctrl Pts',(36.9955423585769,5.85818853286327,-0.0611704102445672));
#78779=CARTESIAN_POINT('Ctrl Pts',(37.114808330994,3.22079005536847,4.89374777128489));
#78780=CARTESIAN_POINT('Ctrl Pts',(37.2340743034112,-2.37327534445112,5.35628899208556));
#78781=CARTESIAN_POINT('Ctrl Pts',(37.3533402758283,-5.78864353195016,0.901853861538382));
#78782=CARTESIAN_POINT('Ctrl Pts',(37.4726062482455,-3.89027435237813,-4.38047408248273));
#78783=CARTESIAN_POINT('Ctrl Pts',(37.5918722206627,1.57955796423474,-5.64159049656991));
#78784=CARTESIAN_POINT('Ctrl Pts',(37.7111381930798,5.59889145836505,-1.72384938880929));
#78785=CARTESIAN_POINT('Ctrl Pts',(37.830404165497,4.47947502597244,3.77640129668631));
#78786=CARTESIAN_POINT('Ctrl Pts',(37.9496701379142,-0.753797156194961,
5.80989413817872));
#78787=CARTESIAN_POINT('Ctrl Pts',(38.0689361103313,-5.29172052081598,2.51017245988127));
#78788=CARTESIAN_POINT('Ctrl Pts',(38.1882020827485,-4.97837853386125,-3.09417052848874));
#78789=CARTESIAN_POINT('Ctrl Pts',(38.3074680551657,-0.0824858617694694,
-5.85741598647027));
#78790=CARTESIAN_POINT('Ctrl Pts',(38.4068563655133,4.03899355773438,-3.68100514101762));
#78791=CARTESIAN_POINT('Ctrl Pts',(38.4863670137914,5.13673732082221,-0.443168429242001));
#78792=CARTESIAN_POINT('Ctrl Pts',(38.5261223379305,4.8694790910934,1.22917467492147));
#78793=CARTESIAN_POINT('Ctrl Pts',(38.546,4.53891924175741,1.9850259738362));
#78794=CARTESIAN_POINT('Ctrl Pts',(-17.7840033022126,2.79181362996783,-3.91758709698588));
#78795=CARTESIAN_POINT('Ctrl Pts',(-17.764125640143,3.44419652954148,-3.45267555171637));
#78796=CARTESIAN_POINT('Ctrl Pts',(-17.724370316004,4.50091513856352,-2.19257893815165));
#78797=CARTESIAN_POINT('Ctrl Pts',(-17.6448596677259,5.20107532249908,1.05263844334769));
#78798=CARTESIAN_POINT('Ctrl Pts',(-17.5454713573782,2.85251838409021,4.92149809869413));
#78799=CARTESIAN_POINT('Ctrl Pts',(-17.4262053849611,-2.60480908979514,
5.06088873571236));
#78800=CARTESIAN_POINT('Ctrl Pts',(-17.3069394125439,-5.66091456100895,
0.547658985425077));
#78801=CARTESIAN_POINT('Ctrl Pts',(-17.1876734401267,-3.5256034875135,-4.4648272083155));
#78802=CARTESIAN_POINT('Ctrl Pts',(-17.0684074677096,1.84887983265183,-5.38050279906848));
#78803=CARTESIAN_POINT('Ctrl Pts',(-16.9491414952924,5.52468767357187,-1.35601227028438));
#78804=CARTESIAN_POINT('Ctrl Pts',(-16.8298755228753,4.12968454665724,3.91276942512457));
#78805=CARTESIAN_POINT('Ctrl Pts',(-16.7106095504581,-1.05669498430824,
5.58996261315058));
#78806=CARTESIAN_POINT('Ctrl Pts',(-16.5913435780409,-5.27283738738912,
2.13552778114678));
#78807=CARTESIAN_POINT('Ctrl Pts',(-16.4720776056237,-4.648717369209,-3.27921068370341));
#78808=CARTESIAN_POINT('Ctrl Pts',(-16.3528116332066,0.242902213228417,
-5.68372969776847));
#78809=CARTESIAN_POINT('Ctrl Pts',(-16.2335456607894,4.91151121149745,-2.87066356623015));
#78810=CARTESIAN_POINT('Ctrl Pts',(-16.1142796883723,5.07145468313125,2.57761090616478));
#78811=CARTESIAN_POINT('Ctrl Pts',(-15.9950137159551,0.575882724972399,
5.65968918026788));
#78812=CARTESIAN_POINT('Ctrl Pts',(-15.8757477435379,-4.44833506603484,
3.54626851611126));
#78813=CARTESIAN_POINT('Ctrl Pts',(-15.7564817711208,-5.38906119904768,
-1.82256322803374));
#78814=CARTESIAN_POINT('Ctrl Pts',(-15.6372157987036,-1.38272190213506,
-5.51831454142211));
#78815=CARTESIAN_POINT('Ctrl Pts',(-15.5179498262864,3.89293133367724,-4.1483489137632));
#78816=CARTESIAN_POINT('Ctrl Pts',(-15.3986838538693,5.59494184347711,1.02972843796234));
#78817=CARTESIAN_POINT('Ctrl Pts',(-15.2794178814521,2.16089313957021,5.26253316330437));
#78818=CARTESIAN_POINT('Ctrl Pts',(-15.160151909035,-3.25681768400598,4.66442416312198));
#78819=CARTESIAN_POINT('Ctrl Pts',(-15.0408859366178,-5.68482672468769,
-0.215544834913055));
#78820=CARTESIAN_POINT('Ctrl Pts',(-14.9216199642006,-2.89426395266302,
-4.89764745133195));
#78821=CARTESIAN_POINT('Ctrl Pts',(-14.8023539917834,2.5531826362492,-5.08379511619378));
#78822=CARTESIAN_POINT('Ctrl Pts',(-14.6830880193663,5.65685210149595,-0.603107533830891));
#78823=CARTESIAN_POINT('Ctrl Pts',(-14.5638220469491,3.56762999275445,4.43122224858523));
#78824=CARTESIAN_POINT('Ctrl Pts',(-14.444556074532,-1.79661422561301,5.39776728873189));
#78825=CARTESIAN_POINT('Ctrl Pts',(-14.3252901021148,-5.51159792000934,
1.40925609896829));
#78826=CARTESIAN_POINT('Ctrl Pts',(-14.2060241296976,-4.16703084898607,
-3.87292761171638));
#78827=CARTESIAN_POINT('Ctrl Pts',(-14.0867581572805,1.00279786548942,-5.59983132092501));
#78828=CARTESIAN_POINT('Ctrl Pts',(-13.9674921848633,5.25207562902259,-2.18618754218488));
#78829=CARTESIAN_POINT('Ctrl Pts',(-13.8482262124461,4.68003956451101,3.23433827185923));
#78830=CARTESIAN_POINT('Ctrl Pts',(-13.7289602400289,-0.188191197364887,
5.68579796118773));
#78831=CARTESIAN_POINT('Ctrl Pts',(-13.6096942676118,-4.88366572225456,
2.91779428602944));
#78832=CARTESIAN_POINT('Ctrl Pts',(-13.4904282951946,-5.09602028828365,
-2.52869365555675));
#78833=CARTESIAN_POINT('Ctrl Pts',(-13.3711623227775,-0.630317107451957,
-5.65388492333468));
#78834=CARTESIAN_POINT('Ctrl Pts',(-13.2518963503603,4.41400618489981,-3.58890843877865));
#78835=CARTESIAN_POINT('Ctrl Pts',(-13.1326303779431,5.40634878253714,1.77062339977217));
#78836=CARTESIAN_POINT('Ctrl Pts',(-13.013364405526,1.43575748790641,5.50475383810973));
#78837=CARTESIAN_POINT('Ctrl Pts',(-12.8940984331088,-3.85283414011536,
4.18561625940866));
#78838=CARTESIAN_POINT('Ctrl Pts',(-12.7748324606917,-5.60459122334528,
-0.975844045667388));
#78839=CARTESIAN_POINT('Ctrl Pts',(-12.6555664882745,-2.21143131111649,
-5.24149653615046));
#78840=CARTESIAN_POINT('Ctrl Pts',(-12.5363005158573,3.21178397597373,-4.69554662142142));
#78841=CARTESIAN_POINT('Ctrl Pts',(-12.4170345434402,5.68663758863899,0.160833198506063));
#78842=CARTESIAN_POINT('Ctrl Pts',(-12.297768571023,2.94125707344572,4.86957094723645));
#78843=CARTESIAN_POINT('Ctrl Pts',(-12.1785025986058,-2.50414613780997,
5.10812749476314));
#78844=CARTESIAN_POINT('Ctrl Pts',(-12.0592366261887,-5.65078686842909,
0.657512091031845));
#78845=CARTESIAN_POINT('Ctrl Pts',(-11.9399706537715,-3.61010380708337,
-4.39668794484507));
#78846=CARTESIAN_POINT('Ctrl Pts',(-11.8207046813543,1.74459158669925,-5.41480512833859));
#78847=CARTESIAN_POINT('Ctrl Pts',(-11.7014387089372,5.49778233065907,-1.46222564160138));
#78848=CARTESIAN_POINT('Ctrl Pts',(-11.58217273652,4.20410477983222,3.83265148199726));
#78849=CARTESIAN_POINT('Ctrl Pts',(-11.4629067641028,-0.948867636666955,
5.60922138895852));
#78850=CARTESIAN_POINT('Ctrl Pts',(-11.3436407916857,-5.23079611155017,
2.236623889181));
#78851=CARTESIAN_POINT('Ctrl Pts',(-11.2243748192685,-4.71094498438226,
-3.18915533274683));
#78852=CARTESIAN_POINT('Ctrl Pts',(-11.1051088468514,0.133471476625133,
-5.68734558007435));
#78853=CARTESIAN_POINT('Ctrl Pts',(-10.9858428744342,4.85536344991656,-2.96465177575344));
#78854=CARTESIAN_POINT('Ctrl Pts',(-10.866576902017,5.12011645675633,2.47954065333013));
#78855=CARTESIAN_POINT('Ctrl Pts',(-10.7473109295998,0.684691854323342,
5.64755800739461));
#78856=CARTESIAN_POINT('Ctrl Pts',(-10.6280449571827,-4.37926792892479,
3.63121560761055));
#78857=CARTESIAN_POINT('Ctrl Pts',(-10.5087789847655,-5.42313613058841,
-1.71851938929136));
#78858=CARTESIAN_POINT('Ctrl Pts',(-10.3895130123484,-1.48865994725382,
-5.49068355887553));
#78859=CARTESIAN_POINT('Ctrl Pts',(-10.2702470399312,3.8123801045003,-4.22249598236326));
#78860=CARTESIAN_POINT('Ctrl Pts',(-10.150981067514,5.61372171061381,0.921869262990718));
#78861=CARTESIAN_POINT('Ctrl Pts',(-10.0317150950969,2.26176469319736,5.21997460289508));
#78862=CARTESIAN_POINT('Ctrl Pts',(-9.91244912267971,-3.16645286598505,
4.72623429695976));
#78863=CARTESIAN_POINT('Ctrl Pts',(-9.79318315026253,-5.6879219191093,-0.106106665105973));
#78864=CARTESIAN_POINT('Ctrl Pts',(-9.67391717784538,-2.98797785140271,
-4.84104355917095));
#78865=CARTESIAN_POINT('Ctrl Pts',(-9.5546512054282,2.4548777716912,-5.13198689674088));
#78866=CARTESIAN_POINT('Ctrl Pts',(-9.43538523301105,5.64419841497453,-0.711855768160145));
#78867=CARTESIAN_POINT('Ctrl Pts',(-9.31611926059388,3.65224335165753,4.36174654038232));
#78868=CARTESIAN_POINT('Ctrl Pts',(-9.19685328817672,-1.69240741107544,
5.43134159643826));
#78869=CARTESIAN_POINT('Ctrl Pts',(-9.07758731575955,-5.48345768708367,
1.51505979295432));
#78870=CARTESIAN_POINT('Ctrl Pts',(-8.95832134334239,-4.24078944127668,
-3.79202047687245));
#78871=CARTESIAN_POINT('Ctrl Pts',(-8.83905537092521,0.894849549605194,
-5.6180920841363));
#78872=CARTESIAN_POINT('Ctrl Pts',(-8.71978939850807,5.20903226068468,-2.28685314119865));
#78873=CARTESIAN_POINT('Ctrl Pts',(-8.60052342609088,4.74141420523234,3.14367710121201));
#78874=CARTESIAN_POINT('Ctrl Pts',(-8.48125745367373,-0.0787393973975508,
5.68836659240252));
#78875=CARTESIAN_POINT('Ctrl Pts',(-8.36199148125656,-4.82661160648078,
3.01123476043447));
#78876=CARTESIAN_POINT('Ctrl Pts',(-8.2427255088394,-5.14373853993627,-2.4301580637971));
#78877=CARTESIAN_POINT('Ctrl Pts',(-8.12345953642222,-0.739003203743718,
-5.64070816893767));
#78878=CARTESIAN_POINT('Ctrl Pts',(-8.00419356400507,4.34412418480804,-3.67318655246773));
#78879=CARTESIAN_POINT('Ctrl Pts',(-7.8849275915879,5.43942133594559,1.66625625649949));
#78880=CARTESIAN_POINT('Ctrl Pts',(-7.76566161917074,1.54142456759122,5.47610488255017));
#78881=CARTESIAN_POINT('Ctrl Pts',(-7.64639564675358,-3.7715730704045,4.25898473310993));
#78882=CARTESIAN_POINT('Ctrl Pts',(-7.5271296743364,-5.62233240835935,-0.867809121970914));
#78883=CARTESIAN_POINT('Ctrl Pts',(-7.40786370191925,-2.31188865242981,
-5.19796933821563));
#78884=CARTESIAN_POINT('Ctrl Pts',(-7.28859772950208,3.12082856564795,-4.75648435781088));
#78885=CARTESIAN_POINT('Ctrl Pts',(-7.16933175708492,5.68867958966067,0.0513703070056891));
#78886=CARTESIAN_POINT('Ctrl Pts',(-7.05006578466775,3.03442196449068,4.81206792592126));
#78887=CARTESIAN_POINT('Ctrl Pts',(-6.93079981225059,-2.40538210186704,
5.15537111431188));
#78888=CARTESIAN_POINT('Ctrl Pts',(-6.81153383983341,-5.63708735007736,
0.766133532657032));
#78889=CARTESIAN_POINT('Ctrl Pts',(-6.69226786741627,-3.69404472524156,
-4.32640127012959));
#78890=CARTESIAN_POINT('Ctrl Pts',(-6.57300189499908,1.6400665309183,-5.44737516207808));
#78891=CARTESIAN_POINT('Ctrl Pts',(-6.45373592258194,5.46862531548002,-1.56775366086475));
#78892=CARTESIAN_POINT('Ctrl Pts',(-6.33446995016476,4.27708143667285,3.75103835841921));
#78893=CARTESIAN_POINT('Ctrl Pts',(-6.2152039777476,-0.84074860602783,5.62644258512658));
#78894=CARTESIAN_POINT('Ctrl Pts',(-6.09593800533044,-5.18678609157587,
2.33687064736132));
#78895=CARTESIAN_POINT('Ctrl Pts',(-5.97667203291327,-4.77144440584691,
-3.09790778819772));
#78896=CARTESIAN_POINT('Ctrl Pts',(-5.85740606049611,0.0240000274783397,
-5.68886090363832));
#78897=CARTESIAN_POINT('Ctrl Pts',(-5.73814008807894,4.79741285415394,-3.05753892682699));
#78898=CARTESIAN_POINT('Ctrl Pts',(-5.61887411566178,5.16688435059337,2.38055045942261));
#78899=CARTESIAN_POINT('Ctrl Pts',(-5.49960814324461,0.793246126878927,
5.63333604220938));
#78900=CARTESIAN_POINT('Ctrl Pts',(-5.38034217082745,-4.30857820660237,
3.71481738714771));
#78901=CARTESIAN_POINT('Ctrl Pts',(-5.26107619841029,-5.4552028907182,-1.61383884057968));
#78902=CARTESIAN_POINT('Ctrl Pts',(-5.14181022599311,-1.59404646330102,
-5.46101915901246));
#78903=CARTESIAN_POINT('Ctrl Pts',(-5.02254425357596,3.73041681626036,-4.29507913305747));
#78904=CARTESIAN_POINT('Ctrl Pts',(-4.90327828115879,5.63042251929442,0.813668628181062));
#78905=CARTESIAN_POINT('Ctrl Pts',(-4.78401230874162,2.36179854770228,5.17548277963853));
#78906=CARTESIAN_POINT('Ctrl Pts',(-4.66474633632446,-3.07491529943844,
4.78629400304068));
#78907=CARTESIAN_POINT('Ctrl Pts',(-4.54548036390729,-5.68891053013843,
0.00337080760888953));
#78908=CARTESIAN_POINT('Ctrl Pts',(-4.42621439149013,-3.08058511232485,
-4.78264673041885));
#78909=CARTESIAN_POINT('Ctrl Pts',(-4.30694841907297,2.35566371127412,-5.17827798226882));
#78910=CARTESIAN_POINT('Ctrl Pts',(-4.1876824466558,5.62945433217017,-0.8203403587989));
#78911=CARTESIAN_POINT('Ctrl Pts',(-4.06841647423864,3.73550405733429,4.29065540680006));
#78912=CARTESIAN_POINT('Ctrl Pts',(-3.94915050182147,-1.58757379261008,
5.46290434066727));
#78913=CARTESIAN_POINT('Ctrl Pts',(-3.82988452940431,-5.45328658921714,
1.62030236626634));
#78914=CARTESIAN_POINT('Ctrl Pts',(-3.71061855698715,-4.31297740564767,
-3.7097089212816));
#78915=CARTESIAN_POINT('Ctrl Pts',(-3.59135258456998,0.786569815286035,
-5.63427211873411));
#78916=CARTESIAN_POINT('Ctrl Pts',(-3.47208661215282,5.16405966405615,-2.38667177641422));
#78917=CARTESIAN_POINT('Ctrl Pts',(-3.35282063973565,4.80103280564923,3.05185163160719));
#78918=CARTESIAN_POINT('Ctrl Pts',(-3.23355466731848,0.0307415646677118,
5.68882846801215));
#78919=CARTESIAN_POINT('Ctrl Pts',(-3.11428869490132,-4.76776989652671,
3.10355998750428));
#78920=CARTESIAN_POINT('Ctrl Pts',(-2.99502272248416,-5.18955174559502,
-2.33072243350754));
#78921=CARTESIAN_POINT('Ctrl Pts',(-2.87575675006699,-0.84741560123151,
-5.62544230981467));
#78922=CARTESIAN_POINT('Ctrl Pts',(-2.75649077764983,4.27263328560509,-3.75610425694008));
#78923=CARTESIAN_POINT('Ctrl Pts',(-2.63722480523266,5.47047933364981,1.56127199500084));
#78924=CARTESIAN_POINT('Ctrl Pts',(-2.5179588328155,1.64652076198106,5.44542778508989));
#78925=CARTESIAN_POINT('Ctrl Pts',(-2.39869286039833,-3.68891515283567,
4.3307758401288));
#78926=CARTESIAN_POINT('Ctrl Pts',(-2.27942688798117,-5.63799129433396,
-0.759452794634447));
#78927=CARTESIAN_POINT('Ctrl Pts',(-2.16016091556401,-2.41148975772396,
-5.15251700925442));
#78928=CARTESIAN_POINT('Ctrl Pts',(-2.04089494314684,3.02871731858882,-4.81566047249431));
#78929=CARTESIAN_POINT('Ctrl Pts',(-1.92162897072967,5.68861471915913,-0.058111610111389));
#78930=CARTESIAN_POINT('Ctrl Pts',(-1.80236299831251,3.12646302053577,4.75278269685096));
#78931=CARTESIAN_POINT('Ctrl Pts',(-1.68309702589535,-2.30572720347124,
5.20070537960349));
#78932=CARTESIAN_POINT('Ctrl Pts',(-1.56383105347818,-5.62130006801447,
0.874471227430688));
#78933=CARTESIAN_POINT('Ctrl Pts',(-1.44456508106102,-3.77661750910527,
-4.25451226019894));
#78934=CARTESIAN_POINT('Ctrl Pts',(-1.32529910864385,1.53493405659396,-5.47792769431762));
#78935=CARTESIAN_POINT('Ctrl Pts',(-1.20603313622669,5.43744292854874,-1.67270104353375));
#78936=CARTESIAN_POINT('Ctrl Pts',(-1.08676716380952,4.34847402449726,3.66803599226292));
#78937=CARTESIAN_POINT('Ctrl Pts',(-0.967501191392359,-0.73231819393922,
5.64157996000141));
#78938=CARTESIAN_POINT('Ctrl Pts',(-0.848235218975195,-5.14085508242627,
2.43625191713739));
#78939=CARTESIAN_POINT('Ctrl Pts',(-0.728969246558032,-4.83017666497017,
-3.00551289590335));
#78940=CARTESIAN_POINT('Ctrl Pts',(-0.609703274140865,-0.0854803103699123,
-5.68826928852731));
#78941=CARTESIAN_POINT('Ctrl Pts',(-0.490437301723702,4.7376854783199,-3.14929368125304));
#78942=CARTESIAN_POINT('Ctrl Pts',(-0.371171329306535,5.21173862610644,
2.28067859976231));
#78943=CARTESIAN_POINT('Ctrl Pts',(-0.251905356889374,0.901506611104705,
5.61702770265542));
#78944=CARTESIAN_POINT('Ctrl Pts',(-0.132639384472207,-4.23629275005268,
3.79704333898294));
#78945=CARTESIAN_POINT('Ctrl Pts',(-0.0133734120550438,-5.48524925025369,
-1.50856058706799));
#78946=CARTESIAN_POINT('Ctrl Pts',(0.105892560362122,-1.69884260489541,
-5.42933220442958));
#78947=CARTESIAN_POINT('Ctrl Pts',(0.225158532779286,3.64707192288057,-4.36607154907015));
#78948=CARTESIAN_POINT('Ctrl Pts',(0.344424505196449,5.64503803266485,0.705166641320319));
#78949=CARTESIAN_POINT('Ctrl Pts',(0.463690477613616,2.46095768145258,5.12907415352552));
#78950=CARTESIAN_POINT('Ctrl Pts',(0.582956450030778,-2.98223890069384,
4.84458104705164));
#78951=CARTESIAN_POINT('Ctrl Pts',(0.702222422447946,-5.68779218411275,
0.112847031904288));
#78952=CARTESIAN_POINT('Ctrl Pts',(0.821488394865107,-3.17205144116504,
-4.72247859040851));
#78953=CARTESIAN_POINT('Ctrl Pts',(0.940754367282274,2.25557720221346,-5.22265122970302));
#78954=CARTESIAN_POINT('Ctrl Pts',(1.06002033969944,5.61262531263547,-0.928521126430262));
#78955=CARTESIAN_POINT('Ctrl Pts',(1.1792863121166,3.81738127374981,4.21797517691703));
#78956=CARTESIAN_POINT('Ctrl Pts',(1.29855228453377,-1.48215219692403,5.49244383197651));
#78957=CARTESIAN_POINT('Ctrl Pts',(1.41781825695093,-5.42109580048183,1.72494484093319));
#78958=CARTESIAN_POINT('Ctrl Pts',(1.5370842293681,-4.38356800649465,-3.62602342997124));
#78959=CARTESIAN_POINT('Ctrl Pts',(1.65635020178526,0.677998765290155,-5.64836543227584));
#78960=CARTESIAN_POINT('Ctrl Pts',(1.77561617420243,5.1171744952606,-2.48560647877295));
#78961=CARTESIAN_POINT('Ctrl Pts',(1.89488214661959,4.85887328530176,2.95889587171378));
#78962=CARTESIAN_POINT('Ctrl Pts',(2.01414811903676,0.140211141221322,5.68718341695967));
#78963=CARTESIAN_POINT('Ctrl Pts',(2.13341409145392,-4.70716238513036,3.1947357734682));
#78964=CARTESIAN_POINT('Ctrl Pts',(2.25268006387108,-5.23344293778499,-2.23042359187943));
#78965=CARTESIAN_POINT('Ctrl Pts',(2.37194603628825,-0.955514148067151,
-5.60809299986253));
#78966=CARTESIAN_POINT('Ctrl Pts',(2.49121200870541,4.19955996481265,-3.83763084261715));
#78967=CARTESIAN_POINT('Ctrl Pts',(2.61047798112258,5.49951127294373,1.4557094974715));
#78968=CARTESIAN_POINT('Ctrl Pts',(2.72974395353974,1.75100714742461,5.41273390736434));
#78969=CARTESIAN_POINT('Ctrl Pts',(2.84900992595691,-3.60489100077176,4.40096299175742));
#78970=CARTESIAN_POINT('Ctrl Pts',(2.96827589837407,-5.65156208181073,-0.650815194738936));
#78971=CARTESIAN_POINT('Ctrl Pts',(3.08754187079124,-2.51019773852067,-5.1051563830885));
#78972=CARTESIAN_POINT('Ctrl Pts',(3.2068078432084,2.93548434931463,-4.87305304887937));
#78973=CARTESIAN_POINT('Ctrl Pts',(3.32607381562557,5.68644300116001,-0.167572004888354));
#78974=CARTESIAN_POINT('Ctrl Pts',(3.44533978804273,3.21734615305874,4.69173721702972));
#78975=CARTESIAN_POINT('Ctrl Pts',(3.5646057604599,-2.20521835102361,5.24411350054252));
#78976=CARTESIAN_POINT('Ctrl Pts',(3.68387173287706,-5.60343086925195,0.982485051172806));
#78977=CARTESIAN_POINT('Ctrl Pts',(3.80313770529422,-3.85779157684188,-4.18104754002049));
#78978=CARTESIAN_POINT('Ctrl Pts',(3.92240367771139,1.42923310081396,-5.50645140955604));
#78979=CARTESIAN_POINT('Ctrl Pts',(4.04166965012854,5.4042467186407,-1.77702892107158));
#78980=CARTESIAN_POINT('Ctrl Pts',(4.16093562254572,4.41825610219412,3.58367512446205));
#78981=CARTESIAN_POINT('Ctrl Pts',(4.28020159496288,-0.623616558920145,
5.65462790727246));
#78982=CARTESIAN_POINT('Ctrl Pts',(4.39946756738005,-5.09302009520808,2.53473089144989));
#78983=CARTESIAN_POINT('Ctrl Pts',(4.51873353979721,-4.88712000954709,-2.91200487543344));
#78984=CARTESIAN_POINT('Ctrl Pts',(4.63799951221437,-0.194928989547843,
-5.68557095385308));
#78985=CARTESIAN_POINT('Ctrl Pts',(4.75726548463154,4.67620344317297,-3.23988205654479));
#78986=CARTESIAN_POINT('Ctrl Pts',(4.8765314570487,5.25466267097029,2.17996206310455));
#78987=CARTESIAN_POINT('Ctrl Pts',(4.99579742946587,1.00943321141648,5.59863902872416));
#78988=CARTESIAN_POINT('Ctrl Pts',(5.11506340188303,-4.16243833107186,3.8778630097371));
#78989=CARTESIAN_POINT('Ctrl Pts',(5.23432937430019,-5.51326408116101,-1.40272361983516));
#78990=CARTESIAN_POINT('Ctrl Pts',(5.35359534671737,-1.80300955951409,-5.39563443077501));
#78991=CARTESIAN_POINT('Ctrl Pts',(5.47286131913451,3.5623762921537,-4.4354469374985));
#78992=CARTESIAN_POINT('Ctrl Pts',(5.5921272915517,5.65756283769236,0.596403487436154));
#78993=CARTESIAN_POINT('Ctrl Pts',(5.71139326396885,2.55920536965963,5.08076591255386));
#78994=CARTESIAN_POINT('Ctrl Pts',(5.83065923638603,-2.88845799358026,4.90107384167857));
#78995=CARTESIAN_POINT('Ctrl Pts',(5.94992520880318,-5.6845672952253,0.222281461931913));
#78996=CARTESIAN_POINT('Ctrl Pts',(6.06919118122036,-3.26234296225833,-4.66056142314072));
#78997=CARTESIAN_POINT('Ctrl Pts',(6.1884571536375,2.15465531276254,-5.26509020487283));
#78998=CARTESIAN_POINT('Ctrl Pts',(6.30772312605469,5.59371758920206,-1.03635800499401));
#78999=CARTESIAN_POINT('Ctrl Pts',(6.42698909847184,3.89784467668328,4.14373276873832));
#79000=CARTESIAN_POINT('Ctrl Pts',(6.546255070889,-1.3761816681846,5.51994913005693));
#79001=CARTESIAN_POINT('Ctrl Pts',(6.66552104330618,-5.38689724312701,1.82894846134447));
#79002=CARTESIAN_POINT('Ctrl Pts',(6.78478701572333,-4.45253509973197,-3.54099499687852));
#79003=CARTESIAN_POINT('Ctrl Pts',(6.9040529881405,0.569176610223374,-5.66036680513182));
#79004=CARTESIAN_POINT('Ctrl Pts',(7.02331896055767,5.06839411878929,-2.58362060660727));
#79005=CARTESIAN_POINT('Ctrl Pts',(7.14258493297483,4.91491422226634,2.86484424882539));
#79006=CARTESIAN_POINT('Ctrl Pts',(7.26185090539199,0.249628788877266,5.68343204850972));
#79007=CARTESIAN_POINT('Ctrl Pts',(7.38111687780916,-4.64481151901909,3.28472835026752));
#79008=CARTESIAN_POINT('Ctrl Pts',(7.50038285022633,-5.27539586087048,-2.12929868580585));
#79009=CARTESIAN_POINT('Ctrl Pts',(7.61964882264348,-1.0632588086421,-5.58866666460871));
#79010=CARTESIAN_POINT('Ctrl Pts',(7.73891479506065,4.12493128602183,-3.91773611513867));
#79011=CARTESIAN_POINT('Ctrl Pts',(7.85818076747781,5.52650640149627,1.3496078602634));
#79012=CARTESIAN_POINT('Ctrl Pts',(7.97744673989498,1.85484502612115,5.37803535794785));
#79013=CARTESIAN_POINT('Ctrl Pts',(8.09671271231215,-3.51953173357715,4.4695201933325));
#79014=CARTESIAN_POINT('Ctrl Pts',(8.21597868472931,-5.66303974468377,-0.541936557537787));
#79015=CARTESIAN_POINT('Ctrl Pts',(8.33524465714647,-2.60797603712152,-5.05590500030049));
#79016=CARTESIAN_POINT('Ctrl Pts',(8.45451062956364,2.84116418778695,-4.92864083092901));
#79017=CARTESIAN_POINT('Ctrl Pts',(8.5737766019808,5.68216523998536,-0.276970337339723));
#79018=CARTESIAN_POINT('Ctrl Pts',(8.69304257439796,3.30703770238863,4.62895409539172));
#79019=CARTESIAN_POINT('Ctrl Pts',(8.81230854681514,-2.10389276919738,5.28557940040471));
#79020=CARTESIAN_POINT('Ctrl Pts',(8.9315745192323,-5.58348637186443,1.09013499965285));
#79021=CARTESIAN_POINT('Ctrl Pts',(9.05084049164945,-3.93753686465025,-4.10603431814493));
#79022=CARTESIAN_POINT('Ctrl Pts',(9.17010646406663,1.32300281121011,-5.53293574368922));
#79023=CARTESIAN_POINT('Ctrl Pts',(9.28937243648379,5.36904898037513,-1.88069865438264));
#79024=CARTESIAN_POINT('Ctrl Pts',(9.40863840890096,4.48640182512404,3.4979869990878));
#79025=CARTESIAN_POINT('Ctrl Pts',(9.52790438131812,-0.514683959940392,
5.6655815944741));
#79026=CARTESIAN_POINT('Ctrl Pts',(9.64717035373528,-5.0432988461893,2.63227109741554));
#79027=CARTESIAN_POINT('Ctrl Pts',(9.76643632615245,-4.94225334991895,-2.81741835861816));
#79028=CARTESIAN_POINT('Ctrl Pts',(9.88570229856962,-0.304305474408852,
-5.68076689897664));
#79029=CARTESIAN_POINT('Ctrl Pts',(10.0049682709868,4.61298951933098,-3.32927050219805));
#79030=CARTESIAN_POINT('Ctrl Pts',(10.124234243404,5.29564058774396,2.07843815104094));
#79031=CARTESIAN_POINT('Ctrl Pts',(10.2435002158211,1.11698595588803,5.57817683088416));
#79032=CARTESIAN_POINT('Ctrl Pts',(10.3627661882383,-4.08704230254025,3.95724646686431));
#79033=CARTESIAN_POINT('Ctrl Pts',(10.4820321606554,-5.53923700780752,-1.29636713688644));
#79034=CARTESIAN_POINT('Ctrl Pts',(10.6012981330726,-1.90650874766131,-5.3599383184282));
#79035=CARTESIAN_POINT('Ctrl Pts',(10.7205641054898,3.47636129213444,-4.50317960432547));
#79036=CARTESIAN_POINT('Ctrl Pts',(10.8398300779069,5.66799229566339,0.487419448282535));
#79037=CARTESIAN_POINT('Ctrl Pts',(10.9590960503241,2.65650522509982,5.03057594826689));
#79038=CARTESIAN_POINT('Ctrl Pts',(11.0783620227412,-2.79360731099475,4.95575146412935));
#79039=CARTESIAN_POINT('Ctrl Pts',(11.1976279951584,-5.6792370578528,0.331633567322531));
#79040=CARTESIAN_POINT('Ctrl Pts',(11.3168939675756,-3.35142623504413,-4.59691816038984));
#79041=CARTESIAN_POINT('Ctrl Pts',(11.4361599399928,2.05293542056789,-5.30557918998872));
#79042=CARTESIAN_POINT('Ctrl Pts',(11.5554259124099,5.57273816457474,-1.14381105579353));
#79043=CARTESIAN_POINT('Ctrl Pts',(11.6746918848271,3.976864465537,4.06795567884079));
#79044=CARTESIAN_POINT('Ctrl Pts',(11.7939578572443,-1.26970145386314,5.5454100479876));
#79045=CARTESIAN_POINT('Ctrl Pts',(11.9132238296614,-5.35070358300338,1.93227470849723));
#79046=CARTESIAN_POINT('Ctrl Pts',(12.0324898020786,-4.51985314255969,-3.45465511331554));
#79047=CARTESIAN_POINT('Ctrl Pts',(12.1517557744957,0.460143653691493,-5.670271792448));
#79048=CARTESIAN_POINT('Ctrl Pts',(12.2710217469129,5.01773660104659,-2.68067785919545));
#79049=CARTESIAN_POINT('Ctrl Pts',(12.3902877193301,4.96913486110191,2.76973159610198));
#79050=CARTESIAN_POINT('Ctrl Pts',(12.5095536917472,0.358953983481827,5.67757575202713));
#79051=CARTESIAN_POINT('Ctrl Pts',(12.6288196641644,-4.5807403905928,3.37350438805925));
#79052=CARTESIAN_POINT('Ctrl Pts',(12.7480856365816,-5.31539497707732,-2.027385168123));
#79053=CARTESIAN_POINT('Ctrl Pts',(12.8673516089987,-1.17060967841375,-5.56717049883224));
#79054=CARTESIAN_POINT('Ctrl Pts',(12.9866175814159,4.04877488886951,-3.99639040654476));
#79055=CARTESIAN_POINT('Ctrl Pts',(13.1058835538331,5.55145472133397,1.24300637940549));
#79056=CARTESIAN_POINT('Ctrl Pts',(13.2251495262502,1.95799594045214,5.34134498786934));
#79057=CARTESIAN_POINT('Ctrl Pts',(13.3444154986674,-3.43286896509233,4.53642205386241));
#79058=CARTESIAN_POINT('Ctrl Pts',(13.4636814710845,-5.67242003206137,-0.4328572075556));
#79059=CARTESIAN_POINT('Ctrl Pts',(13.5829474435017,-2.70478844014697,-5.00478110173774));
#79060=CARTESIAN_POINT('Ctrl Pts',(13.7022134159189,2.74579176662222,-4.98240323103349));
#79061=CARTESIAN_POINT('Ctrl Pts',(13.8214793883361,5.67578301995597,-0.386266090465443));
#79062=CARTESIAN_POINT('Ctrl Pts',(13.9407453607532,3.39550445017166,4.56445658442803));
#79063=CARTESIAN_POINT('Ctrl Pts',(14.0600113331704,-2.00178798515141,5.32508772179077));
#79064=CARTESIAN_POINT('Ctrl Pts',(14.1792773055875,-5.5614739625385,1.19738120340612));
#79065=CARTESIAN_POINT('Ctrl Pts',(14.2985432780047,-4.0158238378954,-4.02950037662921));
#79066=CARTESIAN_POINT('Ctrl Pts',(14.4178092504218,1.21628253145922,-5.55737088792268));
#79067=CARTESIAN_POINT('Ctrl Pts',(14.537075222839,5.33186274966146,-1.9836718481232));
#79068=CARTESIAN_POINT('Ctrl Pts',(14.6563411952562,4.55288595469166,3.41100335177722));
#79069=CARTESIAN_POINT('Ctrl Pts',(14.7756071676734,-0.405560741509822,
5.67443696477539));
#79070=CARTESIAN_POINT('Ctrl Pts',(14.8948731400905,-4.99170975023798,2.72883640983535));
#79071=CARTESIAN_POINT('Ctrl Pts',(15.0141391125077,-4.99555626678405,-2.72178837672192));
#79072=CARTESIAN_POINT('Ctrl Pts',(15.1334050849249,-0.413569256044401,
-5.67385890313799));
#79073=CARTESIAN_POINT('Ctrl Pts',(15.252671057342,4.54806711883782,-3.41742591211722));
#79074=CARTESIAN_POINT('Ctrl Pts',(15.3719370297592,5.33465719975868,1.97614446418445));
#79075=CARTESIAN_POINT('Ctrl Pts',(15.4912030021763,1.2241250110552,5.55564868755867));
#79076=CARTESIAN_POINT('Ctrl Pts',(15.6104689745935,-4.01013258829202,4.03516430973787));
#79077=CARTESIAN_POINT('Ctrl Pts',(15.7297349470107,-5.56315841080468,-1.18953052863603));
#79078=CARTESIAN_POINT('Ctrl Pts',(15.8490009194279,-2.00930183715662,-5.3222570878775));
#79079=CARTESIAN_POINT('Ctrl Pts',(15.968266891845,3.38905877952192,-4.56924446393595));
#79080=CARTESIAN_POINT('Ctrl Pts',(16.0875328642622,5.67632254390165,0.378254887421002));
#79081=CARTESIAN_POINT('Ctrl Pts',(16.2067988366793,2.75282121159081,4.97852284912694));
#79082=CARTESIAN_POINT('Ctrl Pts',(16.3260648090965,-2.69772198203872,5.00859366388301));
#79083=CARTESIAN_POINT('Ctrl Pts',(16.4453307815137,-5.67180344611339,0.440862848196796));
#79084=CARTESIAN_POINT('Ctrl Pts',(16.5645967539308,-3.43926826645123,-4.53157237321053));
#79085=CARTESIAN_POINT('Ctrl Pts',(16.683862726348,1.95045519882603,-5.34410318946374));
#79086=CARTESIAN_POINT('Ctrl Pts',(16.8031286987652,5.54969480873816,-1.25084048228728));
#79087=CARTESIAN_POINT('Ctrl Pts',(16.9223946711823,4.05441137437299,3.99067197218942));
#79088=CARTESIAN_POINT('Ctrl Pts',(17.0416606435995,-1.16275099019935,5.56881715600848));
#79089=CARTESIAN_POINT('Ctrl Pts',(17.1609266160167,-5.31252822487239,2.03488531426176));
#79090=CARTESIAN_POINT('Ctrl Pts',(17.2801925884338,-4.58549720292351,-3.36703575630613));
#79091=CARTESIAN_POINT('Ctrl Pts',(17.399458560851,0.350940277373286,-5.67807672579202));
#79092=CARTESIAN_POINT('Ctrl Pts',(17.5187245332682,4.96522070365914,-2.77674229020602));
#79093=CARTESIAN_POINT('Ctrl Pts',(17.6379905056853,5.02151512053671,2.67359313966889));
#79094=CARTESIAN_POINT('Ctrl Pts',(17.7572564781025,0.468146235122306,5.66961669646236));
#79095=CARTESIAN_POINT('Ctrl Pts',(17.8765224505196,-4.51497272937164,3.46103100756037));
#79096=CARTESIAN_POINT('Ctrl Pts',(17.9957884229368,-5.35342547224728,-1.92472078373913));
#79097=CARTESIAN_POINT('Ctrl Pts',(18.115054395354,-1.27752699868453,-5.54361246389897));
#79098=CARTESIAN_POINT('Ctrl Pts',(18.2343203677711,3.97111897880176,-4.07356458626403));
#79099=CARTESIAN_POINT('Ctrl Pts',(18.3535863401883,5.57434699254372,1.13594453605012));
#79100=CARTESIAN_POINT('Ctrl Pts',(18.4728523126054,2.06042168722449,5.3026763858526));
#79101=CARTESIAN_POINT('Ctrl Pts',(18.5921182850226,-3.34493479192551,4.60164379543117));
#79102=CARTESIAN_POINT('Ctrl Pts',(18.7113842574398,-5.67969946984019,-0.323617543653628));
#79103=CARTESIAN_POINT('Ctrl Pts',(18.8306502298569,-2.80059909194854,-4.95180362175652));
#79104=CARTESIAN_POINT('Ctrl Pts',(18.9499162022741,2.64940240815424,-5.03432033763551));
#79105=CARTESIAN_POINT('Ctrl Pts',(19.0691821746913,5.66729870480444,-0.495418785256739));
#79106=CARTESIAN_POINT('Ctrl Pts',(19.1884481471084,3.48271363167404,4.4982685715746));
#79107=CARTESIAN_POINT('Ctrl Pts',(19.3077141195256,-1.8989418146318,5.36262383231444));
#79108=CARTESIAN_POINT('Ctrl Pts',(19.4269800919428,-5.5374017938371,1.3041839424993));
#79109=CARTESIAN_POINT('Ctrl Pts',(19.54624606436,-4.09262350204653,-3.95147406074749));
#79110=CARTESIAN_POINT('Ctrl Pts',(19.6655120367771,1.10911178671227,-5.57974779240423));
#79111=CARTESIAN_POINT('Ctrl Pts',(19.7847780091943,5.29270179887156,-2.08591036492105));
#79112=CARTESIAN_POINT('Ctrl Pts',(19.9040439816114,4.61768386769258,3.32275639797979));
#79113=CARTESIAN_POINT('Ctrl Pts',(20.0233099540286,-0.296287318736919,
5.68119073848253));
#79114=CARTESIAN_POINT('Ctrl Pts',(20.1425759264458,-4.93827191400179,2.82439106457381));
#79115=CARTESIAN_POINT('Ctrl Pts',(20.2618418988629,-5.04700901876023,-2.62515034746904));
#79116=CARTESIAN_POINT('Ctrl Pts',(20.3811078712801,-0.522679867286884,
-5.66484952479737));
#79117=CARTESIAN_POINT('Ctrl Pts',(20.5003738436973,4.48146028649235,-3.50431563687621));
#79118=CARTESIAN_POINT('Ctrl Pts',(20.6196398161144,5.37169805673866,1.87311888824337));
#79119=CARTESIAN_POINT('Ctrl Pts',(20.7389057885316,1.33081069666864,5.53106294231917));
#79120=CARTESIAN_POINT('Ctrl Pts',(20.8581717609487,-3.93173767277321,4.11158768053889));
#79121=CARTESIAN_POINT('Ctrl Pts',(20.9774377333659,-5.5850194305705,-1.08225336331834));
#79122=CARTESIAN_POINT('Ctrl Pts',(21.0967037057831,-2.11135075733188,-5.28260469482414));
#79123=CARTESIAN_POINT('Ctrl Pts',(21.2159696782002,3.3005010878612,-4.63361704840726));
#79124=CARTESIAN_POINT('Ctrl Pts',(21.3352356506174,5.68255049719854,0.268950235271458));
#79125=CARTESIAN_POINT('Ctrl Pts',(21.4545016230346,2.84811765733817,4.92462589363116));
#79126=CARTESIAN_POINT('Ctrl Pts',(21.5737675954518,-2.60083751900743,5.05958087018941));
#79127=CARTESIAN_POINT('Ctrl Pts',(21.6930335678689,-5.66226921313533,0.549928850164967));
#79128=CARTESIAN_POINT('Ctrl Pts',(21.8122995402861,-3.52583652311729,-4.46454826320829));
#79129=CARTESIAN_POINT('Ctrl Pts',(21.9315655127032,1.84725260233084,-5.38064793546701));
#79130=CARTESIAN_POINT('Ctrl Pts',(22.0508314851204,5.52459605607864,-1.35740664482838));
#79131=CARTESIAN_POINT('Ctrl Pts',(22.1700974575375,4.1304566827527,3.91191027174289));
#79132=CARTESIAN_POINT('Ctrl Pts',(22.2893634299547,-1.05536988759536,5.59016178501306));
#79133=CARTESIAN_POINT('Ctrl Pts',(22.4086294023719,-5.272385307441,2.13674227555503));
#79134=CARTESIAN_POINT('Ctrl Pts',(22.5278953747891,-4.64944296874926,-3.27816937674247));
#79135=CARTESIAN_POINT('Ctrl Pts',(22.6471613472062,0.241606926064419,-5.68377871451211));
#79136=CARTESIAN_POINT('Ctrl Pts',(22.7664273196234,4.91086587652667,-2.87177832101119));
#79137=CARTESIAN_POINT('Ctrl Pts',(22.8856932920405,5.07203560090617,2.57646448557016));
#79138=CARTESIAN_POINT('Ctrl Pts',(23.0049592644577,0.577165103123198,5.65955782954818));
#79139=CARTESIAN_POINT('Ctrl Pts',(23.1242252368749,-4.44753289320691,3.54727579222515));
#79140=CARTESIAN_POINT('Ctrl Pts',(23.243491209292,-5.38947326132513,-1.82134355565483));
#79141=CARTESIAN_POINT('Ctrl Pts',(23.3627571817092,-1.38397117132737,-5.51800128481301));
#79142=CARTESIAN_POINT('Ctrl Pts',(23.4820231541263,3.8919923166271,-4.14923007190245));
#79143=CARTESIAN_POINT('Ctrl Pts',(23.6012891265436,5.59517473669525,1.02846198185014));
#79144=CARTESIAN_POINT('Ctrl Pts',(23.7205550989607,2.16208433181988,5.26204387328368));
#79145=CARTESIAN_POINT('Ctrl Pts',(23.8398210713778,-3.2557617815647,4.66516126237524));
#79146=CARTESIAN_POINT('Ctrl Pts',(23.9590870437951,-5.68487536199228,-0.214258024066976));
#79147=CARTESIAN_POINT('Ctrl Pts',(24.0783530162122,-2.89537250788858,-4.89699218120943));
#79148=CARTESIAN_POINT('Ctrl Pts',(24.1976189886294,2.55203181135149,-5.08437292260451));
#79149=CARTESIAN_POINT('Ctrl Pts',(24.3168849610465,5.65671543680001,-0.60438799568858));
#79150=CARTESIAN_POINT('Ctrl Pts',(24.4361509334637,3.56863294791704,4.43041457036519));
#79151=CARTESIAN_POINT('Ctrl Pts',(24.5554169058808,-1.79539234796575,5.39817383002159));
#79152=CARTESIAN_POINT('Ctrl Pts',(24.674682878298,-5.51127878118019,1.41050366124196));
#79153=CARTESIAN_POINT('Ctrl Pts',(24.7939488507152,-4.167907413416,-3.87198426849273));
#79154=CARTESIAN_POINT('Ctrl Pts',(24.9132148231323,1.0015302689549,-5.60005816957561));
#79155=CARTESIAN_POINT('Ctrl Pts',(25.0324807955495,5.25158063173888,-2.18737633950104));
#79156=CARTESIAN_POINT('Ctrl Pts',(25.1517467679667,4.68077156543346,3.23327882102573));
#79157=CARTESIAN_POINT('Ctrl Pts',(25.2710127403838,-0.186904162359676,
5.68584041425328));
#79158=CARTESIAN_POINT('Ctrl Pts',(25.390278712801,-4.88300512883198,2.9188996718052));
#79159=CARTESIAN_POINT('Ctrl Pts',(25.5095446852182,-5.09659254969641,-2.52754006192641));
#79160=CARTESIAN_POINT('Ctrl Pts',(25.6288106576353,-0.631596897697456,
-5.65374210068714));
#79161=CARTESIAN_POINT('Ctrl Pts',(25.7480766300525,4.4131936909433,-3.58990749581131));
#79162=CARTESIAN_POINT('Ctrl Pts',(25.8673426024697,5.40674944015302,1.76939957999003));
#79163=CARTESIAN_POINT('Ctrl Pts',(25.9866085748868,1.43700350039011,5.50442870079447));
#79164=CARTESIAN_POINT('Ctrl Pts',(26.105874547304,-3.85188659049215,4.18648827494485));
#79165=CARTESIAN_POINT('Ctrl Pts',(26.2251405197212,-5.60481197061107,-0.974575372333387));
#79166=CARTESIAN_POINT('Ctrl Pts',(26.3444064921383,-2.21261771313111,-5.24099582501282));
#79167=CARTESIAN_POINT('Ctrl Pts',(26.4636724645555,3.21072101556802,-4.69627351657181));
#79168=CARTESIAN_POINT('Ctrl Pts',(26.5829384369726,5.68667384895602,0.159545974138274));
#79169=CARTESIAN_POINT('Ctrl Pts',(26.7022044093899,2.94235926814676,4.86890504317082));
#79170=CARTESIAN_POINT('Ctrl Pts',(26.821470381807,-2.50298980423744,5.10869419931819));
#79171=CARTESIAN_POINT('Ctrl Pts',(26.9407363542241,-5.65063789003752,0.658791179309665));
#79172=CARTESIAN_POINT('Ctrl Pts',(27.0600023266413,-3.61109894343789,-4.39587065357536));
#79173=CARTESIAN_POINT('Ctrl Pts',(27.1792682990585,1.74336585341623,-5.41519989320858));
#79174=CARTESIAN_POINT('Ctrl Pts',(27.2985342714756,5.49745120222388,-1.4634700753453));
#79175=CARTESIAN_POINT('Ctrl Pts',(27.4178002438928,4.2049722263732,3.83169974785256));
#79176=CARTESIAN_POINT('Ctrl Pts',(27.53706621631,-0.947597915945529,5.60943602975911));
#79177=CARTESIAN_POINT('Ctrl Pts',(27.6563321887271,-5.23028969812594,2.23780786841534));
#79178=CARTESIAN_POINT('Ctrl Pts',(27.7755981611443,-4.71166675694639,-3.18808888736647));
#79179=CARTESIAN_POINT('Ctrl Pts',(27.8948641335614,0.132184092698237,-5.68737564680772));
#79180=CARTESIAN_POINT('Ctrl Pts',(28.0141301059787,4.8546922506191,-2.96575075386364));
#79181=CARTESIAN_POINT('Ctrl Pts',(28.1333960783957,5.12067759133716,2.47838160658135));
#79182=CARTESIAN_POINT('Ctrl Pts',(28.252662050813,0.685970211023877,5.64740287670818));
#79183=CARTESIAN_POINT('Ctrl Pts',(28.3719280232301,-4.37844585926038,3.63220680025098));
#79184=CARTESIAN_POINT('Ctrl Pts',(28.4911939956473,-5.42352499357456,-1.71729177088093));
#79185=CARTESIAN_POINT('Ctrl Pts',(28.6104599680644,-1.48990277345135,-5.49034644698546));
#79186=CARTESIAN_POINT('Ctrl Pts',(28.7297259404816,3.81142420786515,-4.22335883982919));
#79187=CARTESIAN_POINT('Ctrl Pts',(28.8489919128988,5.61393023998058,0.920598524273739));
#79188=CARTESIAN_POINT('Ctrl Pts',(28.9682578853159,2.26294622224433,5.21946249890676));
#79189=CARTESIAN_POINT('Ctrl Pts',(29.0875238577331,-3.16538296031649,4.72695093022996));
#79190=CARTESIAN_POINT('Ctrl Pts',(29.2067898301503,-5.68794579156296,-0.104819151420763));
#79191=CARTESIAN_POINT('Ctrl Pts',(29.3260558025674,-2.9890735874826,-4.84036708017872));
#79192=CARTESIAN_POINT('Ctrl Pts',(29.4453217749846,2.45371603859621,-5.13254244835828));
#79193=CARTESIAN_POINT('Ctrl Pts',(29.5645877474018,5.64403713558418,-0.71313336369156));
#79194=CARTESIAN_POINT('Ctrl Pts',(29.6838537198189,3.65323057763945,4.36091971135265));
#79195=CARTESIAN_POINT('Ctrl Pts',(29.8031196922361,-1.69117793595491,5.43172454853918));
#79196=CARTESIAN_POINT('Ctrl Pts',(29.9223856646532,-5.48311459954228,1.51630098283608));
#79197=CARTESIAN_POINT('Ctrl Pts',(30.0416516370704,-4.24164768969385,-3.79106043987415));
#79198=CARTESIAN_POINT('Ctrl Pts',(30.1609176094876,0.89357782230812,-5.61829449724229));
#79199=CARTESIAN_POINT('Ctrl Pts',(30.2801835819047,5.20851447798661,-2.28803219270779));
#79200=CARTESIAN_POINT('Ctrl Pts',(30.3994495543219,4.74212568261973,3.14260376002165));
#79201=CARTESIAN_POINT('Ctrl Pts',(30.5187155267391,-0.0774517837577881,
5.68838427002401));
#79202=CARTESIAN_POINT('Ctrl Pts',(30.6379814991563,-4.8259298634531,3.01232722911953));
#79203=CARTESIAN_POINT('Ctrl Pts',(30.7572474715734,-5.14428849573012,-2.42899367124797));
#79204=CARTESIAN_POINT('Ctrl Pts',(30.8765134439906,-0.740280008531856,
-5.64054074457688));
#79205=CARTESIAN_POINT('Ctrl Pts',(30.9957794164077,4.34329261555279,-3.67416978893845));
#79206=CARTESIAN_POINT('Ctrl Pts',(31.1150453888249,5.43979836829653,1.66502495312906));
#79207=CARTESIAN_POINT('Ctrl Pts',(31.2343113612421,1.5426640924258,5.47575582729946));
#79208=CARTESIAN_POINT('Ctrl Pts',(31.3535773336592,-3.77060891526627,4.25983835261126));
#79209=CARTESIAN_POINT('Ctrl Pts',(31.4728433060765,-5.62252870051896,-0.866536435532014));
#79210=CARTESIAN_POINT('Ctrl Pts',(31.5921092784935,-2.31306519910814,-5.19744588879372));
#79211=CARTESIAN_POINT('Ctrl Pts',(31.7113752509108,3.11975181378185,-4.7571906628459));
#79212=CARTESIAN_POINT('Ctrl Pts',(31.8306412233278,5.6886910720407,0.0500826232173974));
#79213=CARTESIAN_POINT('Ctrl Pts',(31.9499071957451,3.03551114049219,4.81138093463942));
#79214=CARTESIAN_POINT('Ctrl Pts',(32.0691731681622,-2.40421507681752,5.15591546155158));
#79215=CARTESIAN_POINT('Ctrl Pts',(32.1884391405794,-5.63691378462165,0.767409517146029));
#79216=CARTESIAN_POINT('Ctrl Pts',(32.3077051129966,-3.69502394944088,-4.32556497989826));
#79217=CARTESIAN_POINT('Ctrl Pts',(32.4269710854137,1.63883342780062,-5.44774626595132));
#79218=CARTESIAN_POINT('Ctrl Pts',(32.5462370578309,5.46827030059994,-1.56899149195925));
#79219=CARTESIAN_POINT('Ctrl Pts',(32.665503030248,4.27793040749859,3.7500701074597));
#79220=CARTESIAN_POINT('Ctrl Pts',(32.7847690026652,-0.839474989907709,
5.62663275179595));
#79221=CARTESIAN_POINT('Ctrl Pts',(32.9040349750823,-5.18625698754698,2.33804466197375));
#79222=CARTESIAN_POINT('Ctrl Pts',(33.0233009474996,-4.77214552217987,-3.09682765058092));
#79223=CARTESIAN_POINT('Ctrl Pts',(33.1425669199166,0.0227123033492882,
-5.68886619051107));
#79224=CARTESIAN_POINT('Ctrl Pts',(33.2618328923339,4.79672063052055,-3.05862478493235));
#79225=CARTESIAN_POINT('Ctrl Pts',(33.381098864751,5.16742307667829,2.37938082888736));
#79226=CARTESIAN_POINT('Ctrl Pts',(33.5003648371682,0.794521261531888,5.63315633967645));
#79227=CARTESIAN_POINT('Ctrl Pts',(33.6196308095853,-4.30773721475356,3.71579257640827));
#79228=CARTESIAN_POINT('Ctrl Pts',(33.7388967820025,-5.45556805752349,-1.61260396625899));
#79229=CARTESIAN_POINT('Ctrl Pts',(33.8581627544197,-1.59528257200157,-5.46065819272098));
#79230=CARTESIAN_POINT('Ctrl Pts',(33.9774287268369,3.72944449189255,-4.29592343555539));
#79231=CARTESIAN_POINT('Ctrl Pts',(34.096694699254,5.63060655607218,0.812394111861771));
#79232=CARTESIAN_POINT('Ctrl Pts',(34.2159606716712,2.36297000307123,5.17494803325048));
#79233=CARTESIAN_POINT('Ctrl Pts',(34.3352266440884,-3.07383180107209,4.78698991444201));
#79234=CARTESIAN_POINT('Ctrl Pts',(34.4544926165055,-5.68890962138567,0.00465854226991125));
#79235=CARTESIAN_POINT('Ctrl Pts',(34.5737585889227,-3.08166762739048,-4.78194929045732));
#79236=CARTESIAN_POINT('Ctrl Pts',(34.6930245613398,2.35449150231328,-5.17881107472906));
#79237=CARTESIAN_POINT('Ctrl Pts',(34.812290533757,5.629268496748,-0.82161461409729));
#79238=CARTESIAN_POINT('Ctrl Pts',(34.9315565061742,3.73647518902874,4.28980973279877));
#79239=CARTESIAN_POINT('Ctrl Pts',(35.0508224785913,-1.58633717557033,5.4632635619564));
#79240=CARTESIAN_POINT('Ctrl Pts',(35.1700884510085,-5.45291968006245,1.62153672395));
#79241=CARTESIAN_POINT('Ctrl Pts',(35.2893544234257,-4.31381701990819,-3.70873254599588));
#79242=CARTESIAN_POINT('Ctrl Pts',(35.4086203958428,0.785294427576647,-5.63445002139296));
#79243=CARTESIAN_POINT('Ctrl Pts',(35.52788636826,5.16351928900528,-2.38784064536003));
#79244=CARTESIAN_POINT('Ctrl Pts',(35.6471523406771,4.80172349350685,3.05076479745392));
#79245=CARTESIAN_POINT('Ctrl Pts',(35.7664183130943,0.0320292848053549,
5.68882136388004));
#79246=CARTESIAN_POINT('Ctrl Pts',(35.8856842855114,-4.76706726540989,3.10463913404421));
#79247=CARTESIAN_POINT('Ctrl Pts',(36.0049502579287,-5.19007917494346,-2.32954767244375));
#79248=CARTESIAN_POINT('Ctrl Pts',(36.1242162303458,-0.84868898024466,-5.62525034734734));
#79249=CARTESIAN_POINT('Ctrl Pts',(36.243482202763,4.27178301087878,-3.7570713056591));
#79250=CARTESIAN_POINT('Ctrl Pts',(36.3627481751801,5.47083248363574,1.56003365830421));
#79251=CARTESIAN_POINT('Ctrl Pts',(36.4820141475973,1.64775356318288,5.44505495213162));
#79252=CARTESIAN_POINT('Ctrl Pts',(36.6012801200144,-3.68793517297259,4.33161072664821));
#79253=CARTESIAN_POINT('Ctrl Pts',(36.7205460924317,-5.63816225396792,-0.758176526943501));
#79254=CARTESIAN_POINT('Ctrl Pts',(36.8398120648488,-2.41265754168496,-5.15197109043847));
#79255=CARTESIAN_POINT('Ctrl Pts',(36.959078037266,3.02763007680679,-4.81634578333499));
#79256=CARTESIAN_POINT('Ctrl Pts',(37.0783440096831,5.68859590628108,-0.0593995470360426));
#79257=CARTESIAN_POINT('Ctrl Pts',(37.1976099821003,3.12754924515988,4.75207538677428));
#79258=CARTESIAN_POINT('Ctrl Pts',(37.3168759545174,-2.30456980569776,5.20122619173273));
#79259=CARTESIAN_POINT('Ctrl Pts',(37.4361419269346,-5.6210642102154,0.875745489588154));
#79260=CARTESIAN_POINT('Ctrl Pts',(37.5554078993518,-3.7776521925,-4.25366080203663));
#79261=CARTESIAN_POINT('Ctrl Pts',(37.674673871769,1.53383028195009,-5.47826831172611));
#79262=CARTESIAN_POINT('Ctrl Pts',(37.7939398441861,5.43680539659932,-1.67394451735641));
#79263=CARTESIAN_POINT('Ctrl Pts',(37.9132058166033,4.34979570085314,3.66707572422626));
#79264=CARTESIAN_POINT('Ctrl Pts',(38.0324717890204,-0.731974977049794,
5.64169961840002));
#79265=CARTESIAN_POINT('Ctrl Pts',(38.1517377614376,-5.13852695641803,2.43750379477149));
#79266=CARTESIAN_POINT('Ctrl Pts',(38.2710037338548,-4.83425611667699,-3.00459531183657));
#79267=CARTESIAN_POINT('Ctrl Pts',(38.3902697062719,-0.0800979232670034,
-5.68784572485145));
#79268=CARTESIAN_POINT('Ctrl Pts',(38.4896580166196,3.92206602589366,-3.57444125581233));
#79269=CARTESIAN_POINT('Ctrl Pts',(38.5691686648977,4.98803046896621,-0.430338849328192));
#79270=CARTESIAN_POINT('Ctrl Pts',(38.6089239890367,4.72850927687308,1.19359047334112));
#79271=CARTESIAN_POINT('Ctrl Pts',(38.6288016511063,4.40751902618983,1.92756012635639));
#79272=CARTESIAN_POINT('Ctrl Pts',(-17.7012016511063,2.70858201811927,-3.80079309428511));
#79273=CARTESIAN_POINT('Ctrl Pts',(-17.6813239890368,3.34151559640192,-3.34974183569964));
#79274=CARTESIAN_POINT('Ctrl Pts',(-17.6415686648977,4.36673052904853,-2.12721215393368));
#79275=CARTESIAN_POINT('Ctrl Pts',(-17.5620580166196,5.04601701997133,1.0212564078875));
#79276=CARTESIAN_POINT('Ctrl Pts',(-17.462669706272,2.76747699723466,4.77477475904616));
#79277=CARTESIAN_POINT('Ctrl Pts',(-17.3434037338548,-2.52715259554554,
4.91000977934608));
#79278=CARTESIAN_POINT('Ctrl Pts',(-17.2241377614376,-5.49214719115606,
0.531331770882378));
#79279=CARTESIAN_POINT('Ctrl Pts',(-17.1048717890205,-3.42049558996118,
-4.33171847885584));
#79280=CARTESIAN_POINT('Ctrl Pts',(-16.9856058166033,1.79375966025411,-5.22009527196343));
#79281=CARTESIAN_POINT('Ctrl Pts',(-16.8663398441861,5.35998160039607,-1.31558583001987));
#79282=CARTESIAN_POINT('Ctrl Pts',(-16.747073871769,4.00656733798903,3.79611905041868));
#79283=CARTESIAN_POINT('Ctrl Pts',(-16.6278078993518,-1.02519201225003,
5.42331051522014));
#79284=CARTESIAN_POINT('Ctrl Pts',(-16.5085419269346,-5.11563966113103,
2.07186184819784));
#79285=CARTESIAN_POINT('Ctrl Pts',(-16.3892759545175,-4.51012637032802,
-3.18144843056949));
#79286=CARTESIAN_POINT('Ctrl Pts',(-16.2700099821003,0.235660632876478,
-5.51428214619193));
#79287=CARTESIAN_POINT('Ctrl Pts',(-16.1507440096831,4.76508560831362,-2.78508122179041));
#79288=CARTESIAN_POINT('Ctrl Pts',(-16.031478037266,4.9202607269294,2.50076526427245));
#79289=CARTESIAN_POINT('Ctrl Pts',(-15.9122120648488,0.558714083441273,
5.49095834237153));
#79290=CARTESIAN_POINT('Ctrl Pts',(-15.7929460924317,-4.31571801251304,
3.4405445374493));
#79291=CARTESIAN_POINT('Ctrl Pts',(-15.6736801200144,-5.22839852259545,
-1.76822762570804));
#79292=CARTESIAN_POINT('Ctrl Pts',(-15.5544141475974,-1.34149917458011,
-5.35379846877344));
#79293=CARTESIAN_POINT('Ctrl Pts',(-15.4351481751801,3.77687238681933,-4.02467526918476));
#79294=CARTESIAN_POINT('Ctrl Pts',(-15.315882202763,5.42814130105117,0.999029412519419));
#79295=CARTESIAN_POINT('Ctrl Pts',(-15.1966162303458,2.09647099580402,5.10564263419233));
#79296=CARTESIAN_POINT('Ctrl Pts',(-15.0773502579287,-3.15972302753357,
4.52536490168926));
#79297=CARTESIAN_POINT('Ctrl Pts',(-14.9580842855115,-5.51534646773363,
-0.209118852948021));
#79298=CARTESIAN_POINT('Ctrl Pts',(-14.8388183130943,-2.80797801605581,
-4.75163516481528));
#79299=CARTESIAN_POINT('Ctrl Pts',(-14.7195523406772,2.47706526799874,-4.93223325787853));
#79300=CARTESIAN_POINT('Ctrl Pts',(-14.60028636826,5.48820584468934,-0.585127246171516));
#79301=CARTESIAN_POINT('Ctrl Pts',(-14.4810203958428,3.46126916995884,4.29911537502828));
#79302=CARTESIAN_POINT('Ctrl Pts',(-14.3617544234257,-1.74305223413087,
5.23684505989782));
#79303=CARTESIAN_POINT('Ctrl Pts',(-14.2424884510085,-5.34728208824364,
1.36724231432135));
#79304=CARTESIAN_POINT('Ctrl Pts',(-14.1232224785913,-4.04280024474373,
-3.75746503060578));
#79305=CARTESIAN_POINT('Ctrl Pts',(-14.0039565061742,0.972901714182095,
-5.43288500978274));
#79306=CARTESIAN_POINT('Ctrl Pts',(-13.884690533757,5.09549686765353,-2.12101130298848));
#79307=CARTESIAN_POINT('Ctrl Pts',(-13.7654245613399,4.54051476518803,3.13791378824016));
#79308=CARTESIAN_POINT('Ctrl Pts',(-13.6461585889227,-0.182580702264231,
5.51628874901311));
#79309=CARTESIAN_POINT('Ctrl Pts',(-13.5268926165055,-4.73807026938147,
2.83080684572858));
#79310=CARTESIAN_POINT('Ctrl Pts',(-13.4076266440883,-4.94409396410031,
-2.45330637090273));
#79311=CARTESIAN_POINT('Ctrl Pts',(-13.2883606716712,-0.611525627868499,
-5.48532712623696));
#79312=CARTESIAN_POINT('Ctrl Pts',(-13.169094699254,4.28241256936083,-3.48191324721959));
#79313=CARTESIAN_POINT('Ctrl Pts',(-13.0498287268369,5.24517071586569,1.71783626600429));
#79314=CARTESIAN_POINT('Ctrl Pts',(-12.9305627544197,1.39295362426069,5.34064204717326));
#79315=CARTESIAN_POINT('Ctrl Pts',(-12.8112967820026,-3.73797060043469,
4.0608315731711));
#79316=CARTESIAN_POINT('Ctrl Pts',(-12.6920308095854,-5.43750300647318,
-0.946751461562825));
#79317=CARTESIAN_POINT('Ctrl Pts',(-12.5727648371682,-2.14550248601868,
-5.08523316651894));
#79318=CARTESIAN_POINT('Ctrl Pts',(-12.453498864751,3.11603189769737,-4.55555951425388));
#79319=CARTESIAN_POINT('Ctrl Pts',(-12.3342328923339,5.51710334487009,0.156038320292407));
#79320=CARTESIAN_POINT('Ctrl Pts',(-12.2149669199167,2.85357014318101,4.72439569821608));
#79321=CARTESIAN_POINT('Ctrl Pts',(-12.0957009474996,-2.42949068190233,
4.95584022158971));
#79322=CARTESIAN_POINT('Ctrl Pts',(-11.9764349750824,-5.48232143283452,
0.637909854493391));
#79323=CARTESIAN_POINT('Ctrl Pts',(-11.8571690026652,-3.50247672353525,
-4.26561063348149));
#79324=CARTESIAN_POINT('Ctrl Pts',(-11.737903030248,1.69258053258732,-5.25337495483456));
#79325=CARTESIAN_POINT('Ctrl Pts',(-11.6186370578309,5.33387837945656,-1.41863268979052));
#79326=CARTESIAN_POINT('Ctrl Pts',(-11.4993710854137,4.07876890015574,3.71838964264088));
#79327=CARTESIAN_POINT('Ctrl Pts',(-11.3801051129966,-0.920579293210441,
5.44199513416622));
#79328=CARTESIAN_POINT('Ctrl Pts',(-11.2608391405794,-5.07485175088737,
2.16994400432173));
#79329=CARTESIAN_POINT('Ctrl Pts',(-11.1415731681622,-4.57049880983454,
-3.09407787631109));
#79330=CARTESIAN_POINT('Ctrl Pts',(-11.0223071957451,0.129492326291972,
-5.51779022914138));
#79331=CARTESIAN_POINT('Ctrl Pts',(-10.9030412233279,4.71061176530949,-2.87626738532846));
#79332=CARTESIAN_POINT('Ctrl Pts',(-10.7837752509108,4.96747175978485,2.40561875431596));
#79333=CARTESIAN_POINT('Ctrl Pts',(-10.6645092784936,0.664279314588377,
5.47918883299221));
#79334=CARTESIAN_POINT('Ctrl Pts',(-10.5452433060764,-4.24870995595397,
3.52295912345773));
#79335=CARTESIAN_POINT('Ctrl Pts',(-10.4259773336592,-5.26145758708642,
-1.66728561880302));
#79336=CARTESIAN_POINT('Ctrl Pts',(-10.3067113612421,-1.44427891638068,
-5.32699124150536));
#79337=CARTESIAN_POINT('Ctrl Pts',(-10.1874453888249,3.69872261043595,-4.09661181056081));
#79338=CARTESIAN_POINT('Ctrl Pts',(-10.0681794164077,5.44636128890534,0.894385815009405));
#79339=CARTESIAN_POINT('Ctrl Pts',(-9.94891344399059,2.19433529210285,5.06435286104834));
#79340=CARTESIAN_POINT('Ctrl Pts',(-9.82964747157342,-3.07205223227173,
4.58533230612251));
#79341=CARTESIAN_POINT('Ctrl Pts',(-9.71038149915626,-5.51834938593094,
-0.102943334763881));
#79342=CARTESIAN_POINT('Ctrl Pts',(-9.59111552673909,-2.89889804676615,
-4.6967187897331));
#79343=CARTESIAN_POINT('Ctrl Pts',(-9.47184955432193,2.38169114073705,-4.97898830943708));
#79344=CARTESIAN_POINT('Ctrl Pts',(-9.35258358190476,5.47592939922501,-0.690633397744341));
#79345=CARTESIAN_POINT('Ctrl Pts',(-9.23331760948761,3.54335997285394,4.23171092799982));
#79346=CARTESIAN_POINT('Ctrl Pts',(-9.11405163707043,-1.64195211018554,
5.26941842552227));
#79347=CARTESIAN_POINT('Ctrl Pts',(-8.99478566465327,-5.31998079274526,
1.46989171036448));
#79348=CARTESIAN_POINT('Ctrl Pts',(-8.87551969223611,-4.11435989135324,
-3.67896995907826));
#79349=CARTESIAN_POINT('Ctrl Pts',(-8.75625371981893,0.868171633294266,
-5.45060136962148));
#79350=CARTESIAN_POINT('Ctrl Pts',(-8.63698774740178,5.05373674003329,-2.21867578474511));
#79351=CARTESIAN_POINT('Ctrl Pts',(-8.51772177498461,4.60005965974758,3.0499554754356));
#79352=CARTESIAN_POINT('Ctrl Pts',(-8.39845580256745,-0.0763919602722595,
5.51878080229521));
#79353=CARTESIAN_POINT('Ctrl Pts',(-8.27918983015028,-4.68271709308568,
2.92146160363265));
#79354=CARTESIAN_POINT('Ctrl Pts',(-8.15992385773312,-4.99038960395785,
-2.3577083950493));
#79355=CARTESIAN_POINT('Ctrl Pts',(-8.04065788531595,-0.716971493908937,
-5.47254320698324));
#79356=CARTESIAN_POINT('Ctrl Pts',(-7.92139191289879,4.21461394311765,-3.56367879947885));
#79357=CARTESIAN_POINT('Ctrl Pts',(-7.80212594048163,5.27725728586228,1.61658059316265));
#79358=CARTESIAN_POINT('Ctrl Pts',(-7.68285996806445,1.49547047884913,5.31284719545623));
#79359=CARTESIAN_POINT('Ctrl Pts',(-7.5635939956473,-3.65913214580814,4.13201273169507));
#79360=CARTESIAN_POINT('Ctrl Pts',(-7.44432802323013,-5.45471527816404,
-0.841937354878873));
#79361=CARTESIAN_POINT('Ctrl Pts',(-7.32506205081297,-2.24296491880738,
-5.04300363358741));
#79362=CARTESIAN_POINT('Ctrl Pts',(-7.2057960783958,3.02778811730507,-4.61468052979649));
#79363=CARTESIAN_POINT('Ctrl Pts',(-7.08653010597863,5.51908446824771,0.0498388174363854));
#79364=CARTESIAN_POINT('Ctrl Pts',(-6.96726413356148,2.94395753361986,4.66860699948275));
#79365=CARTESIAN_POINT('Ctrl Pts',(-6.8479981611443,-2.33367107241249,5.00167537942653));
#79366=CARTESIAN_POINT('Ctrl Pts',(-6.72873218872715,-5.46903033465158,
0.743292993399969));
#79367=CARTESIAN_POINT('Ctrl Pts',(-6.60946621630998,-3.58391513298606,
-4.19741939707365));
#79368=CARTESIAN_POINT('Ctrl Pts',(-6.49020024389281,1.59117165504184,-5.28497398665006));
#79369=CARTESIAN_POINT('Ctrl Pts',(-6.37093427147565,5.30559061476902,-1.52101462972962));
#79370=CARTESIAN_POINT('Ctrl Pts',(-6.25166829905848,4.14956992295298,3.63920962983732));
#79371=CARTESIAN_POINT('Ctrl Pts',(-6.13240232664132,-0.815683587042184,
5.45870291930293));
#79372=CARTESIAN_POINT('Ctrl Pts',(-6.01313635422416,-5.03215379016394,
2.26720213203748));
#79373=CARTESIAN_POINT('Ctrl Pts',(-5.89387038180699,-4.62919457782091,
-3.0055506710169));
#79374=CARTESIAN_POINT('Ctrl Pts',(-5.77460440938983,0.0232845209164049,
-5.51926037675902));
#79375=CARTESIAN_POINT('Ctrl Pts',(-5.65533843697266,4.65438883554905,-2.96638531598526));
#79376=CARTESIAN_POINT('Ctrl Pts',(-5.5360724645555,5.01284537459657,2.30957972924997));
#79377=CARTESIAN_POINT('Ctrl Pts',(-5.41680649213833,0.76959728691932,5.46539086354699));
#79378=CARTESIAN_POINT('Ctrl Pts',(-5.29754051972117,-4.18012768789241,
3.60406850493881));
#79379=CARTESIAN_POINT('Ctrl Pts',(-5.17827454730401,-5.29256834925714,
-1.56572588399702));
#79380=CARTESIAN_POINT('Ctrl Pts',(-5.05900857488683,-1.5465235717021,-5.29821121866109));
#79381=CARTESIAN_POINT('Ctrl Pts',(-4.93974260246968,3.61920287233824,-4.16703105870777));
#79382=CARTESIAN_POINT('Ctrl Pts',(-4.82047663005251,5.46256420073112,0.789410937514474));
#79383=CARTESIAN_POINT('Ctrl Pts',(-4.70121065763534,2.29138686338495,5.02118746091831));
#79384=CARTESIAN_POINT('Ctrl Pts',(-4.58194468521818,-2.98324365133024,
4.64360146784524));
#79385=CARTESIAN_POINT('Ctrl Pts',(-4.46267871280103,-5.51930852375722,
0.00327031460068596));
#79386=CARTESIAN_POINT('Ctrl Pts',(-4.34341274038385,-2.98874443156363,
-4.64006293041094));
#79387=CARTESIAN_POINT('Ctrl Pts',(-4.22414676796669,2.28543492323537,-5.02389933090152));
#79388=CARTESIAN_POINT('Ctrl Pts',(-4.10488079554952,5.46162487791711,-0.795883765567264));
#79389=CARTESIAN_POINT('Ctrl Pts',(-3.98561482313236,3.62413844882069,4.16273921584765));
#79390=CARTESIAN_POINT('Ctrl Pts',(-3.86634885071519,-1.54024386905451,
5.30004019788685));
#79391=CARTESIAN_POINT('Ctrl Pts',(-3.74708287829803,-5.29070917795299,
1.57199671427794));
#79392=CARTESIAN_POINT('Ctrl Pts',(-3.62781690588086,-4.18439573476381,
-3.59911233643337));
#79393=CARTESIAN_POINT('Ctrl Pts',(-3.5085509334637,0.76312001446289,-5.4662990330664));
#79394=CARTESIAN_POINT('Ctrl Pts',(-3.38928496104654,5.01010489970247,-2.31551855301444));
#79395=CARTESIAN_POINT('Ctrl Pts',(-3.27001898862937,4.65790086637442,2.96086757461472));
#79396=CARTESIAN_POINT('Ctrl Pts',(-3.1507530162122,0.0298250744156161,
5.5192289081277));
#79397=CARTESIAN_POINT('Ctrl Pts',(-3.03148704379505,-4.62562961568883,
3.01103436277953));
#79398=CARTESIAN_POINT('Ctrl Pts',(-2.91222107137787,-5.03483699246105,
-2.26123721327999));
#79399=CARTESIAN_POINT('Ctrl Pts',(-2.79295509896072,-0.822151820856484,
-5.45773246493805));
#79400=CARTESIAN_POINT('Ctrl Pts',(-2.67368912654355,4.145254383453,-3.64412450004667));
#79401=CARTESIAN_POINT('Ctrl Pts',(-2.55442315412639,5.30738935957861,1.5147262000798));
#79402=CARTESIAN_POINT('Ctrl Pts',(-2.43515718170922,1.59743346779706,5.28308466630418));
#79403=CARTESIAN_POINT('Ctrl Pts',(-2.31589120929206,-3.57893848718462,
4.20166354915829));
#79404=CARTESIAN_POINT('Ctrl Pts',(-2.19662523687489,-5.46990732985377,
-0.736811426477842));
#79405=CARTESIAN_POINT('Ctrl Pts',(-2.07735926445773,-2.33959664231811,
-4.99890636305885));
#79406=CARTESIAN_POINT('Ctrl Pts',(-1.95809329204056,2.93842295883862,-4.67209244240168));
#79407=CARTESIAN_POINT('Ctrl Pts',(-1.8388273196234,5.51902153171351,-0.056379143830598));
#79408=CARTESIAN_POINT('Ctrl Pts',(-1.71956134720623,3.0332545936587,4.61108922548945));
#79409=CARTESIAN_POINT('Ctrl Pts',(-1.60029537478907,-2.23698715951982,
5.04565810608688));
#79410=CARTESIAN_POINT('Ctrl Pts',(-1.4810294023719,-5.45371371471264,0.848400844725927));
#79411=CARTESIAN_POINT('Ctrl Pts',(-1.36176342995474,-3.66402619597342,
-4.12767359545265));
#79412=CARTESIAN_POINT('Ctrl Pts',(-1.24249745753757,1.48917346776363,-5.31461566421181));
#79413=CARTESIAN_POINT('Ctrl Pts',(-1.12323148512041,5.27533786020922,-1.62283324344174));
#79414=CARTESIAN_POINT('Ctrl Pts',(-1.00396551270325,4.21883410217057,3.55868179158226));
#79415=CARTESIAN_POINT('Ctrl Pts',(-0.884699540286082,-0.710485782558413,
5.47338900756735));
#79416=CARTESIAN_POINT('Ctrl Pts',(-0.765433567868916,-4.98759211021465,
2.36362057392911));
#79417=CARTESIAN_POINT('Ctrl Pts',(-0.646167595451754,-4.68617586741602,
-2.91591032355664));
#79418=CARTESIAN_POINT('Ctrl Pts',(-0.526901623034587,-0.0829319081640793,
-5.51868639931506));
#79419=CARTESIAN_POINT('Ctrl Pts',(-0.407635650617423,4.5964420963982,-3.05540460984056));
#79420=CARTESIAN_POINT('Ctrl Pts',(-0.288369678200257,5.05636242128851,
2.21268532330241));
#79421=CARTESIAN_POINT('Ctrl Pts',(-0.169103705783095,0.874630229555327,
5.44956872026812));
#79422=CARTESIAN_POINT('Ctrl Pts',(-0.0498377333659291,-4.10999725881205,
3.68384307591051));
#79423=CARTESIAN_POINT('Ctrl Pts',(0.0694282390512345,-5.3217189445097,
-1.46358626360836));
#79424=CARTESIAN_POINT('Ctrl Pts',(0.188694211468401,-1.64819545325033,
-5.26746893899353));
#79425=CARTESIAN_POINT('Ctrl Pts',(0.307960183885564,3.5383427185345,-4.23590699633152));
#79426=CARTESIAN_POINT('Ctrl Pts',(0.427226156302729,5.47674398561209,0.684143692098591));
#79427=CARTESIAN_POINT('Ctrl Pts',(0.546492128719893,2.38758979173424,4.97616240307561));
#79428=CARTESIAN_POINT('Ctrl Pts',(0.665758101137058,-2.89333018989815,
4.70015081541011));
#79429=CARTESIAN_POINT('Ctrl Pts',(0.785024073554225,-5.51822351869001,
0.109482752764602));
#79430=CARTESIAN_POINT('Ctrl Pts',(0.904290045971388,-3.07748389858988,
-4.58168856747125));
#79431=CARTESIAN_POINT('Ctrl Pts',(1.02355601838855,2.18833226717407,-5.06694969027927));
#79432=CARTESIAN_POINT('Ctrl Pts',(1.14282199080572,5.445297577554,-0.9008393681789));
#79433=CARTESIAN_POINT('Ctrl Pts',(1.26208796322288,3.70357468113084,4.09222578270839));
#79434=CARTESIAN_POINT('Ctrl Pts',(1.38135393564004,-1.43796517991438,5.32869903604344));
#79435=CARTESIAN_POINT('Ctrl Pts',(1.50061990805721,-5.25947808480922,1.67351951013068));
#79436=CARTESIAN_POINT('Ctrl Pts',(1.61988588047437,-4.25288183643263,-3.51792173885636));
#79437=CARTESIAN_POINT('Ctrl Pts',(1.73915185289153,0.657785764873116,-5.47997218632601));
#79438=CARTESIAN_POINT('Ctrl Pts',(1.8584178253087,4.96461750621998,-2.41150374088671));
#79439=CARTESIAN_POINT('Ctrl Pts',(1.97768379772586,4.71401696288765,2.87068308055491));
#79440=CARTESIAN_POINT('Ctrl Pts',(2.09694977014304,0.136031063025135,5.51763290055334));
#79441=CARTESIAN_POINT('Ctrl Pts',(2.21621574256019,-4.56682898022772,3.09949194880851));
#79442=CARTESIAN_POINT('Ctrl Pts',(2.33548171497737,-5.07741966798188,-2.1639285548667));
#79443=CARTESIAN_POINT('Ctrl Pts',(2.45474768739452,-0.927027653899548,
-5.44090038544007));
#79444=CARTESIAN_POINT('Ctrl Pts',(2.57401365981169,4.07435957852114,-3.72322055488116));
#79445=CARTESIAN_POINT('Ctrl Pts',(2.69327963222886,5.33555577723577,1.4123108097663));
#79446=CARTESIAN_POINT('Ctrl Pts',(2.81254560464602,1.69880482787383,5.25136548263106));
#79447=CARTESIAN_POINT('Ctrl Pts',(2.93181157706318,-3.49741932525881,4.2697582295351));
#79448=CARTESIAN_POINT('Ctrl Pts',(3.05107754948035,-5.48307353498178,-0.631412611023234));
#79449=CARTESIAN_POINT('Ctrl Pts',(3.17034352189751,-2.43536186781919,-4.95295768689262));
#79450=CARTESIAN_POINT('Ctrl Pts',(3.28960949431468,2.84796951976903,-4.72777398887077));
#79451=CARTESIAN_POINT('Ctrl Pts',(3.40887546673184,5.51691455857687,-0.162576224397382));
#79452=CARTESIAN_POINT('Ctrl Pts',(3.528141439149,3.12142825104746,4.55186367864189));
#79453=CARTESIAN_POINT('Ctrl Pts',(3.64740741156617,-2.13947475128482,5.08777211203403));
#79454=CARTESIAN_POINT('Ctrl Pts',(3.76667338398333,-5.43637724571383,0.953194480502964));
#79455=CARTESIAN_POINT('Ctrl Pts',(3.88593935640051,-3.74278024239289,-4.05639905982263));
#79456=CARTESIAN_POINT('Ctrl Pts',(4.00520532881766,1.38662374701919,-5.34228900936473));
#79457=CARTESIAN_POINT('Ctrl Pts',(4.12447130123482,5.24313132025201,-1.72405082116765));
#79458=CARTESIAN_POINT('Ctrl Pts',(4.24373727365199,4.28653578497914,3.47683595233796));
#79459=CARTESIAN_POINT('Ctrl Pts',(4.36300324606916,-0.605024841042691,
5.48604795978835));
#79460=CARTESIAN_POINT('Ctrl Pts',(4.48226921848632,-4.9411832149985,2.45916362025659));
#79461=CARTESIAN_POINT('Ctrl Pts',(4.60153519090348,-4.74142157490775,-2.82519003332091));
#79462=CARTESIAN_POINT('Ctrl Pts',(4.72080116332065,-0.189117622405927,
-5.51606850938893));
#79463=CARTESIAN_POINT('Ctrl Pts',(4.84006713573782,4.53679300913506,-3.1432922975186));
#79464=CARTESIAN_POINT('Ctrl Pts',(4.95933310815498,5.09800678279429,2.11497142249248));
#79465=CARTESIAN_POINT('Ctrl Pts',(5.07859908057215,0.979339242271404,5.43172826307833));
#79466=CARTESIAN_POINT('Ctrl Pts',(5.1978650529893,-4.03834464236845,3.76225329089237));
#79467=CARTESIAN_POINT('Ctrl Pts',(5.31713102540649,-5.3488985765674,-1.36090458628507));
#79468=CARTESIAN_POINT('Ctrl Pts',(5.43639699782363,-1.74925690561014,-5.234775788279));
#79469=CARTESIAN_POINT('Ctrl Pts',(5.55566297024081,3.45617209656404,-4.3032141143927));
#79470=CARTESIAN_POINT('Ctrl Pts',(5.67492894265797,5.48889539189286,0.578623065763662));
#79471=CARTESIAN_POINT('Ctrl Pts',(5.79419491507513,2.48290844722863,4.92929436309676));
#79472=CARTESIAN_POINT('Ctrl Pts',(5.9134608874923,-2.8023451485171,4.75495940508004));
#79473=CARTESIAN_POINT('Ctrl Pts',(6.03272685990946,-5.51509477257414,0.215654642662343));
#79474=CARTESIAN_POINT('Ctrl Pts',(6.15199283232664,-3.16508358210627,-4.52161732056773));
#79475=CARTESIAN_POINT('Ctrl Pts',(6.27125880474377,2.09041913570026,-5.10812344334733));
#79476=CARTESIAN_POINT('Ctrl Pts',(6.39052477716097,5.42695354514956,-1.00546133399804));
#79477=CARTESIAN_POINT('Ctrl Pts',(6.50979074957811,3.78163924961165,4.0201967440877));
#79478=CARTESIAN_POINT('Ctrl Pts',(6.62905672199529,-1.33515392291886,5.35538432584356));
#79479=CARTESIAN_POINT('Ctrl Pts',(6.74832269441244,-5.22629908012832,1.77442249772322));
#79480=CARTESIAN_POINT('Ctrl Pts',(6.86758866682961,-4.31979283170086,-3.4354282362702));
#79481=CARTESIAN_POINT('Ctrl Pts',(6.98685463924679,0.552207896342436,-5.49161576538213));
#79482=CARTESIAN_POINT('Ctrl Pts',(7.10612061166394,4.91729140639404,-2.50659579908286));
#79483=CARTESIAN_POINT('Ctrl Pts',(7.22538658408111,4.76838716600991,2.77943539417787));
#79484=CARTESIAN_POINT('Ctrl Pts',(7.34465255649827,0.242186670879671,5.5139933706729));
#79485=CARTESIAN_POINT('Ctrl Pts',(7.46391852891544,-4.50633696423125,3.18680160037922));
#79486=CARTESIAN_POINT('Ctrl Pts',(7.5831845013326,-5.11812185950969,-2.06581845925188));
#79487=CARTESIAN_POINT('Ctrl Pts',(7.70245047374978,-1.03156015100075,-5.42205320245419));
#79488=CARTESIAN_POINT('Ctrl Pts',(7.82171644616692,4.0019557850734,-3.80093766979861));
#79489=CARTESIAN_POINT('Ctrl Pts',(7.94098241858411,5.36174610705912,1.30937235300469));
#79490=CARTESIAN_POINT('Ctrl Pts',(8.06024839100124,1.79954701496616,5.21770139202147));
#79491=CARTESIAN_POINT('Ctrl Pts',(8.17951436341844,-3.41460485164159,4.33627155313435));
#79492=CARTESIAN_POINT('Ctrl Pts',(8.29878033583558,-5.49420901728412,-0.525779944245337));
#79493=CARTESIAN_POINT('Ctrl Pts',(8.41804630825275,-2.53022512749731,-4.90517462273849));
#79494=CARTESIAN_POINT('Ctrl Pts',(8.53731228066992,2.75646130062513,-4.78170454686741));
#79495=CARTESIAN_POINT('Ctrl Pts',(8.65657825308707,5.51276432918079,-0.268713092886506));
#79496=CARTESIAN_POINT('Ctrl Pts',(8.77584422550425,3.2084458496022,4.49095229384002));
#79497=CARTESIAN_POINT('Ctrl Pts',(8.8951101979214,-2.04116996261123,5.12800179983491));
#79498=CARTESIAN_POINT('Ctrl Pts',(9.01437617033858,-5.41702734842686,1.05763508913624));
#79499=CARTESIAN_POINT('Ctrl Pts',(9.13364214275574,-3.82014810472759,-3.98362218757285));
#79500=CARTESIAN_POINT('Ctrl Pts',(9.2529081151729,1.28356047334216,-5.36798377294959));
#79501=CARTESIAN_POINT('Ctrl Pts',(9.37217408759007,5.20898292298034,-1.82462987574903));
#79502=CARTESIAN_POINT('Ctrl Pts',(9.49144006000723,4.35264989723879,3.39370242470428));
#79503=CARTESIAN_POINT('Ctrl Pts',(9.61070603242441,-0.499339821234622,
5.49667508756937));
#79504=CARTESIAN_POINT('Ctrl Pts',(9.72997200484156,-4.89294429261305,2.55379588549317));
#79505=CARTESIAN_POINT('Ctrl Pts',(9.84923797725873,-4.79491123937786,-2.73342339967016));
#79506=CARTESIAN_POINT('Ctrl Pts',(9.96850394967589,-0.295233294641205,
-5.51140767654798));
#79507=CARTESIAN_POINT('Ctrl Pts',(10.0877699220931,4.47546366552298,-3.2300158287476));
#79508=CARTESIAN_POINT('Ctrl Pts',(10.2070358945102,5.13776303561924,2.01647421634918));
#79509=CARTESIAN_POINT('Ctrl Pts',(10.3263018669274,1.08368554481396,5.41187609940749));
#79510=CARTESIAN_POINT('Ctrl Pts',(10.4455678393446,-3.96519637597766,3.83927010970967));
#79511=CARTESIAN_POINT('Ctrl Pts',(10.5648338117617,-5.37409717912364,-1.25771888143246));
#79512=CARTESIAN_POINT('Ctrl Pts',(10.6840997841789,-1.84967049944617,-5.20014387482263));
#79513=CARTESIAN_POINT('Ctrl Pts',(10.803365756596,3.3727214393139,-4.36892748488331));
#79514=CARTESIAN_POINT('Ctrl Pts',(10.9226317290132,5.49901391915264,0.472888139354224));
#79515=CARTESIAN_POINT('Ctrl Pts',(11.0418977014304,2.57730752744729,4.88060069912919));
#79516=CARTESIAN_POINT('Ctrl Pts',(11.1611636738475,-2.71032222460136,4.80800693782864));
#79517=CARTESIAN_POINT('Ctrl Pts',(11.2804296462647,-5.5099234441787,0.321746662246017));
#79518=CARTESIAN_POINT('Ctrl Pts',(11.3996956186819,-3.25151103850694,-4.4598714378157));
#79519=CARTESIAN_POINT('Ctrl Pts',(11.518961591099,1.99173179213046,-5.14740534090655));
#79520=CARTESIAN_POINT('Ctrl Pts',(11.6382275635162,5.40659957463875,-1.10971091501));
#79521=CARTESIAN_POINT('Ctrl Pts',(11.7574935359333,3.85830324210287,3.94667877681414));
#79522=CARTESIAN_POINT('Ctrl Pts',(11.8767595083505,-1.23184817546466,5.38008618406631));
#79523=CARTESIAN_POINT('Ctrl Pts',(11.9960254807677,-5.1911844521573,1.87466830640958));
#79524=CARTESIAN_POINT('Ctrl Pts',(12.1152914531849,-4.38510393926939,-3.35166238114473));
#79525=CARTESIAN_POINT('Ctrl Pts',(12.234557425602,0.446425510915778,-5.50122545789394));
#79526=CARTESIAN_POINT('Ctrl Pts',(12.3538233980192,4.86814412802,-2.6007595091051));
#79527=CARTESIAN_POINT('Ctrl Pts',(12.4730893704363,4.82099133907667,2.68715831017164));
#79528=CARTESIAN_POINT('Ctrl Pts',(12.5923553428535,0.348252581961536,5.50831166643045));
#79529=CARTESIAN_POINT('Ctrl Pts',(12.7116213152707,-4.44417597165164,3.2729309813026));
#79530=CARTESIAN_POINT('Ctrl Pts',(12.8308872876878,-5.15692849249391,-1.96694326270007));
#79531=CARTESIAN_POINT('Ctrl Pts',(12.950153260105,-1.13571059728118,-5.40119789626338));
#79532=CARTESIAN_POINT('Ctrl Pts',(13.0694192325222,3.92806981873332,-3.87724706132231));
#79533=CARTESIAN_POINT('Ctrl Pts',(13.1886852049393,5.38595064914221,1.20594895430169));
#79534=CARTESIAN_POINT('Ctrl Pts',(13.3079511773565,1.89962271798245,5.18210486237994));
#79535=CARTESIAN_POINT('Ctrl Pts',(13.4272171497737,-3.33052573767825,4.40117888593941));
#79536=CARTESIAN_POINT('Ctrl Pts',(13.5464831221908,-5.50330965259982,-0.419952548484216));
#79537=CARTESIAN_POINT('Ctrl Pts',(13.665749094608,-2.62415128759299,-4.85557486763419));
#79538=CARTESIAN_POINT('Ctrl Pts',(13.7850150670251,2.66393219258639,-4.8338641425549));
#79539=CARTESIAN_POINT('Ctrl Pts',(13.9042810394423,5.50657238061311,-0.374750440220661));
#79540=CARTESIAN_POINT('Ctrl Pts',(14.0235470118595,3.29427516129926,4.42837763035443));
#79541=CARTESIAN_POINT('Ctrl Pts',(14.1428129842767,-1.94210920187053,5.16633226993638));
#79542=CARTESIAN_POINT('Ctrl Pts',(14.2620789566938,-5.39567118932092,1.16168398977903));
#79543=CARTESIAN_POINT('Ctrl Pts',(14.381344929111,-3.89610112885092,-3.90936993250106));
#79544=CARTESIAN_POINT('Ctrl Pts',(14.5006109015281,1.1800218174666,-5.39169043859891));
#79545=CARTESIAN_POINT('Ctrl Pts',(14.6198768739453,5.17290531566747,-1.92453315651251));
#79546=CARTESIAN_POINT('Ctrl Pts',(14.7391428463625,4.41715195278582,3.30931199819195));
#79547=CARTESIAN_POINT('Ctrl Pts',(14.8584088187797,-0.393469864863733,
5.5052664550247));
#79548=CARTESIAN_POINT('Ctrl Pts',(14.9776747911968,-4.84289320892863,2.64748232143101));
#79549=CARTESIAN_POINT('Ctrl Pts',(15.096940763614,-4.84662505027999,-2.64064440949086));
#79550=CARTESIAN_POINT('Ctrl Pts',(15.2162067360311,-0.401239623642889,
-5.50470562698815));
#79551=CARTESIAN_POINT('Ctrl Pts',(15.3354727084483,4.41247677962867,-3.31554308441536));
#79552=CARTESIAN_POINT('Ctrl Pts',(15.4547386808655,5.17561645555266,1.91723018450819));
#79553=CARTESIAN_POINT('Ctrl Pts',(15.5740046532826,1.18763049126349,5.39001958174527));
#79554=CARTESIAN_POINT('Ctrl Pts',(15.6932706256998,-3.89057955098784,3.91486500824893));
#79555=CARTESIAN_POINT('Ctrl Pts',(15.812536598117,-5.39730541957021,-1.15406736512861));
#79556=CARTESIAN_POINT('Ctrl Pts',(15.9318025705341,-1.94939904536532,-5.16358602497382));
#79557=CARTESIAN_POINT('Ctrl Pts',(16.0510685429513,3.28802165374775,-4.43302277005912));
#79558=CARTESIAN_POINT('Ctrl Pts',(16.1703345153684,5.50709581987209,0.366978073083481));
#79559=CARTESIAN_POINT('Ctrl Pts',(16.2896004877856,2.67075207054522,4.83009944546223));
#79560=CARTESIAN_POINT('Ctrl Pts',(16.4088664602028,-2.61729549995758,4.85927376685843));
#79561=CARTESIAN_POINT('Ctrl Pts',(16.5281324326199,-5.50271144876792,0.42771951904863));
#79562=CARTESIAN_POINT('Ctrl Pts',(16.6473984050371,-3.3367342583345,-4.39647378755214));
#79563=CARTESIAN_POINT('Ctrl Pts',(16.7666643774543,1.89230678652,-5.18478083442946));
#79564=CARTESIAN_POINT('Ctrl Pts',(16.8859303498714,5.38424320436169,-1.21354950111718));
#79565=CARTESIAN_POINT('Ctrl Pts',(17.0051963222886,3.93353826516432,3.87169910915921));
#79566=CARTESIAN_POINT('Ctrl Pts',(17.1244622947058,-1.12808619808918,5.40279546207863));
#79567=CARTESIAN_POINT('Ctrl Pts',(17.2437282671229,-5.1541472060249,1.97421980893783));
#79568=CARTESIAN_POINT('Ctrl Pts',(17.3629942395401,-4.44879097037678,-3.26665519718109));
#79569=CARTESIAN_POINT('Ctrl Pts',(17.4822602119573,0.340477786383454,-5.50879770479514));
#79570=CARTESIAN_POINT('Ctrl Pts',(17.6015261843744,4.81719387338903,-2.69395999628055));
#79571=CARTESIAN_POINT('Ctrl Pts',(17.7207921567916,4.87180999949389,2.59388600447428));
#79572=CARTESIAN_POINT('Ctrl Pts',(17.8400581292088,0.454189513473253,5.50058989211409));
#79573=CARTESIAN_POINT('Ctrl Pts',(17.9593241016259,-4.38036902456705,3.35784819251709));
#79574=CARTESIAN_POINT('Ctrl Pts',(18.0785900740431,-5.19382519442694,-1.86733958484043));
#79575=CARTESIAN_POINT('Ctrl Pts',(18.1978560464602,-1.23944041935899,-5.37834219088336));
#79576=CARTESIAN_POINT('Ctrl Pts',(18.3171220188774,3.85272904406541,-3.95212046734302));
#79577=CARTESIAN_POINT('Ctrl Pts',(18.4363879912946,5.40816043903902,1.10207891776834));
#79578=CARTESIAN_POINT('Ctrl Pts',(18.5556539637117,1.99899487267145,5.14458907731317));
#79579=CARTESIAN_POINT('Ctrl Pts',(18.6749199361289,-3.24521312308923,4.46445618873186));
#79580=CARTESIAN_POINT('Ctrl Pts',(18.7941859085461,-5.51037207039808,-0.313969618200402));
#79581=CARTESIAN_POINT('Ctrl Pts',(18.9134518809632,-2.71710556141284,-4.80417679145097));
#79582=CARTESIAN_POINT('Ctrl Pts',(19.0327178533804,2.5704164649311,-4.88423345799399));
#79583=CARTESIAN_POINT('Ctrl Pts',(19.1519838257976,5.49834100613709,-0.480648994181217));
#79584=CARTESIAN_POINT('Ctrl Pts',(19.2712497982147,3.37888439821132,4.36416286347117));
#79585=CARTESIAN_POINT('Ctrl Pts',(19.3905157706319,-1.84232915741783,5.2027493261837));
#79586=CARTESIAN_POINT('Ctrl Pts',(19.5097817430491,-5.37231667790874,1.26530264665799));
#79587=CARTESIAN_POINT('Ctrl Pts',(19.6290477154662,-3.97061118463848,-3.83366979483112));
#79588=CARTESIAN_POINT('Ctrl Pts',(19.7483136878834,1.07604612619046,-5.41340022626143));
#79589=CARTESIAN_POINT('Ctrl Pts',(19.8675796603005,5.13491186009314,-2.02372366306542));
#79590=CARTESIAN_POINT('Ctrl Pts',(19.9868456327177,4.48001806250103,3.22369592781969));
#79591=CARTESIAN_POINT('Ctrl Pts',(20.1061116051349,-0.287454182153403,
5.51181888023721));
#79592=CARTESIAN_POINT('Ctrl Pts',(20.2253775775521,-4.79104850097146,2.74018823016145));
#79593=CARTESIAN_POINT('Ctrl Pts',(20.3446435499692,-4.89654385477662,-2.54688742460792));
#79594=CARTESIAN_POINT('Ctrl Pts',(20.4639095223864,-0.507097348680508,
-5.49596484289502));
#79595=CARTESIAN_POINT('Ctrl Pts',(20.5831754948035,4.34785567940971,-3.39984238846463));
#79596=CARTESIAN_POINT('Ctrl Pts',(20.7024414672207,5.21155302312105,1.81727608320107));
#79597=CARTESIAN_POINT('Ctrl Pts',(20.8217074396379,1.29113558434761,5.3661668049184));
#79598=CARTESIAN_POINT('Ctrl Pts',(20.940973412055,-3.81452180264571,3.98900998902192));
#79599=CARTESIAN_POINT('Ctrl Pts',(21.0602393844722,-5.41851470245351,-1.04998842597045));
#79600=CARTESIAN_POINT('Ctrl Pts',(21.1795053568893,-2.04840560769031,-5.1251157783761));
#79601=CARTESIAN_POINT('Ctrl Pts',(21.2987713293066,3.2021041094591,-4.49547623145327));
#79602=CARTESIAN_POINT('Ctrl Pts',(21.4180373017236,5.51313810082114,0.260932092029769));
#79603=CARTESIAN_POINT('Ctrl Pts',(21.5373032741409,2.76320746820189,4.77780930584825));
#79604=CARTESIAN_POINT('Ctrl Pts',(21.656569246558,-2.52329942816223,4.90874090487696));
#79605=CARTESIAN_POINT('Ctrl Pts',(21.7758352189752,-5.49346145739179,0.533533964736603));
#79606=CARTESIAN_POINT('Ctrl Pts',(21.8951011913923,-3.42072167813528,-4.33144784986639));
#79607=CARTESIAN_POINT('Ctrl Pts',(22.0143671638096,1.79218094212641,-5.22023608144834));
#79608=CARTESIAN_POINT('Ctrl Pts',(22.1336331362266,5.35989271427127,-1.31693863443915));
#79609=CARTESIAN_POINT('Ctrl Pts',(22.2528991086439,4.00731645459238,3.79528551075277));
#79610=CARTESIAN_POINT('Ctrl Pts',(22.372165081061,-1.02390642029995,5.42350374922381));
#79611=CARTESIAN_POINT('Ctrl Pts',(22.4914310534782,-5.11520105892454,2.07304013520094));
#79612=CARTESIAN_POINT('Ctrl Pts',(22.6106970258953,-4.51083033775836,-3.18043816782147));
#79613=CARTESIAN_POINT('Ctrl Pts',(22.7299629983125,0.234403961770981,-5.51432970161217));
#79614=CARTESIAN_POINT('Ctrl Pts',(22.8492289707297,4.76445951254608,-2.7861627426778));
#79615=CARTESIAN_POINT('Ctrl Pts',(22.9684949431468,4.92082432595416,2.49965302161611));
#79616=CARTESIAN_POINT('Ctrl Pts',(23.087760915564,0.559958230386614,5.4908309075766));
#79617=CARTESIAN_POINT('Ctrl Pts',(23.2070268879812,-4.31493975465448,3.44152178390302));
#79618=CARTESIAN_POINT('Ctrl Pts',(23.3262928603983,-5.22879830016766,-1.76704431510376));
#79619=CARTESIAN_POINT('Ctrl Pts',(23.4455588328155,-1.34271119963572,-5.35349455120195));
#79620=CARTESIAN_POINT('Ctrl Pts',(23.5648248052326,3.77596136443968,-4.02553015758615));
#79621=CARTESIAN_POINT('Ctrl Pts',(23.6840907776498,5.42836725108453,0.997800712933093));
#79622=CARTESIAN_POINT('Ctrl Pts',(23.803356750067,2.09762667534973,5.10516793124745));
#79623=CARTESIAN_POINT('Ctrl Pts',(23.9226227224841,-3.15869860443647,4.52608002599466));
#79624=CARTESIAN_POINT('Ctrl Pts',(24.0418886949013,-5.51539365502694,-0.207870405458184));
#79625=CARTESIAN_POINT('Ctrl Pts',(24.1611546673185,-2.80905352221347,-4.75099943009008));
#79626=CARTESIAN_POINT('Ctrl Pts',(24.2804206397356,2.47594875234367,-4.93279383829738));
#79627=CARTESIAN_POINT('Ctrl Pts',(24.3996866121528,5.48807325434234,-0.586369533953697));
#79628=CARTESIAN_POINT('Ctrl Pts',(24.51895258457,3.46224222428067,4.29833177590844));
#79629=CARTESIAN_POINT('Ctrl Pts',(24.6382185569871,-1.74186678400333,5.23723948107804));
#79630=CARTESIAN_POINT('Ctrl Pts',(24.7574845294043,-5.34697246381719,1.36845268334623));
#79631=CARTESIAN_POINT('Ctrl Pts',(24.8767505018215,-4.04365067638685,-3.75654981102771));
#79632=CARTESIAN_POINT('Ctrl Pts',(24.9960164742386,0.971671908172561,-5.43310509545365));
#79633=CARTESIAN_POINT('Ctrl Pts',(25.1152824466558,5.09501662759478,-2.12216465900021));
#79634=CARTESIAN_POINT('Ctrl Pts',(25.234548419073,4.54122494315783,3.13688592253812));
#79635=CARTESIAN_POINT('Ctrl Pts',(25.3538143914901,-0.181332037298062,
5.5163299364365));
#79636=CARTESIAN_POINT('Ctrl Pts',(25.4730803639073,-4.73742937005836,2.8318792769264));
#79637=CARTESIAN_POINT('Ctrl Pts',(25.5923463363244,-4.94464916483277,-2.45218716905851));
#79638=CARTESIAN_POINT('Ctrl Pts',(25.7116123087416,-0.612767264061086,
-5.48518856152378));
#79639=CARTESIAN_POINT('Ctrl Pts',(25.8308782811588,4.2816242980748,-3.48288251962541));
#79640=CARTESIAN_POINT('Ctrl Pts',(25.9501442535759,5.24555942878053,1.71664893164223));
#79641=CARTESIAN_POINT('Ctrl Pts',(26.0694102259931,1.39416248969908,5.34032660309201));
#79642=CARTESIAN_POINT('Ctrl Pts',(26.1886761984103,-3.73705129986135,4.06167759153547));
#79643=CARTESIAN_POINT('Ctrl Pts',(26.3079421708274,-5.43771717265829,-0.945520610856157));
#79644=CARTESIAN_POINT('Ctrl Pts',(26.4272081432446,-2.14665351813937,-5.08474738295189));
#79645=CARTESIAN_POINT('Ctrl Pts',(26.5464741156617,3.1150006270531,-4.55626473866868));
#79646=CARTESIAN_POINT('Ctrl Pts',(26.6657400880789,5.51713852416773,0.154789471609084));
#79647=CARTESIAN_POINT('Ctrl Pts',(26.7850060604961,2.8546394784388,4.72374964657473));
#79648=CARTESIAN_POINT('Ctrl Pts',(26.9042720329133,-2.42836882180111,4.95639003112961));
#79649=CARTESIAN_POINT('Ctrl Pts',(27.0235380053304,-5.4821768958969,0.639150809645876));
#79650=CARTESIAN_POINT('Ctrl Pts',(27.1428039777476,-3.50344219214909,-4.26481770790332));
#79651=CARTESIAN_POINT('Ctrl Pts',(27.2620699501647,1.69139134177108,-5.2537579506824));
#79652=CARTESIAN_POINT('Ctrl Pts',(27.3813359225819,5.33355712286708,-1.41984002355569));
#79653=CARTESIAN_POINT('Ctrl Pts',(27.5006018949991,4.07961048573915,3.7174662822981));
#79654=CARTESIAN_POINT('Ctrl Pts',(27.6198678674162,-0.919347426341828,
5.44220337593657));
#79655=CARTESIAN_POINT('Ctrl Pts',(27.7391338398334,-5.07436043503451,2.17109268589186));
#79656=CARTESIAN_POINT('Ctrl Pts',(27.8583998122506,-4.57119906438141,-3.0930432245888));
#79657=CARTESIAN_POINT('Ctrl Pts',(27.9776657846677,0.128243322806431,-5.51781939950306));
#79658=CARTESIAN_POINT('Ctrl Pts',(28.0969317570849,4.7099605763017,-2.8773335998908));
#79659=CARTESIAN_POINT('Ctrl Pts',(28.2161977295021,4.96801616540672,2.40449426192572));
#79660=CARTESIAN_POINT('Ctrl Pts',(28.3354637019192,0.665519559973907,5.47903832717648));
#79661=CARTESIAN_POINT('Ctrl Pts',(28.4547296743364,-4.24791239443814,3.52392076593041));
#79662=CARTESIAN_POINT('Ctrl Pts',(28.5739956467536,-5.26183485700175,-1.66609459906019));
#79663=CARTESIAN_POINT('Ctrl Pts',(28.6932616191707,-1.44548469052482,-5.32666417984418));
#79664=CARTESIAN_POINT('Ctrl Pts',(28.8125275915879,3.69779521169796,-4.09744894388208));
#79665=CARTESIAN_POINT('Ctrl Pts',(28.931793564005,5.44656360144046,0.893152960494481));
#79666=CARTESIAN_POINT('Ctrl Pts',(29.0510595364223,2.1954815965324,5.06385602428271));
#79667=CARTESIAN_POINT('Ctrl Pts',(29.1703255088393,-3.07101422342191,4.58602757459188));
#79668=CARTESIAN_POINT('Ctrl Pts',(29.2895914812566,-5.51837254668137,-0.10169420538848));
#79669=CARTESIAN_POINT('Ctrl Pts',(29.4088574536737,-2.89996111595197,-4.69606247843269));
#79670=CARTESIAN_POINT('Ctrl Pts',(29.5281234260909,2.38056404208793,-4.97952729853896));
#79671=CARTESIAN_POINT('Ctrl Pts',(29.6473893985081,5.47577292801507,-0.691872904653279));
#79672=CARTESIAN_POINT('Ctrl Pts',(29.7666553709252,3.54431776692506,4.23090874900843));
#79673=CARTESIAN_POINT('Ctrl Pts',(29.8859213433424,-1.64075928908623,5.26978996077206));
#79674=CARTESIAN_POINT('Ctrl Pts',(30.0051873157595,-5.31964793358328,1.4710958969759));
#79675=CARTESIAN_POINT('Ctrl Pts',(30.1244532881768,-4.11519255303412,-3.67803854341268));
#79676=CARTESIAN_POINT('Ctrl Pts',(30.2437192605938,0.866937819671528,-5.45079774823832));
#79677=CARTESIAN_POINT('Ctrl Pts',(30.3629852330111,5.0532343938558,-2.21981968549902));
#79678=CARTESIAN_POINT('Ctrl Pts',(30.4822512054281,4.60074992604512,3.0489141334863));
#79679=CARTESIAN_POINT('Ctrl Pts',(30.6015171778454,-0.0751427339222241,
5.51879795289839));
#79680=CARTESIAN_POINT('Ctrl Pts',(30.7207831502625,-4.68205567468513,2.92252150283363));
#79681=CARTESIAN_POINT('Ctrl Pts',(30.8400491226797,-4.99092316406302,-2.35657871623164));
#79682=CARTESIAN_POINT('Ctrl Pts',(30.9593150950968,-0.718210233648821,
-5.47238077400128));
#79683=CARTESIAN_POINT('Ctrl Pts',(31.078581067514,4.21380716521979,-3.56463272297702));
#79684=CARTESIAN_POINT('Ctrl Pts',(31.1978470399312,5.27762307784604,1.61538599831857));
#79685=CARTESIAN_POINT('Ctrl Pts',(31.3171130123484,1.496673050053,5.31250854649871));
#79686=CARTESIAN_POINT('Ctrl Pts',(31.4363789847655,-3.65819673477567,4.13284090246077));
#79687=CARTESIAN_POINT('Ctrl Pts',(31.5556449571827,-5.45490571831667,-0.840702610708948));
#79688=CARTESIAN_POINT('Ctrl Pts',(31.6749109295998,-2.24410638940634,-5.04249578962663));
#79689=CARTESIAN_POINT('Ctrl Pts',(31.794176902017,3.02674346636162,-4.61536577794365));
#79690=CARTESIAN_POINT('Ctrl Pts',(31.9134428744342,5.51909560830654,0.0485895230291355));
#79691=CARTESIAN_POINT('Ctrl Pts',(32.0327088468513,2.94501423830122,4.66794048929288));
#79692=CARTESIAN_POINT('Ctrl Pts',(32.1519748192685,-2.3325388395765,5.0022034981839));
#79693=CARTESIAN_POINT('Ctrl Pts',(32.2712407916856,-5.46886194365754,0.744530937296086));
#79694=CARTESIAN_POINT('Ctrl Pts',(32.3905067641028,-3.58486516382964,-4.19660803894495));
#79695=CARTESIAN_POINT('Ctrl Pts',(32.50977273652,1.5899753141059,-5.28533402690029));
#79696=CARTESIAN_POINT('Ctrl Pts',(32.6290387089371,5.305246183855,-1.52221555768843));
#79697=CARTESIAN_POINT('Ctrl Pts',(32.7483046813544,4.15039358363284,3.63827024509121));
#79698=CARTESIAN_POINT('Ctrl Pts',(32.8675706537714,-0.814447940907383,
5.45888741658297));
#79699=CARTESIAN_POINT('Ctrl Pts',(32.9868366261887,-5.03164046017552,2.26834114605837));
#79700=CARTESIAN_POINT('Ctrl Pts',(33.1061025986057,-4.62987479195544,-3.00450273526126));
#79701=CARTESIAN_POINT('Ctrl Pts',(33.2253685710231,0.0220351873710713,
-5.5192655060156));
#79702=CARTESIAN_POINT('Ctrl Pts',(33.34463454344,4.65371724899836,-2.96743880168604));
#79703=CARTESIAN_POINT('Ctrl Pts',(33.4639005158574,5.01336803978119,2.30844496860492));
#79704=CARTESIAN_POINT('Ctrl Pts',(33.5831664882744,0.770834406315328,5.46521651843883));
#79705=CARTESIAN_POINT('Ctrl Pts',(33.7024324606917,-4.17931176831432,3.6050146211362));
#79706=CARTESIAN_POINT('Ctrl Pts',(33.8216984331088,-5.29292262943967,-1.56452782466247));
#79707=CARTESIAN_POINT('Ctrl Pts',(33.9409644055259,-1.54772282861625,-5.29786101376356));
#79708=CARTESIAN_POINT('Ctrl Pts',(34.0602303779431,3.6182595356233,-4.16785019023544));
#79709=CARTESIAN_POINT('Ctrl Pts',(34.1794963503603,5.4627427508684,0.788174418017909));
#79710=CARTESIAN_POINT('Ctrl Pts',(34.2987623227774,2.29252339446042,5.0206686567849));
#79711=CARTESIAN_POINT('Ctrl Pts',(34.4180282951946,-2.98219245501818,4.64427663222141));
#79712=CARTESIAN_POINT('Ctrl Pts',(34.5372942676118,-5.51930764209687,0.00451965836400682));
#79713=CARTESIAN_POINT('Ctrl Pts',(34.656560240029,-2.98979467388986,-4.63938628304514));
#79714=CARTESIAN_POINT('Ctrl Pts',(34.7758262124461,2.28429766103466,-5.02441653041523));
#79715=CARTESIAN_POINT('Ctrl Pts',(34.8950921848632,5.46144458275793,-0.797120031824677));
#79716=CARTESIAN_POINT('Ctrl Pts',(35.0143581572805,3.62508062841914,4.16191875370487));
#79717=CARTESIAN_POINT('Ctrl Pts',(35.1336241296976,-1.53904411895615,5.30038870980534));
#79718=CARTESIAN_POINT('Ctrl Pts',(35.2528901021148,-5.29035320736527,1.57319427237781));
#79719=CARTESIAN_POINT('Ctrl Pts',(35.3721560745319,-4.18521031782329,-3.59816506956947));
#79720=CARTESIAN_POINT('Ctrl Pts',(35.4914220469491,0.76188264955475,-5.46647163195967));
#79721=CARTESIAN_POINT('Ctrl Pts',(35.6106880193662,5.0095806347121,-2.31665257477511));
#79722=CARTESIAN_POINT('Ctrl Pts',(35.7299539917834,4.65857096293502,2.95981314196468));
#79723=CARTESIAN_POINT('Ctrl Pts',(35.8492199642006,0.0310744040885409,
5.51922201578924));
#79724=CARTESIAN_POINT('Ctrl Pts',(35.9684859366178,-4.6249479319303,3.01208133700502));
#79725=CARTESIAN_POINT('Ctrl Pts',(36.0877519090349,-5.03534869769585,-2.2600974750615));
#79726=CARTESIAN_POINT('Ctrl Pts',(36.2070178814521,-0.82338723695312,-5.45754622539771));
#79727=CARTESIAN_POINT('Ctrl Pts',(36.3262838538693,4.14442945774543,-3.64506271839436));
#79728=CARTESIAN_POINT('Ctrl Pts',(36.4455498262864,5.30773198119607,1.51352478159224));
#79729=CARTESIAN_POINT('Ctrl Pts',(36.5648157987036,1.59862951581808,5.28272294851769));
#79730=CARTESIAN_POINT('Ctrl Pts',(36.6840817711207,-3.57798772320569,4.20247354542357));
#79731=CARTESIAN_POINT('Ctrl Pts',(36.803347743538,-5.47007319271275,-0.735573207822807));
#79732=CARTESIAN_POINT('Ctrl Pts',(36.922613715955,-2.34072961144035,-4.99837671957824));
#79733=CARTESIAN_POINT('Ctrl Pts',(37.0418796883723,2.93736813071235,-4.67275732224894));
#79734=CARTESIAN_POINT('Ctrl Pts',(37.1611456607894,5.51900327969889,-0.057628683827517));
#79735=CARTESIAN_POINT('Ctrl Pts',(37.2804116332065,3.03430843495129,4.61040300226366));
#79736=CARTESIAN_POINT('Ctrl Pts',(37.3996776056238,-2.2358642669444,5.0461633913799));
#79737=CARTESIAN_POINT('Ctrl Pts',(37.5189435780408,-5.45348488848064,0.849637117637928));
#79738=CARTESIAN_POINT('Ctrl Pts',(37.6382095504581,-3.66503003262188,-4.12684752159054));
#79739=CARTESIAN_POINT('Ctrl Pts',(37.7574755228752,1.48810259966544,-5.31494612688231));
#79740=CARTESIAN_POINT('Ctrl Pts',(37.8767414952924,5.27471933483358,-1.62403964590353));
#79741=CARTESIAN_POINT('Ctrl Pts',(37.9960074677095,4.22011637573384,3.55775015176621));
#79742=CARTESIAN_POINT('Ctrl Pts',(38.1152734401267,-0.710152797904622,
5.47350509862131));
#79743=CARTESIAN_POINT('Ctrl Pts',(38.2345394125439,-4.9853333920201,2.36483512966171));
#79744=CARTESIAN_POINT('Ctrl Pts',(38.353805384961,-4.69013369949273,-2.91502009518441));
#79745=CARTESIAN_POINT('Ctrl Pts',(38.4730713573783,-0.077709984764535,
-5.51827546323263));
#79746=CARTESIAN_POINT('Ctrl Pts',(38.5724596677258,3.80513849405293,-3.46787737060704));
#79747=CARTESIAN_POINT('Ctrl Pts',(38.651970316004,4.8393236171102,-0.417509269414375));
#79748=CARTESIAN_POINT('Ctrl Pts',(38.691725640143,4.58753946265277,1.15800627176077));
#79749=CARTESIAN_POINT('Ctrl Pts',(38.7116033022125,4.27611881062226,1.87009427887657));
#79750=CARTESIAN_POINT('Ctrl Pts',(-17.6184,2.62535040627071,-3.68399909158434));
#79751=CARTESIAN_POINT('Ctrl Pts',(-17.5985223379305,3.23883466326236,-3.24680811968291));
#79752=CARTESIAN_POINT('Ctrl Pts',(-17.5587670137914,4.23254591953354,-2.06184536971571));
#79753=CARTESIAN_POINT('Ctrl Pts',(-17.4792563655133,4.8909587174436,0.989874372427294));
#79754=CARTESIAN_POINT('Ctrl Pts',(-17.3798680551657,2.68243561037911,4.62805141939821));
#79755=CARTESIAN_POINT('Ctrl Pts',(-17.2606020827485,-2.44949610129593,
4.7591308229798));
#79756=CARTESIAN_POINT('Ctrl Pts',(-17.1413361103314,-5.32337982130319,
0.515004556339686));
#79757=CARTESIAN_POINT('Ctrl Pts',(-17.0220701379142,-3.31538769240887,
-4.19860974939619));
#79758=CARTESIAN_POINT('Ctrl Pts',(-16.902804165497,1.73863948785637,-5.05968774485838));
#79759=CARTESIAN_POINT('Ctrl Pts',(-16.7835381930798,5.19527552722027,-1.27515938975536));
#79760=CARTESIAN_POINT('Ctrl Pts',(-16.6642722206627,3.88345012932081,3.67946867571279));
#79761=CARTESIAN_POINT('Ctrl Pts',(-16.5450062482455,-0.993689040191803,
5.25665841728971));
#79762=CARTESIAN_POINT('Ctrl Pts',(-16.4257402758284,-4.95844193487295,
2.00819591524889));
#79763=CARTESIAN_POINT('Ctrl Pts',(-16.3064743034112,-4.37153537144703,
-3.08368617743557));
#79764=CARTESIAN_POINT('Ctrl Pts',(-16.187208330994,0.228419052524531,-5.34483459461538));
#79765=CARTESIAN_POINT('Ctrl Pts',(-16.0679423585769,4.61866000512981,-2.69949887735067));
#79766=CARTESIAN_POINT('Ctrl Pts',(-15.9486763861597,4.76906677072755,2.42391962238011));
#79767=CARTESIAN_POINT('Ctrl Pts',(-15.8294104137425,0.541545441910157,
5.32222750447519));
#79768=CARTESIAN_POINT('Ctrl Pts',(-15.7101444413254,-4.18310095899125,
3.33482055878733));
#79769=CARTESIAN_POINT('Ctrl Pts',(-15.5908784689082,-5.06773584614322,
-1.71389202338234));
#79770=CARTESIAN_POINT('Ctrl Pts',(-15.4716124964911,-1.30027644702517,
-5.18928239612476));
#79771=CARTESIAN_POINT('Ctrl Pts',(-15.3523465240739,3.66081343996144,-3.90100162460633));
#79772=CARTESIAN_POINT('Ctrl Pts',(-15.2330805516567,5.26134075862523,0.968330387076498));
#79773=CARTESIAN_POINT('Ctrl Pts',(-15.1138145792395,2.03204885203783,4.94875210508029));
#79774=CARTESIAN_POINT('Ctrl Pts',(-14.9945486068224,-3.06262837106116,
4.38630564025653));
#79775=CARTESIAN_POINT('Ctrl Pts',(-14.8752826344052,-5.34586621077957,
-0.202692870982978));
#79776=CARTESIAN_POINT('Ctrl Pts',(-14.7560166619881,-2.72169207944861,
-4.60562287829862));
#79777=CARTESIAN_POINT('Ctrl Pts',(-14.6367506895709,2.40094789974828,-4.78067139956327));
#79778=CARTESIAN_POINT('Ctrl Pts',(-14.5174847171537,5.31955958788271,-0.56714695851215));
#79779=CARTESIAN_POINT('Ctrl Pts',(-14.3982187447365,3.35490834716323,4.16700850147134));
#79780=CARTESIAN_POINT('Ctrl Pts',(-14.2789527723194,-1.68949024264872,
5.07592283106375));
#79781=CARTESIAN_POINT('Ctrl Pts',(-14.1596867999022,-5.18296625647794,
1.32522852967441));
#79782=CARTESIAN_POINT('Ctrl Pts',(-14.0404208274851,-3.91856964050138,
-3.6420024494952));
#79783=CARTESIAN_POINT('Ctrl Pts',(-13.9211548550679,0.943005562874773,
-5.26593869864046));
#79784=CARTESIAN_POINT('Ctrl Pts',(-13.8018888826508,4.93891810628447,-2.05583506379208));
#79785=CARTESIAN_POINT('Ctrl Pts',(-13.6826229102336,4.40098996586505,3.04148930462108));
#79786=CARTESIAN_POINT('Ctrl Pts',(-13.5633569378164,-0.176970207163579,
5.34677953683851));
#79787=CARTESIAN_POINT('Ctrl Pts',(-13.4440909653992,-4.59247481650836,
2.74381940542772));
#79788=CARTESIAN_POINT('Ctrl Pts',(-13.3248249929821,-4.79216763991698,
-2.37791908624871));
#79789=CARTESIAN_POINT('Ctrl Pts',(-13.2055590205649,-0.592734148285034,
-5.31676932913924));
#79790=CARTESIAN_POINT('Ctrl Pts',(-13.0862930481478,4.15081895382183,-3.37491805566053));
#79791=CARTESIAN_POINT('Ctrl Pts',(-12.9670270757306,5.08399264919423,1.66504913223642));
#79792=CARTESIAN_POINT('Ctrl Pts',(-12.8477611033134,1.35014976061496,5.17653025623679));
#79793=CARTESIAN_POINT('Ctrl Pts',(-12.7284951308963,-3.62310706075401,
3.93604688693356));
#79794=CARTESIAN_POINT('Ctrl Pts',(-12.6092291584791,-5.27041478960109,
-0.917658877458269));
#79795=CARTESIAN_POINT('Ctrl Pts',(-12.4899631860619,-2.07957366092086,
-4.92896979688741));
#79796=CARTESIAN_POINT('Ctrl Pts',(-12.3706972136447,3.02027981942101,-4.41557240708635));
#79797=CARTESIAN_POINT('Ctrl Pts',(-12.2514312412276,5.34756910110119,0.151243442078761));
#79798=CARTESIAN_POINT('Ctrl Pts',(-12.1321652688104,2.76588321291629,4.57922044919569));
#79799=CARTESIAN_POINT('Ctrl Pts',(-12.0128992963933,-2.35483522599469,
4.80355294841628));
#79800=CARTESIAN_POINT('Ctrl Pts',(-11.8936333239761,-5.31385599723994,
0.618307617954934));
#79801=CARTESIAN_POINT('Ctrl Pts',(-11.7743673515589,-3.39484963998713,
-4.13453332211792));
#79802=CARTESIAN_POINT('Ctrl Pts',(-11.6551013791418,1.64056947847539,-5.09194478133052));
#79803=CARTESIAN_POINT('Ctrl Pts',(-11.5358354067246,5.16997442825406,-1.37503973797965));
#79804=CARTESIAN_POINT('Ctrl Pts',(-11.4165694343074,3.95343302047925,3.60412780328452));
#79805=CARTESIAN_POINT('Ctrl Pts',(-11.2973034618903,-0.892290949753927,
5.2747688793739));
#79806=CARTESIAN_POINT('Ctrl Pts',(-11.1780374894731,-4.91890739022456,
2.10326411946247));
#79807=CARTESIAN_POINT('Ctrl Pts',(-11.058771517056,-4.43005263528682,-2.99900041987535));
#79808=CARTESIAN_POINT('Ctrl Pts',(-10.9395055446388,0.125513175958816,
-5.3482348782084));
#79809=CARTESIAN_POINT('Ctrl Pts',(-10.8202395722216,4.56586008070243,-2.78788299490349));
#79810=CARTESIAN_POINT('Ctrl Pts',(-10.7009735998044,4.81482706281336,2.3316968553018));
#79811=CARTESIAN_POINT('Ctrl Pts',(-10.5817076273873,0.643866774853417,
5.31081965858981));
#79812=CARTESIAN_POINT('Ctrl Pts',(-10.4624416549701,-4.11815198298316,
3.41470263930491));
#79813=CARTESIAN_POINT('Ctrl Pts',(-10.343175682553,-5.09977904358443,-1.61605184831468));
#79814=CARTESIAN_POINT('Ctrl Pts',(-10.2239097101358,-1.39989788550755,
-5.1632989241352));
#79815=CARTESIAN_POINT('Ctrl Pts',(-10.1046437377186,3.5850651163716,-3.97072763875836));
#79816=CARTESIAN_POINT('Ctrl Pts',(-9.98537776530147,5.27900086719687,0.866902367028086));
#79817=CARTESIAN_POINT('Ctrl Pts',(-9.86611179288431,2.12690589100833,4.90873111920161));
#79818=CARTESIAN_POINT('Ctrl Pts',(-9.74684582046714,-2.97765159855841,
4.44443031528525));
#79819=CARTESIAN_POINT('Ctrl Pts',(-9.62757984804998,-5.34877685275258,
-0.0997800044217893));
#79820=CARTESIAN_POINT('Ctrl Pts',(-9.50831387563282,-2.80981824212958,
-4.55239402029525));
#79821=CARTESIAN_POINT('Ctrl Pts',(-9.38904790321564,2.30850450978291,-4.82598972213328));
#79822=CARTESIAN_POINT('Ctrl Pts',(-9.26978193079849,5.30766038347549,-0.669411027328533));
#79823=CARTESIAN_POINT('Ctrl Pts',(-9.15051595838132,3.43447659405036,4.10167531561732));
#79824=CARTESIAN_POINT('Ctrl Pts',(-9.03124998596416,-1.59149680929566,
5.10749525460629));
#79825=CARTESIAN_POINT('Ctrl Pts',(-8.91198401354699,-5.15650389840683,
1.42472362777463));
#79826=CARTESIAN_POINT('Ctrl Pts',(-8.79271804112983,-3.98793034142981,
-3.56591944128407));
#79827=CARTESIAN_POINT('Ctrl Pts',(-8.67345206871266,0.841493716983345,
-5.28311065510666));
#79828=CARTESIAN_POINT('Ctrl Pts',(-8.55418609629549,4.8984412193819,-2.15049842829157));
#79829=CARTESIAN_POINT('Ctrl Pts',(-8.43492012387834,4.45870511426281,2.9562338496592));
#79830=CARTESIAN_POINT('Ctrl Pts',(-8.31565415146116,-0.0740445231469701,
5.3491950121879));
#79831=CARTESIAN_POINT('Ctrl Pts',(-8.19638817904401,-4.53882257969058,
2.83168844683082));
#79832=CARTESIAN_POINT('Ctrl Pts',(-8.07712220662684,-4.83704066797944,
-2.2852587263015));
#79833=CARTESIAN_POINT('Ctrl Pts',(-7.95785623420967,-0.694939784074152,
-5.30437824502882));
#79834=CARTESIAN_POINT('Ctrl Pts',(-7.83859026179251,4.08510370142725,-3.45417104648997));
#79835=CARTESIAN_POINT('Ctrl Pts',(-7.71932428937535,5.11509323577896,1.56690492982581));
#79836=CARTESIAN_POINT('Ctrl Pts',(-7.60005831695818,1.44951639010705,5.1495895083623));
#79837=CARTESIAN_POINT('Ctrl Pts',(-7.48079234454102,-3.54669122121178,
4.00504073028022));
#79838=CARTESIAN_POINT('Ctrl Pts',(-7.36152637212386,-5.28709814796872,
-0.816065587786831));
#79839=CARTESIAN_POINT('Ctrl Pts',(-7.24226039970668,-2.17404118518495,
-4.88803792895919));
#79840=CARTESIAN_POINT('Ctrl Pts',(-7.12299442728953,2.93474766896221,-4.4728767017821));
#79841=CARTESIAN_POINT('Ctrl Pts',(-7.00372845487236,5.34948934683475,0.0483073278670784));
#79842=CARTESIAN_POINT('Ctrl Pts',(-6.8844624824552,2.85349310274905,4.52514607304423));
#79843=CARTESIAN_POINT('Ctrl Pts',(-6.76519651003803,-2.26196004295795,
4.84797964454119));
#79844=CARTESIAN_POINT('Ctrl Pts',(-6.64593053762087,-5.30097331922578,
0.720452454142903));
#79845=CARTESIAN_POINT('Ctrl Pts',(-6.5266645652037,-3.47378554073058,-4.06843752401771));
#79846=CARTESIAN_POINT('Ctrl Pts',(-6.40739859278654,1.54227677916538,-5.12257281122204));
#79847=CARTESIAN_POINT('Ctrl Pts',(-6.28813262036938,5.14255591405802,-1.47427559859448));
#79848=CARTESIAN_POINT('Ctrl Pts',(-6.16886664795221,4.0220584092331,3.52738090125541));
#79849=CARTESIAN_POINT('Ctrl Pts',(-6.04960067553505,-0.790618568056538,
5.2909632534793));
#79850=CARTESIAN_POINT('Ctrl Pts',(-5.93033470311788,-4.87752148875202,
2.19753361671364));
#79851=CARTESIAN_POINT('Ctrl Pts',(-5.81106873070072,-4.48694474979491,
-2.91319355383608));
#79852=CARTESIAN_POINT('Ctrl Pts',(-5.69180275828355,0.0225690143544715,
-5.34965984987971));
#79853=CARTESIAN_POINT('Ctrl Pts',(-5.57253678586638,4.51136481694416,-2.87523170514354));
#79854=CARTESIAN_POINT('Ctrl Pts',(-5.45327081344922,4.85880639859978,2.23860899907733));
#79855=CARTESIAN_POINT('Ctrl Pts',(-5.33400484103205,0.745948446959714,
5.29744568488459));
#79856=CARTESIAN_POINT('Ctrl Pts',(-5.21473886861489,-4.05167716918246,
3.49331962272991));
#79857=CARTESIAN_POINT('Ctrl Pts',(-5.09547289619773,-5.12993380779606,
-1.51761292741435));
#79858=CARTESIAN_POINT('Ctrl Pts',(-4.97620692378056,-1.49900068010318,
-5.13540327830972));
#79859=CARTESIAN_POINT('Ctrl Pts',(-4.8569409513634,3.50798892841612,-4.03898298435808));
#79860=CARTESIAN_POINT('Ctrl Pts',(-4.73767497894623,5.29470588216781,0.765153246847895));
#79861=CARTESIAN_POINT('Ctrl Pts',(-4.61840900652908,2.22097517906763,4.86689214219808));
#79862=CARTESIAN_POINT('Ctrl Pts',(-4.4991430341119,-2.89157200322203,4.50090893264979));
#79863=CARTESIAN_POINT('Ctrl Pts',(-4.37987706169475,-5.34970651737601,
0.00316982159248442));
#79864=CARTESIAN_POINT('Ctrl Pts',(-4.26061108927757,-2.89690375080243,
-4.49747913040303));
#79865=CARTESIAN_POINT('Ctrl Pts',(-4.14134511686041,2.21520613519663,-4.86952067953422));
#79866=CARTESIAN_POINT('Ctrl Pts',(-4.02207914444325,5.29379542366406,-0.771427172335632));
#79867=CARTESIAN_POINT('Ctrl Pts',(-3.90281317202608,3.51277284030709,4.03482302489525));
#79868=CARTESIAN_POINT('Ctrl Pts',(-3.78354719960892,-1.49291394549895,
5.13717605510642));
#79869=CARTESIAN_POINT('Ctrl Pts',(-3.66428122719175,-5.12813176668884,
1.52369106228954));
#79870=CARTESIAN_POINT('Ctrl Pts',(-3.54501525477459,-4.05581406387994,
-3.48851575158515));
#79871=CARTESIAN_POINT('Ctrl Pts',(-3.42574928235742,0.73967021363975,-5.29832594739868));
#79872=CARTESIAN_POINT('Ctrl Pts',(-3.30648330994026,4.85615013534878,-2.24436532961465));
#79873=CARTESIAN_POINT('Ctrl Pts',(-3.18721733752309,4.51476892709962,2.86988351762224));
#79874=CARTESIAN_POINT('Ctrl Pts',(-3.06795136510593,0.0289085841635225,
5.34962934824326));
#79875=CARTESIAN_POINT('Ctrl Pts',(-2.94868539268877,-4.48348933485096,
2.91850873805477));
#79876=CARTESIAN_POINT('Ctrl Pts',(-2.8294194202716,-4.88012223932707,-2.19175199305243));
#79877=CARTESIAN_POINT('Ctrl Pts',(-2.71015344785444,-0.796888040481462,
-5.29002262006144));
#79878=CARTESIAN_POINT('Ctrl Pts',(-2.59088747543727,4.01787548130092,-3.53214474315326));
#79879=CARTESIAN_POINT('Ctrl Pts',(-2.4716215030201,5.1442993855074,1.46818040515877));
#79880=CARTESIAN_POINT('Ctrl Pts',(-2.35235553060294,1.54834617361307,5.12074154751847));
#79881=CARTESIAN_POINT('Ctrl Pts',(-2.23308955818578,-3.46896182153357,
4.07255125818778));
#79882=CARTESIAN_POINT('Ctrl Pts',(-2.11382358576862,-5.3018233653736,-0.714170058321242));
#79883=CARTESIAN_POINT('Ctrl Pts',(-1.99455761335145,-2.26770352691226,
-4.84529571686329));
#79884=CARTESIAN_POINT('Ctrl Pts',(-1.87529164093429,2.84812859908841,-4.52852441230905));
#79885=CARTESIAN_POINT('Ctrl Pts',(-1.75602566851712,5.3494283442679,-0.0546466775498073));
#79886=CARTESIAN_POINT('Ctrl Pts',(-1.63675969609995,2.94004616678162,4.46939575412793));
#79887=CARTESIAN_POINT('Ctrl Pts',(-1.51749372368279,-2.1682471155684,4.89061083257026));
#79888=CARTESIAN_POINT('Ctrl Pts',(-1.39822775126562,-5.28612736141081,
0.822330462021165));
#79889=CARTESIAN_POINT('Ctrl Pts',(-1.27896177884846,-3.55143488284157,
-4.00083493070636));
#79890=CARTESIAN_POINT('Ctrl Pts',(-1.1596958064313,1.4434128789333,-5.15130363410601));
#79891=CARTESIAN_POINT('Ctrl Pts',(-1.04042983401413,5.1132327918697,-1.57296544334973));
#79892=CARTESIAN_POINT('Ctrl Pts',(-0.921163861596969,4.08919417984387,
3.4493275909016));
#79893=CARTESIAN_POINT('Ctrl Pts',(-0.801897889179802,-0.688653371177603,
5.30519805513329));
#79894=CARTESIAN_POINT('Ctrl Pts',(-0.682631916762638,-4.83432913800304,
2.29098923072084));
#79895=CARTESIAN_POINT('Ctrl Pts',(-0.563365944345475,-4.54217506986187,
-2.82630775120993));
#79896=CARTESIAN_POINT('Ctrl Pts',(-0.444099971928309,-0.0803835059582494,
-5.3491035101028));
#79897=CARTESIAN_POINT('Ctrl Pts',(-0.324833999511145,4.45519871447649,
-2.9615155384281));
#79898=CARTESIAN_POINT('Ctrl Pts',(-0.205568027093979,4.90098621647057,
2.14469204684251));
#79899=CARTESIAN_POINT('Ctrl Pts',(-0.0863020546768169,0.847753848005954,
5.28210973788082));
#79900=CARTESIAN_POINT('Ctrl Pts',(0.0329639177403491,-3.98370176757143,
3.57064281283809));
#79901=CARTESIAN_POINT('Ctrl Pts',(0.152229890157513,-5.1581886387657,-1.41861194014872));
#79902=CARTESIAN_POINT('Ctrl Pts',(0.271495862574679,-1.59754830160526,
-5.10560567355749));
#79903=CARTESIAN_POINT('Ctrl Pts',(0.390761834991842,3.42961351418844,-4.10574244359289));
#79904=CARTESIAN_POINT('Ctrl Pts',(0.510027807409007,5.30844993855932,0.663120742876867));
#79905=CARTESIAN_POINT('Ctrl Pts',(0.629293779826171,2.3142219020159,4.82325065262569));
#79906=CARTESIAN_POINT('Ctrl Pts',(0.748559752243337,-2.80442147910245,
4.55572058376859));
#79907=CARTESIAN_POINT('Ctrl Pts',(0.867825724660504,-5.34865485326728,
0.106118473624908));
#79908=CARTESIAN_POINT('Ctrl Pts',(0.987091697077666,-2.98291635601472,
-4.44089854453399));
#79909=CARTESIAN_POINT('Ctrl Pts',(1.10635766949483,2.12108733213468,-4.91124815085553));
#79910=CARTESIAN_POINT('Ctrl Pts',(1.22562364191199,5.27796984247255,-0.873157609927544));
#79911=CARTESIAN_POINT('Ctrl Pts',(1.34488961432916,3.58976808851186,3.96647638849978));
#79912=CARTESIAN_POINT('Ctrl Pts',(1.46415558674632,-1.39377816290472,5.16495424011036));
#79913=CARTESIAN_POINT('Ctrl Pts',(1.58342155916349,-5.09786036913662,1.62209417932818));
#79914=CARTESIAN_POINT('Ctrl Pts',(1.70268753158065,-4.12219566637061,-3.40982004774148));
#79915=CARTESIAN_POINT('Ctrl Pts',(1.82195350399781,0.637572764456073,-5.31157894037619));
#79916=CARTESIAN_POINT('Ctrl Pts',(1.94121947641498,4.81206051717935,-2.33740100300047));
#79917=CARTESIAN_POINT('Ctrl Pts',(2.06048544883214,4.56916064047356,2.78247028939603));
#79918=CARTESIAN_POINT('Ctrl Pts',(2.17975142124932,0.13185098482894,5.34808238414702));
#79919=CARTESIAN_POINT('Ctrl Pts',(2.29901739366647,-4.42649557532506,3.00424812414882));
#79920=CARTESIAN_POINT('Ctrl Pts',(2.41828336608365,-4.92139639817879,-2.09743351785397));
#79921=CARTESIAN_POINT('Ctrl Pts',(2.5375493385008,-0.898541159731936,-5.27370777101761));
#79922=CARTESIAN_POINT('Ctrl Pts',(2.65681531091797,3.94915919222963,-3.60881026714515));
#79923=CARTESIAN_POINT('Ctrl Pts',(2.77608128333514,5.17160028152781,1.36891212206108));
#79924=CARTESIAN_POINT('Ctrl Pts',(2.8953472557523,1.64660250832305,5.0899970578978));
#79925=CARTESIAN_POINT('Ctrl Pts',(3.01461322816947,-3.38994764974585,4.13855346731278));
#79926=CARTESIAN_POINT('Ctrl Pts',(3.13387920058662,-5.31458498815282,-0.61201002730754));
#79927=CARTESIAN_POINT('Ctrl Pts',(3.25314517300379,-2.3605259971177,-4.80075899069673));
#79928=CARTESIAN_POINT('Ctrl Pts',(3.37241114542096,2.76045469022341,-4.58249492886218));
#79929=CARTESIAN_POINT('Ctrl Pts',(3.49167711783813,5.34738611599374,-0.157580443906409));
#79930=CARTESIAN_POINT('Ctrl Pts',(3.61094309025528,3.02551034903617,4.41199014025406));
#79931=CARTESIAN_POINT('Ctrl Pts',(3.73020906267246,-2.07373115154603,4.93143072352554));
#79932=CARTESIAN_POINT('Ctrl Pts',(3.84947503508961,-5.26932362217573,0.923903909833121));
#79933=CARTESIAN_POINT('Ctrl Pts',(3.96874100750679,-3.62776890794389,-3.93175057962476));
#79934=CARTESIAN_POINT('Ctrl Pts',(4.08800697992394,1.34401439322441,-5.17812660917343));
#79935=CARTESIAN_POINT('Ctrl Pts',(4.2072729523411,5.08201592186332,-1.67107272126372));
#79936=CARTESIAN_POINT('Ctrl Pts',(4.32653892475827,4.15481546776415,3.36999678021387));
#79937=CARTESIAN_POINT('Ctrl Pts',(4.44580489717544,-0.586433123165232,
5.31746801230425));
#79938=CARTESIAN_POINT('Ctrl Pts',(4.56507086959259,-4.78934633478894,2.38359634906328));
#79939=CARTESIAN_POINT('Ctrl Pts',(4.68433684200976,-4.5957231402684,-2.73837519120838));
#79940=CARTESIAN_POINT('Ctrl Pts',(4.80360281442692,-0.183306255264012,
-5.34656606492479));
#79941=CARTESIAN_POINT('Ctrl Pts',(4.9228687868441,4.39738257509714,-3.04670253849241));
#79942=CARTESIAN_POINT('Ctrl Pts',(5.04213475926125,4.94135089461829,2.04998078188042));
#79943=CARTESIAN_POINT('Ctrl Pts',(5.16140073167843,0.949245273126337,5.26481749743252));
#79944=CARTESIAN_POINT('Ctrl Pts',(5.28066670409559,-3.91425095366504,3.64664357204764));
#79945=CARTESIAN_POINT('Ctrl Pts',(5.39993267651275,-5.18453307197378,-1.31908555273497));
#79946=CARTESIAN_POINT('Ctrl Pts',(5.51919864892993,-1.69550425170618,-5.07391714578299));
#79947=CARTESIAN_POINT('Ctrl Pts',(5.63846462134707,3.34996790097437,-4.17098129128691));
#79948=CARTESIAN_POINT('Ctrl Pts',(5.75773059376426,5.32022794609337,0.560842644091171));
#79949=CARTESIAN_POINT('Ctrl Pts',(5.8769965661814,2.40661152479762,4.77782281363966));
#79950=CARTESIAN_POINT('Ctrl Pts',(5.99626253859857,-2.71623230345395,4.6088449684815));
#79951=CARTESIAN_POINT('Ctrl Pts',(6.11552851101574,-5.34562224992299,0.209027823392774));
#79952=CARTESIAN_POINT('Ctrl Pts',(6.23479448343291,-3.06782420195421,-4.38267321799473));
#79953=CARTESIAN_POINT('Ctrl Pts',(6.35406045585007,2.02618295863798,-4.95115668182184));
#79954=CARTESIAN_POINT('Ctrl Pts',(6.47332642826723,5.26018950109706,-0.974564663002068));
#79955=CARTESIAN_POINT('Ctrl Pts',(6.59259240068441,3.66543382254001,3.89666071943709));
#79956=CARTESIAN_POINT('Ctrl Pts',(6.71185837310155,-1.29412617765311,5.19081952163018));
#79957=CARTESIAN_POINT('Ctrl Pts',(6.83112434551873,-5.06570091712964,1.71989653410197));
#79958=CARTESIAN_POINT('Ctrl Pts',(6.95039031793588,-4.18705056366974,-3.32986147566189));
#79959=CARTESIAN_POINT('Ctrl Pts',(7.06965629035308,0.535239182461503,-5.32286472563243));
#79960=CARTESIAN_POINT('Ctrl Pts',(7.18892226277021,4.76618869399877,-2.42957099155845));
#79961=CARTESIAN_POINT('Ctrl Pts',(7.3081882351874,4.62186010975348,2.69402653953035));
#79962=CARTESIAN_POINT('Ctrl Pts',(7.42745420760454,0.234744552882073,5.34455469283609));
#79963=CARTESIAN_POINT('Ctrl Pts',(7.54672018002173,-4.36786240944341,3.08887485049092));
#79964=CARTESIAN_POINT('Ctrl Pts',(7.66598615243887,-4.9608478581489,-2.0023382326979));
#79965=CARTESIAN_POINT('Ctrl Pts',(7.78525212485605,-0.999861493359396,
-5.25543974029968));
#79966=CARTESIAN_POINT('Ctrl Pts',(7.90451809727322,3.87898028412496,-3.68413922445854));
#79967=CARTESIAN_POINT('Ctrl Pts',(8.02378406969037,5.19698581262198,1.26913684574598));
#79968=CARTESIAN_POINT('Ctrl Pts',(8.14305004210754,1.74424900381116,5.05736742609511));
#79969=CARTESIAN_POINT('Ctrl Pts',(8.2623160145247,-3.30967796970602,4.2030229129362));
#79970=CARTESIAN_POINT('Ctrl Pts',(8.38158198694187,-5.32537828988446,-0.509623330952893));
#79971=CARTESIAN_POINT('Ctrl Pts',(8.50084795935902,-2.4524742178731,-4.75444424517648));
#79972=CARTESIAN_POINT('Ctrl Pts',(8.6201139317762,2.67175841346331,-4.63476826280582));
#79973=CARTESIAN_POINT('Ctrl Pts',(8.73937990419336,5.34336341837622,-0.260455848433275));
#79974=CARTESIAN_POINT('Ctrl Pts',(8.85864587661052,3.10985399681577,4.35295049228831));
#79975=CARTESIAN_POINT('Ctrl Pts',(8.97791184902769,-1.97844715602509,4.97042419926512));
#79976=CARTESIAN_POINT('Ctrl Pts',(9.09717782144485,-5.25056832498928,1.02513517861963));
#79977=CARTESIAN_POINT('Ctrl Pts',(9.21644379386203,-3.70275934480493,-3.86121005700076));
#79978=CARTESIAN_POINT('Ctrl Pts',(9.33570976627918,1.24411813547422,-5.20303180220995));
#79979=CARTESIAN_POINT('Ctrl Pts',(9.45497573869635,5.04891686558556,-1.76856109711541));
#79980=CARTESIAN_POINT('Ctrl Pts',(9.57424171111352,4.21889796935353,3.28941785032073));
#79981=CARTESIAN_POINT('Ctrl Pts',(9.69350768353068,-0.483995682528848,
5.32776858066465));
#79982=CARTESIAN_POINT('Ctrl Pts',(9.81277365594783,-4.7425897390368,2.47532067357079));
#79983=CARTESIAN_POINT('Ctrl Pts',(9.932039628365,-4.64756912883677,-2.64942844072216));
#79984=CARTESIAN_POINT('Ctrl Pts',(10.0513056007822,-0.286161114873556,
-5.34204845411932));
#79985=CARTESIAN_POINT('Ctrl Pts',(10.1705715731993,4.33793781171498,-3.13076115529714));
#79986=CARTESIAN_POINT('Ctrl Pts',(10.2898375456165,4.97988548349452,1.95451028165742));
#79987=CARTESIAN_POINT('Ctrl Pts',(10.4091035180337,1.05038513373988,5.24557536793082));
#79988=CARTESIAN_POINT('Ctrl Pts',(10.5283694904508,-3.84335044941505,3.72129375255503));
#79989=CARTESIAN_POINT('Ctrl Pts',(10.647635462868,-5.20895735043977,-1.21907062597848));
#79990=CARTESIAN_POINT('Ctrl Pts',(10.7669014352852,-1.79283225123103,-5.04034943121707));
#79991=CARTESIAN_POINT('Ctrl Pts',(10.8861674077023,3.26908158649335,-4.23467536544114));
#79992=CARTESIAN_POINT('Ctrl Pts',(11.0054333801195,5.3300355426419,0.458356830425908));
#79993=CARTESIAN_POINT('Ctrl Pts',(11.1246993525366,2.49810982979476,4.73062544999149));
#79994=CARTESIAN_POINT('Ctrl Pts',(11.2439653249538,-2.62703713820798,4.66026241152792));
#79995=CARTESIAN_POINT('Ctrl Pts',(11.363231297371,-5.34060983050459,0.311859757169513));
#79996=CARTESIAN_POINT('Ctrl Pts',(11.4824972697881,-3.15159584196975,-4.32282471524157));
#79997=CARTESIAN_POINT('Ctrl Pts',(11.6017632422053,1.93052816369304,-4.98923149182437));
#79998=CARTESIAN_POINT('Ctrl Pts',(11.7210292146225,5.24046098470274,-1.07561077422649));
#79999=CARTESIAN_POINT('Ctrl Pts',(11.8402951870396,3.73974201866875,3.8254018747875));
#80000=CARTESIAN_POINT('Ctrl Pts',(11.9595611594568,-1.1939948970662,5.21476232014501));
#80001=CARTESIAN_POINT('Ctrl Pts',(12.078827131874,-5.0316653213112,1.81706190432193));
#80002=CARTESIAN_POINT('Ctrl Pts',(12.1980931042911,-4.2503547359791,-3.24866964897392));
#80003=CARTESIAN_POINT('Ctrl Pts',(12.3173590767083,0.432707368140066,-5.33217912333988));
#80004=CARTESIAN_POINT('Ctrl Pts',(12.4366250491255,4.71855165499341,-2.52084115901474));
#80005=CARTESIAN_POINT('Ctrl Pts',(12.5558910215426,4.67284781705142,2.6045850242413));
#80006=CARTESIAN_POINT('Ctrl Pts',(12.6751569939598,0.337551180441248,5.33904758083378));
#80007=CARTESIAN_POINT('Ctrl Pts',(12.7944229663769,-4.30761155271047,3.17235757454594));
#80008=CARTESIAN_POINT('Ctrl Pts',(12.9136889387941,-4.99846200791051,-1.90650135727714));
#80009=CARTESIAN_POINT('Ctrl Pts',(13.0329549112113,-1.10081151614861,-5.23522529369453));
#80010=CARTESIAN_POINT('Ctrl Pts',(13.1522208836285,3.80736474859714,-3.75810371609987));
#80011=CARTESIAN_POINT('Ctrl Pts',(13.2714868560456,5.22044657695045,1.16889152919789));
#80012=CARTESIAN_POINT('Ctrl Pts',(13.3907528284628,1.84124949551275,5.02286473689053));
#80013=CARTESIAN_POINT('Ctrl Pts',(13.5100188008799,-3.22818251026418,4.26593571801641));
#80014=CARTESIAN_POINT('Ctrl Pts',(13.6292847732971,-5.33419927313827,-0.407047889412836));
#80015=CARTESIAN_POINT('Ctrl Pts',(13.7485507457143,-2.54351413503901,-4.70636863353064));
#80016=CARTESIAN_POINT('Ctrl Pts',(13.8678167181314,2.58207261855057,-4.68532505407631));
#80017=CARTESIAN_POINT('Ctrl Pts',(13.9870826905486,5.33736174127025,-0.363234789975878));
#80018=CARTESIAN_POINT('Ctrl Pts',(14.1063486629658,3.19304587242686,4.29229867628082));
#80019=CARTESIAN_POINT('Ctrl Pts',(14.2256146353829,-1.88243041858965,5.00757681808199));
#80020=CARTESIAN_POINT('Ctrl Pts',(14.3448806078001,-5.22986841610334,1.12598677615193));
#80021=CARTESIAN_POINT('Ctrl Pts',(14.4641465802173,-3.77637841980645,-3.7892394883729));
#80022=CARTESIAN_POINT('Ctrl Pts',(14.5834125526344,1.14376110347399,-5.22600998927515));
#80023=CARTESIAN_POINT('Ctrl Pts',(14.7026785250516,5.01394788167348,-1.86539446490182));
#80024=CARTESIAN_POINT('Ctrl Pts',(14.8219444974688,4.28141795087999,3.20762064460667));
#80025=CARTESIAN_POINT('Ctrl Pts',(14.9412104698859,-0.381378988217642,
5.33609594527402));
#80026=CARTESIAN_POINT('Ctrl Pts',(15.0604764423031,-4.69407666761928,2.56612823302666));
#80027=CARTESIAN_POINT('Ctrl Pts',(15.1797424147203,-4.69769383377592,-2.55950044225979));
#80028=CARTESIAN_POINT('Ctrl Pts',(15.2990083871374,-0.388909991241378,
-5.33555235083833));
#80029=CARTESIAN_POINT('Ctrl Pts',(15.4182743595546,4.27688644041953,-3.21366025671349));
#80030=CARTESIAN_POINT('Ctrl Pts',(15.5375403319717,5.01657571134664,1.85831590483193));
#80031=CARTESIAN_POINT('Ctrl Pts',(15.6568063043889,1.15113597147179,5.22439047593186));
#80032=CARTESIAN_POINT('Ctrl Pts',(15.7760722768061,-3.77102651368367,3.79456570676));
#80033=CARTESIAN_POINT('Ctrl Pts',(15.8953382492232,-5.23145242833573,-1.11860420162119));
#80034=CARTESIAN_POINT('Ctrl Pts',(16.0146042216404,-1.88949625357401,-5.00491496207014));
#80035=CARTESIAN_POINT('Ctrl Pts',(16.1338701940576,3.18698452797358,-4.2968010761823));
#80036=CARTESIAN_POINT('Ctrl Pts',(16.2531361664747,5.33786909584254,0.355701258745961));
#80037=CARTESIAN_POINT('Ctrl Pts',(16.3724021388919,2.58868292949964,4.68167604179753));
#80038=CARTESIAN_POINT('Ctrl Pts',(16.4916681113091,-2.53686901787644,4.70995386983385));
#80039=CARTESIAN_POINT('Ctrl Pts',(16.6109340837262,-5.33361945142245,0.414576189900464));
#80040=CARTESIAN_POINT('Ctrl Pts',(16.7302000561434,-3.23420025021777,-4.26137520189376));
#80041=CARTESIAN_POINT('Ctrl Pts',(16.8494660285605,1.83415837421399,-5.02545847939519));
#80042=CARTESIAN_POINT('Ctrl Pts',(16.9687320009777,5.21879159998521,-1.17625851994709));
#80043=CARTESIAN_POINT('Ctrl Pts',(17.0879979733949,3.81266515595566,3.75272624612899));
#80044=CARTESIAN_POINT('Ctrl Pts',(17.2072639458121,-1.09342140597902,5.23677376814878));
#80045=CARTESIAN_POINT('Ctrl Pts',(17.3265299182292,-4.99576618717741,1.91355430361389));
#80046=CARTESIAN_POINT('Ctrl Pts',(17.4457958906464,-4.31208473783005,-3.16627463805604));
#80047=CARTESIAN_POINT('Ctrl Pts',(17.5650618630635,0.330015295393627,-5.33951868379825));
#80048=CARTESIAN_POINT('Ctrl Pts',(17.6843278354807,4.66916704311892,-2.61117770235508));
#80049=CARTESIAN_POINT('Ctrl Pts',(17.8035938078979,4.72210487845107,2.51417886927967));
#80050=CARTESIAN_POINT('Ctrl Pts',(17.922859780315,0.440232791824194,5.33156308776582));
#80051=CARTESIAN_POINT('Ctrl Pts',(18.0421257527322,-4.24576531976245,3.25466537747382));
#80052=CARTESIAN_POINT('Ctrl Pts',(18.1613917251494,-5.03422491660662,-1.80995838594174));
#80053=CARTESIAN_POINT('Ctrl Pts',(18.2806576975665,-1.20135384003343,-5.21307191786773));
#80054=CARTESIAN_POINT('Ctrl Pts',(18.3999236699837,3.73433910932905,-3.83067634842202));
#80055=CARTESIAN_POINT('Ctrl Pts',(18.5191896424009,5.24197388553433,1.06821329948656));
#80056=CARTESIAN_POINT('Ctrl Pts',(18.638455614818,1.9375680581184,4.98650176877373));
#80057=CARTESIAN_POINT('Ctrl Pts',(18.7577215872352,-3.14549145425294,4.32726858203256));
#80058=CARTESIAN_POINT('Ctrl Pts',(18.8769875596524,-5.34104467095598,-0.304321692747175));
#80059=CARTESIAN_POINT('Ctrl Pts',(18.9962535320695,-2.63361203087714,-4.65654996114543));
#80060=CARTESIAN_POINT('Ctrl Pts',(19.1155195044867,2.49143052170795,-4.73414657835247));
#80061=CARTESIAN_POINT('Ctrl Pts',(19.2347854769038,5.32938330746976,-0.465879203105705));
#80062=CARTESIAN_POINT('Ctrl Pts',(19.354051449321,3.27505516474859,4.23005715536775));
#80063=CARTESIAN_POINT('Ctrl Pts',(19.4733174217382,-1.78571650020385,5.04287482005294));
#80064=CARTESIAN_POINT('Ctrl Pts',(19.5925833941553,-5.20723156198039,1.22642135081669));
#80065=CARTESIAN_POINT('Ctrl Pts',(19.7118493665725,-3.84859886723042,-3.71586552891477));
#80066=CARTESIAN_POINT('Ctrl Pts',(19.8311153389897,1.04298046566866,-5.24705266011862));
#80067=CARTESIAN_POINT('Ctrl Pts',(19.9503813114068,4.97712192131473,-1.9615369612098));
#80068=CARTESIAN_POINT('Ctrl Pts',(20.069647283824,4.34235225730947,3.12463545765959));
#80069=CARTESIAN_POINT('Ctrl Pts',(20.1889132562412,-0.278621045569882,
5.34244702199188));
#80070=CARTESIAN_POINT('Ctrl Pts',(20.3081792286583,-4.64382508794112,2.65598539574908));
#80071=CARTESIAN_POINT('Ctrl Pts',(20.4274452010755,-4.74607869079302,-2.46862450174681));
#80072=CARTESIAN_POINT('Ctrl Pts',(20.5467111734927,-0.491514830074133,
-5.32708016099266));
#80073=CARTESIAN_POINT('Ctrl Pts',(20.6659771459098,4.21425107232707,-3.29536914005304));
#80074=CARTESIAN_POINT('Ctrl Pts',(20.785243118327,5.05140798950344,1.76143327815877));
#80075=CARTESIAN_POINT('Ctrl Pts',(20.9045090907442,1.25146047202657,5.20127066751764));
#80076=CARTESIAN_POINT('Ctrl Pts',(21.0237750631613,-3.69730593251821,3.86643229750494));
#80077=CARTESIAN_POINT('Ctrl Pts',(21.1430410355785,-5.25200997433651,-1.01772348862257));
#80078=CARTESIAN_POINT('Ctrl Pts',(21.2623070079956,-1.98546045804875,-4.96762686192806));
#80079=CARTESIAN_POINT('Ctrl Pts',(21.3815729804128,3.10370713105701,-4.35733541449928));
#80080=CARTESIAN_POINT('Ctrl Pts',(21.50083895283,5.34372570444373,0.252913948788086));
#80081=CARTESIAN_POINT('Ctrl Pts',(21.6201049252471,2.67829727906562,4.63099271806533));
#80082=CARTESIAN_POINT('Ctrl Pts',(21.7393708976643,-2.44576133731702,4.75790093956452));
#80083=CARTESIAN_POINT('Ctrl Pts',(21.8586368700814,-5.32465370164826,0.517139079308235));
#80084=CARTESIAN_POINT('Ctrl Pts',(21.9779028424986,-3.31560683315326,-4.19834743652449));
#80085=CARTESIAN_POINT('Ctrl Pts',(22.0971688149158,1.73710928192197,-5.05982422742967));
#80086=CARTESIAN_POINT('Ctrl Pts',(22.2164347873329,5.19518937246391,-1.27647062404992));
#80087=CARTESIAN_POINT('Ctrl Pts',(22.3357007597501,3.88417622643207,3.67866074976264));
#80088=CARTESIAN_POINT('Ctrl Pts',(22.4549667321673,-0.992442953004545,
5.25684571343457));
#80089=CARTESIAN_POINT('Ctrl Pts',(22.5742327045844,-4.95801681040808,2.00933799484685));
#80090=CARTESIAN_POINT('Ctrl Pts',(22.6934986770016,-4.37221770676746,-3.08270695890047));
#80091=CARTESIAN_POINT('Ctrl Pts',(22.8127646494188,0.227200997477541,-5.34488068871223));
#80092=CARTESIAN_POINT('Ctrl Pts',(22.9320306218359,4.61805314856548,-2.70054716434442));
#80093=CARTESIAN_POINT('Ctrl Pts',(23.0512965942531,4.76961305100215,2.42284155766206));
#80094=CARTESIAN_POINT('Ctrl Pts',(23.1705625666702,0.542751357650036,5.32210398560502));
#80095=CARTESIAN_POINT('Ctrl Pts',(23.2898285390875,-4.18234661610206,3.33576777558089));
#80096=CARTESIAN_POINT('Ctrl Pts',(23.4090945115045,-5.06812333901019,-1.71274507455268));
#80097=CARTESIAN_POINT('Ctrl Pts',(23.5283604839218,-1.30145122794406,-5.1889878175909));
#80098=CARTESIAN_POINT('Ctrl Pts',(23.6476264563389,3.65993041225227,-3.90183024326985));
#80099=CARTESIAN_POINT('Ctrl Pts',(23.7668924287561,5.26155976547379,0.967139444016044));
#80100=CARTESIAN_POINT('Ctrl Pts',(23.8861584011732,2.03316901887958,4.94829198921123));
#80101=CARTESIAN_POINT('Ctrl Pts',(24.0054243735904,-3.06163542730824,4.38699878961408));
#80102=CARTESIAN_POINT('Ctrl Pts',(24.1246903460076,-5.34591194806159,-0.201482786849391));
#80103=CARTESIAN_POINT('Ctrl Pts',(24.2439563184247,-2.72273453653836,-4.60500667897073));
#80104=CARTESIAN_POINT('Ctrl Pts',(24.3632222908419,2.39986569333583,-4.78121475399025));
#80105=CARTESIAN_POINT('Ctrl Pts',(24.4824882632591,5.31943107188467,-0.568351072218813));
#80106=CARTESIAN_POINT('Ctrl Pts',(24.6017542356763,3.35585150064429,4.16624898145168));
#80107=CARTESIAN_POINT('Ctrl Pts',(24.7210202080934,-1.6883412200409,5.0763051321345));
#80108=CARTESIAN_POINT('Ctrl Pts',(24.8402861805106,-5.1826661464542,1.32640170545049));
#80109=CARTESIAN_POINT('Ctrl Pts',(24.9595521529277,-3.9193939393577,-3.64111535356268));
#80110=CARTESIAN_POINT('Ctrl Pts',(25.0788181253449,0.941813547390232,-5.2661520213317));
#80111=CARTESIAN_POINT('Ctrl Pts',(25.1980840977621,4.93845262345068,-2.05695297849937));
#80112=CARTESIAN_POINT('Ctrl Pts',(25.3173500701792,4.40167832088221,3.04049302405052));
#80113=CARTESIAN_POINT('Ctrl Pts',(25.4366160425964,-0.175759912236459,
5.34681945861972));
#80114=CARTESIAN_POINT('Ctrl Pts',(25.5558820150136,-4.59185361128473,2.74485888204762));
#80115=CARTESIAN_POINT('Ctrl Pts',(25.6751479874307,-4.79270577996915,-2.37683427619063));
#80116=CARTESIAN_POINT('Ctrl Pts',(25.7944139598479,-0.593937630424711,
-5.31663502236041));
#80117=CARTESIAN_POINT('Ctrl Pts',(25.9136799322651,4.15005490520629,-3.37585754343952));
#80118=CARTESIAN_POINT('Ctrl Pts',(26.0329459046822,5.08436941740803,1.66389828329445));
#80119=CARTESIAN_POINT('Ctrl Pts',(26.1522118770994,1.35132147900805,5.17622450538955));
#80120=CARTESIAN_POINT('Ctrl Pts',(26.2714778495166,-3.62221600923054,3.93686690812609));
#80121=CARTESIAN_POINT('Ctrl Pts',(26.3907438219337,-5.27062237470552,-0.916465849378926));
#80122=CARTESIAN_POINT('Ctrl Pts',(26.5100097943509,-2.08068932314761,-4.92849894089096));
#80123=CARTESIAN_POINT('Ctrl Pts',(26.629275766768,3.01928023853817,-4.41625596076554));
#80124=CARTESIAN_POINT('Ctrl Pts',(26.7485417391852,5.34760319937945,0.1500329690799));
#80125=CARTESIAN_POINT('Ctrl Pts',(26.8678077116024,2.76691968873083,4.57859424997864));
#80126=CARTESIAN_POINT('Ctrl Pts',(26.9870736840195,-2.35374783936478,4.80408586294104));
#80127=CARTESIAN_POINT('Ctrl Pts',(27.1063396564367,-5.31371590175628,0.619510439982084));
#80128=CARTESIAN_POINT('Ctrl Pts',(27.2256056288538,-3.39578544086029,-4.13376476223128));
#80129=CARTESIAN_POINT('Ctrl Pts',(27.344871601271,1.63941683012594,-5.09231600815622));
#80130=CARTESIAN_POINT('Ctrl Pts',(27.4641375736882,5.16966304351028,-1.37620997176607));
#80131=CARTESIAN_POINT('Ctrl Pts',(27.5834035461054,3.95424874510512,3.60323281674365));
#80132=CARTESIAN_POINT('Ctrl Pts',(27.7026695185225,-0.891096936738138,
5.27497072211403));
#80133=CARTESIAN_POINT('Ctrl Pts',(27.8219354909397,-4.91843117194308,2.10437750336837));
#80134=CARTESIAN_POINT('Ctrl Pts',(27.9412014633568,-4.43073137181643,-2.99799756181113));
#80135=CARTESIAN_POINT('Ctrl Pts',(28.060467435774,0.124302552914632,-5.34826315219841));
#80136=CARTESIAN_POINT('Ctrl Pts',(28.1797334081912,4.56522890198429,-2.78891644591795));
#80137=CARTESIAN_POINT('Ctrl Pts',(28.2989993806083,4.81535473947628,2.33060691727008));
#80138=CARTESIAN_POINT('Ctrl Pts',(28.4182653530255,0.645068908923938,5.31067377764479));
#80139=CARTESIAN_POINT('Ctrl Pts',(28.5375313254427,-4.11737892961589,3.41563473160984));
#80140=CARTESIAN_POINT('Ctrl Pts',(28.6567972978598,-5.10014472042894,-1.61489742723945));
#80141=CARTESIAN_POINT('Ctrl Pts',(28.7760632702771,-1.4010666075983,-5.1629819127029));
#80142=CARTESIAN_POINT('Ctrl Pts',(28.8953292426941,3.58416621553077,-3.97153904793497));
#80143=CARTESIAN_POINT('Ctrl Pts',(29.0145952151114,5.27919696290035,0.865707396715219));
#80144=CARTESIAN_POINT('Ctrl Pts',(29.1338611875285,2.12801697082046,4.90824954965865));
#80145=CARTESIAN_POINT('Ctrl Pts',(29.2531271599457,-2.97664548652733,4.44510421895379));
#80146=CARTESIAN_POINT('Ctrl Pts',(29.3723931323628,-5.34879930179978,-0.0985692593562008));
#80147=CARTESIAN_POINT('Ctrl Pts',(29.49165910478,-2.81084864442134,-4.55175787668666));
#80148=CARTESIAN_POINT('Ctrl Pts',(29.6109250771972,2.30741204557965,-4.82651214871964));
#80149=CARTESIAN_POINT('Ctrl Pts',(29.7301910496143,5.30750872044597,-0.670612445614996));
#80150=CARTESIAN_POINT('Ctrl Pts',(29.8494570220315,3.43540495621067,4.10089778666421));
#80151=CARTESIAN_POINT('Ctrl Pts',(29.9687229944486,-1.59034064221755,5.10785537300494));
#80152=CARTESIAN_POINT('Ctrl Pts',(30.0879889668658,-5.15618126762428,1.42589081111571));
#80153=CARTESIAN_POINT('Ctrl Pts',(30.207254939283,-3.9887374163744,-3.56501664695121));
#80154=CARTESIAN_POINT('Ctrl Pts',(30.3265209117001,0.840297817034937,-5.28330099923434));
#80155=CARTESIAN_POINT('Ctrl Pts',(30.4457868841173,4.89795430972499,-2.15160717829025));
#80156=CARTESIAN_POINT('Ctrl Pts',(30.5650528565345,4.45937416947051,2.95522450695096));
#80157=CARTESIAN_POINT('Ctrl Pts',(30.6843188289516,-0.0728336840866598,
5.34921163577276));
#80158=CARTESIAN_POINT('Ctrl Pts',(30.8035848013688,-4.53818148591717,2.83271577654773));
#80159=CARTESIAN_POINT('Ctrl Pts',(30.922850773786,-4.83755783239591,-2.28416376121532));
#80160=CARTESIAN_POINT('Ctrl Pts',(31.0421167462031,-0.696140458765788,
-5.30422080342567));
#80161=CARTESIAN_POINT('Ctrl Pts',(31.1613827186203,4.08432171488679,-3.45509565701559));
#80162=CARTESIAN_POINT('Ctrl Pts',(31.2806486910375,5.11544778739555,1.56574704350808));
#80163=CARTESIAN_POINT('Ctrl Pts',(31.3999146634546,1.45068200768019,5.14926126569795));
#80164=CARTESIAN_POINT('Ctrl Pts',(31.5191806358718,-3.54578455428506,4.00584345231029));
#80165=CARTESIAN_POINT('Ctrl Pts',(31.638446608289,-5.28728273611438,-0.814868785885891));
#80166=CARTESIAN_POINT('Ctrl Pts',(31.7577125807061,-2.17514757970455,-4.88754569045954));
#80167=CARTESIAN_POINT('Ctrl Pts',(31.8769785531233,2.9337351189414,-4.47354089304141));
#80168=CARTESIAN_POINT('Ctrl Pts',(31.9962445255404,5.34950014457238,0.047096422840884));
#80169=CARTESIAN_POINT('Ctrl Pts',(32.1155104979576,2.85451733611025,4.52450004394633));
#80170=CARTESIAN_POINT('Ctrl Pts',(32.2347764703748,-2.26086260233548,4.84849153481623));
#80171=CARTESIAN_POINT('Ctrl Pts',(32.3540424427919,-5.30081010269343,0.721652357446135));
#80172=CARTESIAN_POINT('Ctrl Pts',(32.4733084152091,-3.47470637821841,-4.06765109799164));
#80173=CARTESIAN_POINT('Ctrl Pts',(32.5925743876263,1.54111720041119,-5.12292178784925));
#80174=CARTESIAN_POINT('Ctrl Pts',(32.7118403600434,5.14222206711005,-1.47543962341761));
#80175=CARTESIAN_POINT('Ctrl Pts',(32.8311063324606,4.02285675976709,3.52647038272272));
#80176=CARTESIAN_POINT('Ctrl Pts',(32.9503723048777,-0.789420891907063,
5.29114208137));
#80177=CARTESIAN_POINT('Ctrl Pts',(33.0696382772949,-4.87702393280405,2.19863763014299));
#80178=CARTESIAN_POINT('Ctrl Pts',(33.1889042497121,-4.487604061731,-2.91217781994159));
#80179=CARTESIAN_POINT('Ctrl Pts',(33.3081702221293,0.0213580713928514,
-5.34966482152014));
#80180=CARTESIAN_POINT('Ctrl Pts',(33.4274361945464,4.51071386747616,-2.87625281843973));
#80181=CARTESIAN_POINT('Ctrl Pts',(33.5467021669636,4.85931300288409,2.23750910832247));
#80182=CARTESIAN_POINT('Ctrl Pts',(33.6659681393807,0.747147551098779,5.29727669720119));
#80183=CARTESIAN_POINT('Ctrl Pts',(33.785234111798,-4.05088632187509,3.49423666586414));
#80184=CARTESIAN_POINT('Ctrl Pts',(33.904500084215,-5.13027720135584,-1.51645168306597));
#80185=CARTESIAN_POINT('Ctrl Pts',(34.0237660566323,-1.50016308523093,-5.13506383480611));
#80186=CARTESIAN_POINT('Ctrl Pts',(34.1430320290494,3.50707457935405,-4.03977694491552));
#80187=CARTESIAN_POINT('Ctrl Pts',(34.2622980014666,5.29487894566462,0.763954724174054));
#80188=CARTESIAN_POINT('Ctrl Pts',(34.3815639738838,2.22207678584961,4.86638928031932));
#80189=CARTESIAN_POINT('Ctrl Pts',(34.5008299463009,-2.89055310896428,4.5015633500008));
#80190=CARTESIAN_POINT('Ctrl Pts',(34.6200959187181,-5.34970566280806,0.00438077445810644));
#80191=CARTESIAN_POINT('Ctrl Pts',(34.7393618911352,-2.89792172038924,-4.49682327563297));
#80192=CARTESIAN_POINT('Ctrl Pts',(34.8586278635524,2.21410381975605,-4.8700219861014));
#80193=CARTESIAN_POINT('Ctrl Pts',(34.9778938359695,5.29362066876786,-0.772625449552068));
#80194=CARTESIAN_POINT('Ctrl Pts',(35.0971598083868,3.51368606780953,4.03402777461097));
#80195=CARTESIAN_POINT('Ctrl Pts',(35.2164257808038,-1.49175106234197,5.13751385765428));
#80196=CARTESIAN_POINT('Ctrl Pts',(35.3356917532211,-5.12778673466809,1.52485182080563));
#80197=CARTESIAN_POINT('Ctrl Pts',(35.4549577256382,-4.05660361573838,-3.48759759314308));
#80198=CARTESIAN_POINT('Ctrl Pts',(35.5742236980554,0.738470871532858,-5.29849324252636));
#80199=CARTESIAN_POINT('Ctrl Pts',(35.6934896704726,4.85564198041892,-2.24546450419021));
#80200=CARTESIAN_POINT('Ctrl Pts',(35.8127556428897,4.5154184323632,2.86886148647546));
#80201=CARTESIAN_POINT('Ctrl Pts',(35.9320216153069,0.0301195233717248,
5.34962266769844));
#80202=CARTESIAN_POINT('Ctrl Pts',(36.051287587724,-4.48282859845072,2.91952353996583));
#80203=CARTESIAN_POINT('Ctrl Pts',(36.1705535601412,-4.88061822044823,-2.19064727767925));
#80204=CARTESIAN_POINT('Ctrl Pts',(36.2898195325583,-0.79808549366158,-5.28984210344808));
#80205=CARTESIAN_POINT('Ctrl Pts',(36.4090855049755,4.01707590461207,-3.53305413112963));
#80206=CARTESIAN_POINT('Ctrl Pts',(36.5283514773927,5.14463147875642,1.46701590488028));
#80207=CARTESIAN_POINT('Ctrl Pts',(36.6476174498098,1.54950546845328,5.12039094490375));
#80208=CARTESIAN_POINT('Ctrl Pts',(36.7668834222271,-3.46804027343879,4.07333636419893));
#80209=CARTESIAN_POINT('Ctrl Pts',(36.8861493946441,-5.30198413145758,-0.712969888702118));
#80210=CARTESIAN_POINT('Ctrl Pts',(37.0054153670614,-2.26880168119574,-4.84478234871799));
#80211=CARTESIAN_POINT('Ctrl Pts',(37.1246813394785,2.84710618461792,-4.5291688611629));
#80212=CARTESIAN_POINT('Ctrl Pts',(37.2439473118957,5.34941065311671,-0.0558578206189876));
#80213=CARTESIAN_POINT('Ctrl Pts',(37.3632132843128,2.9410676247427,4.46873061775304));
#80214=CARTESIAN_POINT('Ctrl Pts',(37.48247925673,-2.16715872819103,4.89110059102707));
#80215=CARTESIAN_POINT('Ctrl Pts',(37.6017452291471,-5.28590556674589,0.823528745687691));
#80216=CARTESIAN_POINT('Ctrl Pts',(37.7210112015644,-3.55240787274374,-4.00003424114442));
#80217=CARTESIAN_POINT('Ctrl Pts',(37.8402771739814,1.44237491738078,-5.15162394203852));
#80218=CARTESIAN_POINT('Ctrl Pts',(37.9595431463987,5.11263327306786,-1.57413477445065));
#80219=CARTESIAN_POINT('Ctrl Pts',(38.0788091188158,4.09043705061455,3.44842457930616));
#80220=CARTESIAN_POINT('Ctrl Pts',(38.198075091233,-0.688330618759455,5.30531057884261));
#80221=CARTESIAN_POINT('Ctrl Pts',(38.3173410636501,-4.83213982762216,2.29216646455193));
#80222=CARTESIAN_POINT('Ctrl Pts',(38.4366070360674,-4.54601128230848,-2.82544487853224));
#80223=CARTESIAN_POINT('Ctrl Pts',(38.5558730084845,-0.0753220462620636,
-5.34870520161382));
#80224=CARTESIAN_POINT('Ctrl Pts',(38.6552613188321,3.68821096221221,-3.36131348540175));
#80225=CARTESIAN_POINT('Ctrl Pts',(38.7347719671102,4.6906167652542,-0.404679689500564));
#80226=CARTESIAN_POINT('Ctrl Pts',(38.7745272912493,4.44656964843245,1.12242207018042));
#80227=CARTESIAN_POINT('Ctrl Pts',(38.7944049533188,4.14471859505469,1.81262843139675));
#80228=CARTESIAN_POINT('Ctrl Pts',(38.546,4.53891924175751,1.98502597383594));
#80229=CARTESIAN_POINT('Ctrl Pts',(38.5261223379305,4.86947909109343,1.22917467492126));
#80230=CARTESIAN_POINT('Ctrl Pts',(38.5062446758609,5.0031082059578,0.393003122839607));
#80231=CARTESIAN_POINT('Ctrl Pts',(38.4863670137914,4.93270479300402,-0.429812242173168));
#80232=CARTESIAN_POINT('Ctrl Pts',(38.4664893517219,4.86230138005024,-1.25262760718594));
#80233=CARTESIAN_POINT('Ctrl Pts',(38.4466116896524,4.58786543927832,-2.06208678512975));
#80234=CARTESIAN_POINT('Ctrl Pts',(38.4267340275828,4.1301428507968,-2.74682029345583));
#80235=CARTESIAN_POINT('Ctrl Pts',(38.3869787034438,3.21469767383359,-4.11628731010823));
#80236=CARTESIAN_POINT('Ctrl Pts',(38.3472233793047,1.56610590603186,-4.98685164828932));
#80237=CARTESIAN_POINT('Ctrl Pts',(38.3074680551656,-0.0741720898843624,
-4.96159290771613));
#80238=CARTESIAN_POINT('Ctrl Pts',(38.2677127310266,-1.71445008580022,-4.93633416714295));
#80239=CARTESIAN_POINT('Ctrl Pts',(38.2279574068875,-3.34641430983077,-4.01525234781577));
#80240=CARTESIAN_POINT('Ctrl Pts',(38.1882020827485,-4.21462008633842,-2.620654273424));
#80241=CARTESIAN_POINT('Ctrl Pts',(38.166064292547,-4.69808130186775,-1.84407100426816));
#80242=CARTESIAN_POINT('Ctrl Pts',(38.1439265023456,-4.94471401759233,-0.920658400937587));
#80243=CARTESIAN_POINT('Ctrl Pts',(38.1217887121441,-4.94678507297176,0.00149831882859774));
#80244=CARTESIAN_POINT('Origin',(-20.5573438024112,0.,0.));
#80245=CARTESIAN_POINT('',(-18.6,-2.5,-3.06161699786838E-16));
#80246=CARTESIAN_POINT('Origin',(-18.6,0.,0.));
#80247=CARTESIAN_POINT('',(-22.5146876048223,-2.5,-3.06161699786838E-16));
#80248=CARTESIAN_POINT('',(-20.5573438024112,-2.5,-3.06161699786838E-16));
#80249=CARTESIAN_POINT('Origin',(-22.5146876048223,0.,0.));
#80250=CARTESIAN_POINT('Origin',(-18.1,0.,0.));
#80251=CARTESIAN_POINT('',(-18.1,-3.75,-4.59242549680257E-16));
#80252=CARTESIAN_POINT('Origin',(10.45,0.,0.));
#80253=CARTESIAN_POINT('Origin',(38.546,0.,0.));
#80254=CARTESIAN_POINT('Origin',(38.75,0.,0.));
#80255=CARTESIAN_POINT('',(39.,-4.5,-5.51091059616309E-16));
#80256=CARTESIAN_POINT('Origin',(39.,0.,0.));
#80257=CARTESIAN_POINT('',(38.75,-4.75,-5.81707229594993E-16));
#80258=CARTESIAN_POINT('Origin',(39.,0.,0.));
#80259=CARTESIAN_POINT('Origin',(-24.173,-3.33066907387547E-15,0.));
#80260=CARTESIAN_POINT('',(-24.173,-3.33066907387547E-15,3.00000000000001));
#80261=CARTESIAN_POINT('',(-24.173,-3.33066907387547E-15,-3.00000000000001));
#80262=CARTESIAN_POINT('Origin',(-24.173,-3.33066907387547E-15,0.));
#82360=UNCERTAINTY_MEASURE_WITH_UNIT(LENGTH_MEASURE(0.01),#82385,
'DISTANCE_ACCURACY_VALUE',
'Maximum model space distance between geometric entities at asserted c
onnectivities');
#82363=UNCERTAINTY_MEASURE_WITH_UNIT(LENGTH_MEASURE(0.01),#82385,
'DISTANCE_ACCURACY_VALUE',
'Maximum model space distance between geometric entities at asserted c
onnectivities');
#82381=(
GEOMETRIC_REPRESENTATION_CONTEXT(3)
GLOBAL_UNCERTAINTY_ASSIGNED_CONTEXT((#82360))
GLOBAL_UNIT_ASSIGNED_CONTEXT((#82385,#82387,#82388))
REPRESENTATION_CONTEXT('','3D')
);
#82384=(
GEOMETRIC_REPRESENTATION_CONTEXT(3)
GLOBAL_UNCERTAINTY_ASSIGNED_CONTEXT((#82363))
GLOBAL_UNIT_ASSIGNED_CONTEXT((#82385,#82387,#82388))
REPRESENTATION_CONTEXT('','3D')
);
#82385=(
LENGTH_UNIT()
NAMED_UNIT(*)
SI_UNIT(.MILLI.,.METRE.)
);
#82387=(
NAMED_UNIT(*)
PLANE_ANGLE_UNIT()
SI_UNIT($,.RADIAN.)
);
#82388=(
NAMED_UNIT(*)
SI_UNIT($,.STERADIAN.)
SOLID_ANGLE_UNIT()
);
#82406=SHAPE_DEFINITION_REPRESENTATION(#82426,#82482);
#82426=PRODUCT_DEFINITION_SHAPE('',$,#82503);
#82482=SHAPE_REPRESENTATION('',(#32982),#82381);
#82485=PRODUCT_DEFINITION_CONTEXT('part definition',#82547,'design');
#82503=PRODUCT_DEFINITION('2026-10-20-12-38-14-832',
'05_AJS100_Adjustment_Screw_M10x0.75',#82523,#82485);
#82523=PRODUCT_DEFINITION_FORMATION('',$,#82566);
#82547=APPLICATION_CONTEXT(
'Core Data for Automotive Mechanical Design Process');
#82548=PRODUCT_CONTEXT('part definition',#82547,'mechanical');
#82566=PRODUCT('2026-10-20-12-38-14-832',
'05_AJS100_Adjustment_Screw_M10x0.75',$,(#82548));
#82632=COLOUR_RGB('Black',0.12,0.14,0.17);
#82633=FILL_AREA_STYLE_COLOUR('',#82632);
#82634=FILL_AREA_STYLE('',(#82633));
#82635=SURFACE_STYLE_FILL_AREA(#82634);
#82636=SURFACE_SIDE_STYLE('',(#82635));
#82637=SURFACE_STYLE_USAGE(.BOTH.,#82636);
#82638=PRESENTATION_STYLE_ASSIGNMENT((#82637));
ENDSEC;
END-ISO-10303-21;
